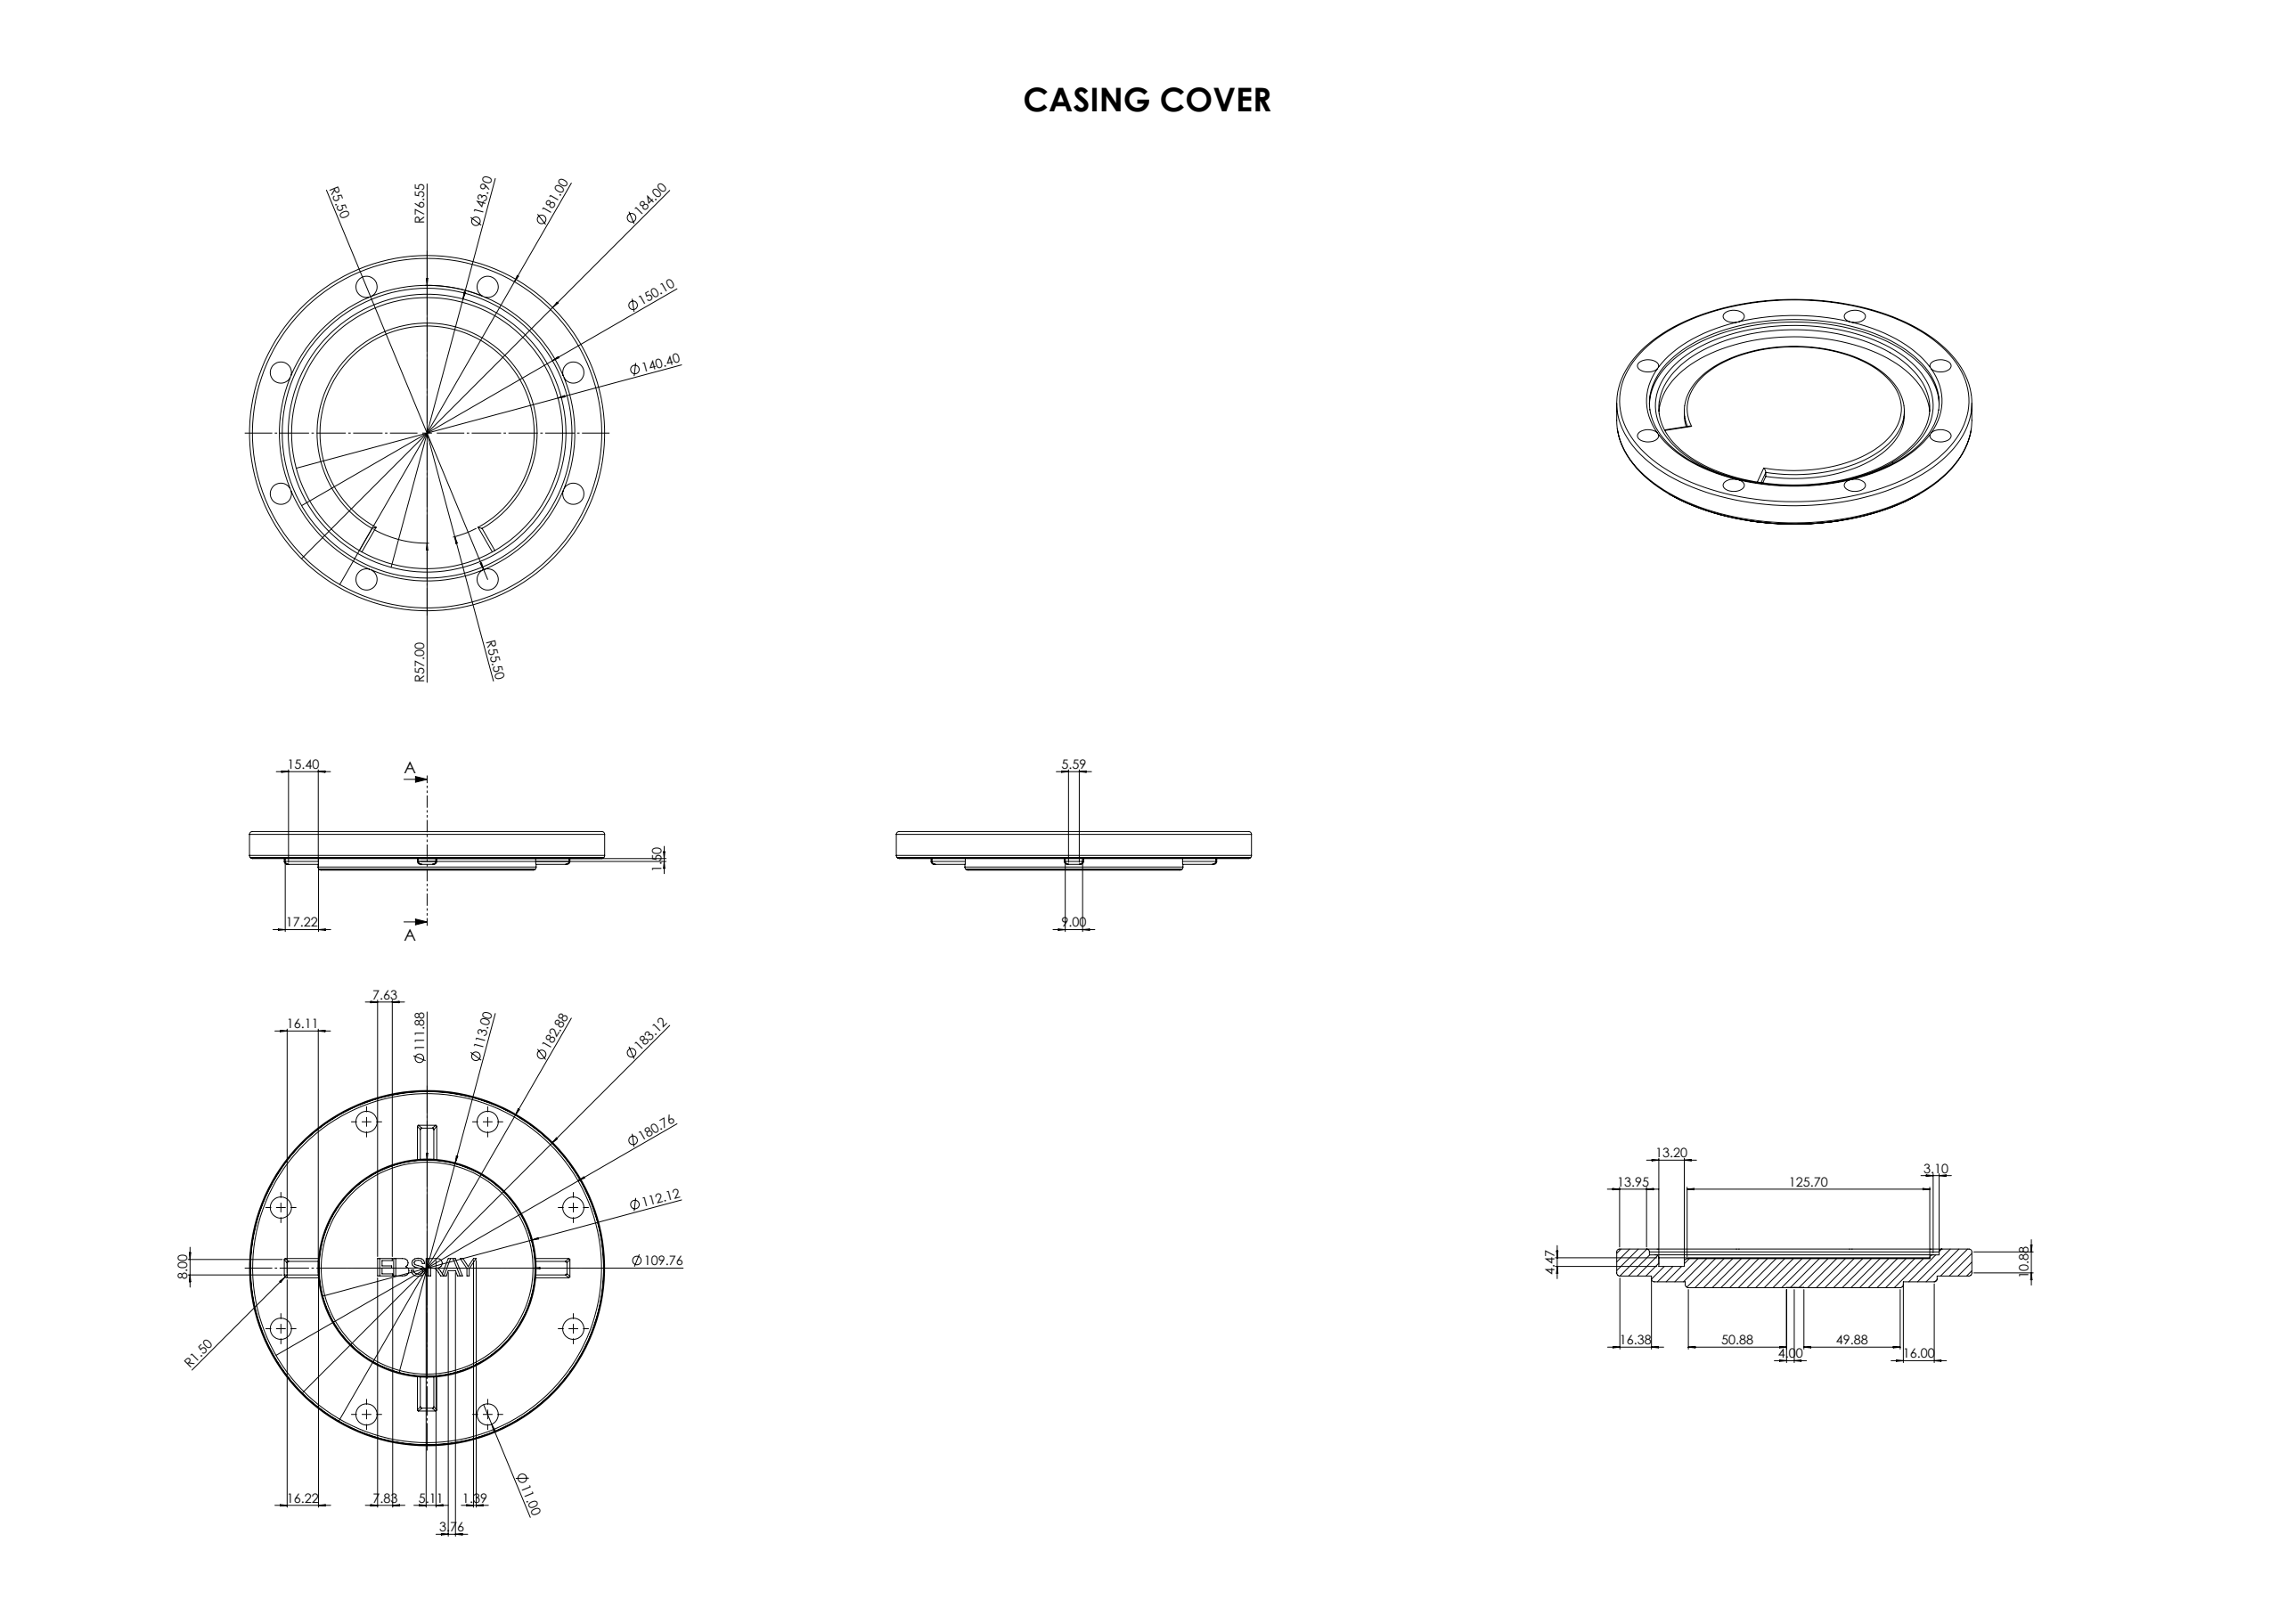
ISO-10303-21;
HEADER;
/* Generated by software containing ST-Developer
 * from STEP Tools, Inc. (www.steptools.com) 
 */

FILE_DESCRIPTION(
/* description */ (''),
/* implementation_level */ '2;1');

FILE_NAME(
/* name */ '02_Casing_Cover.step',
/* time_stamp */ '2026-10-26T04:15:57-07:00',
/* author */ (''),
/* organization */ (''),
/* preprocessor_version */ 'ST-DEVELOPER v20.2',
/* originating_system */ 'Autodesk Translation Framework v15.15.0.0',
/* authorisation */ '');

FILE_SCHEMA (('AUTOMOTIVE_DESIGN { 1 0 10303 214 3 1 1 }'));
ENDSEC;

DATA;
#10=MECHANICAL_DESIGN_GEOMETRIC_PRESENTATION_REPRESENTATION('',(#453),#55737);
#197=ELLIPSE('',#27930,1.60681112727484,1.5);
#198=ELLIPSE('',#27931,1.86380959388014,1.5);
#199=ELLIPSE('',#27932,1.60681112727484,1.5);
#200=ELLIPSE('',#27934,1.62076900489975,1.5);
#201=ELLIPSE('',#27935,1.62076900489975,1.5);
#338=SPHERICAL_SURFACE('',#27885,1.5);
#339=CONICAL_SURFACE('',#27821,91.5,0.785398163397447);
#340=CONICAL_SURFACE('',#27879,56.,0.785398163397451);
#413=SHAPE_REPRESENTATION_RELATIONSHIP('SRR','None',#55822,#433);
#433=ADVANCED_BREP_SHAPE_REPRESENTATION('',(#473),#55718);
#453=STYLED_ITEM('',(#55977),#473);
#473=MANIFOLD_SOLID_BREP('Body1',#27222);
#496=B_SPLINE_SURFACE_WITH_KNOTS('',3,3,((#38586,#38587,#38588,#38589,#38590,
#38591),(#38592,#38593,#38594,#38595,#38596,#38597),(#38598,#38599,#38600,
#38601,#38602,#38603),(#38604,#38605,#38606,#38607,#38608,#38609)),
 .UNSPECIFIED.,.F.,.F.,.F.,(4,4),(4,1,1,4),(0.,1.),(0.,0.571428571428571,
0.857142857142857,1.),.UNSPECIFIED.);
#497=B_SPLINE_SURFACE_WITH_KNOTS('',3,3,((#38729,#38730,#38731,#38732,#38733,
#38734),(#38735,#38736,#38737,#38738,#38739,#38740),(#38741,#38742,#38743,
#38744,#38745,#38746),(#38747,#38748,#38749,#38750,#38751,#38752)),
 .UNSPECIFIED.,.F.,.F.,.F.,(4,4),(4,1,1,4),(0.,1.),(-1.75610615531806,-1.00348923161032,
-0.501744615805159,2.22044604925036E-16),.UNSPECIFIED.);
#498=B_SPLINE_SURFACE_WITH_KNOTS('',3,3,((#38856,#38857,#38858,#38859,#38860,
#38861),(#38862,#38863,#38864,#38865,#38866,#38867),(#38868,#38869,#38870,
#38871,#38872,#38873),(#38874,#38875,#38876,#38877,#38878,#38879)),
 .UNSPECIFIED.,.F.,.F.,.F.,(4,4),(4,1,1,4),(0.,1.),(0.,0.571428571428571,
0.857142857142857,1.),.UNSPECIFIED.);
#499=B_SPLINE_SURFACE_WITH_KNOTS('',3,3,((#38940,#38941,#38942,#38943,#38944,
#38945,#38946),(#38947,#38948,#38949,#38950,#38951,#38952,#38953),(#38954,
#38955,#38956,#38957,#38958,#38959,#38960),(#38961,#38962,#38963,#38964,
#38965,#38966,#38967)),.UNSPECIFIED.,.F.,.F.,.F.,(4,4),(4,1,1,1,4),(0.,
1.),(-1.75610615531806,-1.2543615395129,-0.752616923707738,-0.501744615805159,
4.16333634234434E-16),.UNSPECIFIED.);
#500=B_SPLINE_SURFACE_WITH_KNOTS('',3,3,((#38998,#38999,#39000,#39001,#39002,
#39003),(#39004,#39005,#39006,#39007,#39008,#39009),(#39010,#39011,#39012,
#39013,#39014,#39015),(#39016,#39017,#39018,#39019,#39020,#39021)),
 .UNSPECIFIED.,.F.,.F.,.F.,(4,4),(4,1,1,4),(0.,1.),(0.,0.571428571428571,
0.857142857142857,1.),.UNSPECIFIED.);
#501=B_SPLINE_SURFACE_WITH_KNOTS('',3,3,((#39141,#39142,#39143,#39144,#39145,
#39146),(#39147,#39148,#39149,#39150,#39151,#39152),(#39153,#39154,#39155,
#39156,#39157,#39158),(#39159,#39160,#39161,#39162,#39163,#39164)),
 .UNSPECIFIED.,.F.,.F.,.F.,(4,4),(4,1,1,4),(0.,1.),(-1.75610615531806,-1.00348923161032,
-0.501744615805159,2.77555756156289E-17),.UNSPECIFIED.);
#502=B_SPLINE_SURFACE_WITH_KNOTS('',3,3,((#39202,#39203,#39204,#39205,#39206,
#39207),(#39208,#39209,#39210,#39211,#39212,#39213),(#39214,#39215,#39216,
#39217,#39218,#39219),(#39220,#39221,#39222,#39223,#39224,#39225)),
 .UNSPECIFIED.,.F.,.F.,.F.,(4,4),(4,1,1,4),(0.,1.),(0.,0.571428571428571,
0.857142857142857,1.),.UNSPECIFIED.);
#503=B_SPLINE_SURFACE_WITH_KNOTS('',3,3,((#39345,#39346,#39347,#39348,#39349,
#39350),(#39351,#39352,#39353,#39354,#39355,#39356),(#39357,#39358,#39359,
#39360,#39361,#39362),(#39363,#39364,#39365,#39366,#39367,#39368)),
 .UNSPECIFIED.,.F.,.F.,.F.,(4,4),(4,1,1,4),(0.,1.),(-1.75610615531806,-1.00348923161032,
-0.501744615805159,2.77555756156289E-17),.UNSPECIFIED.);
#504=B_SPLINE_SURFACE_WITH_KNOTS('',3,3,((#39469,#39470,#39471,#39472,#39473,
#39474),(#39475,#39476,#39477,#39478,#39479,#39480),(#39481,#39482,#39483,
#39484,#39485,#39486),(#39487,#39488,#39489,#39490,#39491,#39492)),
 .UNSPECIFIED.,.F.,.F.,.F.,(4,4),(4,1,1,4),(0.,1.),(0.,0.571428571428571,
0.857142857142857,1.),.UNSPECIFIED.);
#505=B_SPLINE_SURFACE_WITH_KNOTS('',3,3,((#39553,#39554,#39555,#39556,#39557,
#39558),(#39559,#39560,#39561,#39562,#39563,#39564),(#39565,#39566,#39567,
#39568,#39569,#39570),(#39571,#39572,#39573,#39574,#39575,#39576)),
 .UNSPECIFIED.,.F.,.F.,.F.,(4,4),(4,1,1,4),(0.,1.),(-1.75610615531806,-1.00348923161032,
-0.501744615805159,1.27116549159798E-31),.UNSPECIFIED.);
#506=B_SPLINE_SURFACE_WITH_KNOTS('',3,3,((#39606,#39607,#39608,#39609,#39610,
#39611),(#39612,#39613,#39614,#39615,#39616,#39617),(#39618,#39619,#39620,
#39621,#39622,#39623),(#39624,#39625,#39626,#39627,#39628,#39629)),
 .UNSPECIFIED.,.F.,.F.,.F.,(4,4),(4,1,1,4),(0.,1.),(0.,0.571428571428571,
0.857142857142857,1.),.UNSPECIFIED.);
#507=B_SPLINE_SURFACE_WITH_KNOTS('',3,3,((#39749,#39750,#39751,#39752,#39753,
#39754,#39755),(#39756,#39757,#39758,#39759,#39760,#39761,#39762),(#39763,
#39764,#39765,#39766,#39767,#39768,#39769),(#39770,#39771,#39772,#39773,
#39774,#39775,#39776)),.UNSPECIFIED.,.F.,.F.,.F.,(4,4),(4,1,1,1,4),(0.,
1.),(-1.75610615531805,-1.25436153951289,-0.752616923707736,-0.501744615805158,
1.11022302462516E-16),.UNSPECIFIED.);
#508=B_SPLINE_SURFACE_WITH_KNOTS('',3,3,((#39880,#39881,#39882,#39883,#39884,
#39885),(#39886,#39887,#39888,#39889,#39890,#39891),(#39892,#39893,#39894,
#39895,#39896,#39897),(#39898,#39899,#39900,#39901,#39902,#39903)),
 .UNSPECIFIED.,.F.,.F.,.F.,(4,4),(4,1,1,4),(0.,1.),(0.,0.571428571428571,
0.857142857142857,1.),.UNSPECIFIED.);
#509=B_SPLINE_SURFACE_WITH_KNOTS('',3,3,((#39964,#39965,#39966,#39967,#39968,
#39969,#39970),(#39971,#39972,#39973,#39974,#39975,#39976,#39977),(#39978,
#39979,#39980,#39981,#39982,#39983,#39984),(#39985,#39986,#39987,#39988,
#39989,#39990,#39991)),.UNSPECIFIED.,.F.,.F.,.F.,(4,4),(4,1,1,1,4),(0.,
1.),(-1.75610615531806,-1.2543615395129,-0.752616923707739,-0.501744615805159,
4.10679309198325E-32),.UNSPECIFIED.);
#510=B_SPLINE_SURFACE_WITH_KNOTS('',2,1,((#40770,#40771),(#40772,#40773),
(#40774,#40775)),.UNSPECIFIED.,.F.,.F.,.F.,(3,3),(2,2),(0.,1.),(0.,0.05),
 .UNSPECIFIED.);
#511=B_SPLINE_SURFACE_WITH_KNOTS('',2,1,((#40783,#40784),(#40785,#40786),
(#40787,#40788)),.UNSPECIFIED.,.F.,.F.,.F.,(3,3),(2,2),(0.,1.),(0.,0.05),
 .UNSPECIFIED.);
#512=B_SPLINE_SURFACE_WITH_KNOTS('',2,1,((#40794,#40795),(#40796,#40797),
(#40798,#40799)),.UNSPECIFIED.,.F.,.F.,.F.,(3,3),(2,2),(0.,1.),(0.,0.05),
 .UNSPECIFIED.);
#513=B_SPLINE_SURFACE_WITH_KNOTS('',2,1,((#40805,#40806),(#40807,#40808),
(#40809,#40810)),.UNSPECIFIED.,.F.,.F.,.F.,(3,3),(2,2),(0.,1.),(0.,0.05),
 .UNSPECIFIED.);
#514=B_SPLINE_SURFACE_WITH_KNOTS('',2,1,((#40816,#40817),(#40818,#40819),
(#40820,#40821)),.UNSPECIFIED.,.F.,.F.,.F.,(3,3),(2,2),(0.,1.),(0.,0.05),
 .UNSPECIFIED.);
#515=B_SPLINE_SURFACE_WITH_KNOTS('',2,1,((#40827,#40828),(#40829,#40830),
(#40831,#40832)),.UNSPECIFIED.,.F.,.F.,.F.,(3,3),(2,2),(0.,1.),(0.,0.05),
 .UNSPECIFIED.);
#516=B_SPLINE_SURFACE_WITH_KNOTS('',2,1,((#40838,#40839),(#40840,#40841),
(#40842,#40843)),.UNSPECIFIED.,.F.,.F.,.F.,(3,3),(2,2),(0.,1.),(0.,0.05),
 .UNSPECIFIED.);
#517=B_SPLINE_SURFACE_WITH_KNOTS('',2,1,((#40849,#40850),(#40851,#40852),
(#40853,#40854)),.UNSPECIFIED.,.F.,.F.,.F.,(3,3),(2,2),(0.,1.),(0.,0.05),
 .UNSPECIFIED.);
#518=B_SPLINE_SURFACE_WITH_KNOTS('',2,1,((#40860,#40861),(#40862,#40863),
(#40864,#40865)),.UNSPECIFIED.,.F.,.F.,.F.,(3,3),(2,2),(0.,1.),(0.,0.05),
 .UNSPECIFIED.);
#519=B_SPLINE_SURFACE_WITH_KNOTS('',2,1,((#40871,#40872),(#40873,#40874),
(#40875,#40876)),.UNSPECIFIED.,.F.,.F.,.F.,(3,3),(2,2),(0.,1.),(0.,0.05),
 .UNSPECIFIED.);
#520=B_SPLINE_SURFACE_WITH_KNOTS('',2,1,((#40888,#40889),(#40890,#40891),
(#40892,#40893)),.UNSPECIFIED.,.F.,.F.,.F.,(3,3),(2,2),(0.,1.),(0.,0.05),
 .UNSPECIFIED.);
#521=B_SPLINE_SURFACE_WITH_KNOTS('',2,1,((#40898,#40899),(#40900,#40901),
(#40902,#40903)),.UNSPECIFIED.,.F.,.F.,.F.,(3,3),(2,2),(0.,1.),(0.,0.05),
 .UNSPECIFIED.);
#522=B_SPLINE_SURFACE_WITH_KNOTS('',2,1,((#40911,#40912),(#40913,#40914),
(#40915,#40916)),.UNSPECIFIED.,.F.,.F.,.F.,(3,3),(2,2),(0.,1.),(0.,0.05),
 .UNSPECIFIED.);
#523=B_SPLINE_SURFACE_WITH_KNOTS('',2,1,((#40922,#40923),(#40924,#40925),
(#40926,#40927)),.UNSPECIFIED.,.F.,.F.,.F.,(3,3),(2,2),(0.,1.),(0.,0.05),
 .UNSPECIFIED.);
#524=B_SPLINE_SURFACE_WITH_KNOTS('',2,1,((#40933,#40934),(#40935,#40936),
(#40937,#40938)),.UNSPECIFIED.,.F.,.F.,.F.,(3,3),(2,2),(0.,1.),(0.,0.05),
 .UNSPECIFIED.);
#525=B_SPLINE_SURFACE_WITH_KNOTS('',2,1,((#40944,#40945),(#40946,#40947),
(#40948,#40949)),.UNSPECIFIED.,.F.,.F.,.F.,(3,3),(2,2),(0.,1.),(0.,0.05),
 .UNSPECIFIED.);
#526=B_SPLINE_SURFACE_WITH_KNOTS('',2,1,((#40955,#40956),(#40957,#40958),
(#40959,#40960)),.UNSPECIFIED.,.F.,.F.,.F.,(3,3),(2,2),(0.,1.),(0.,0.05),
 .UNSPECIFIED.);
#527=B_SPLINE_SURFACE_WITH_KNOTS('',2,1,((#40966,#40967),(#40968,#40969),
(#40970,#40971)),.UNSPECIFIED.,.F.,.F.,.F.,(3,3),(2,2),(0.,1.),(0.,0.05),
 .UNSPECIFIED.);
#528=B_SPLINE_SURFACE_WITH_KNOTS('',2,1,((#40977,#40978),(#40979,#40980),
(#40981,#40982)),.UNSPECIFIED.,.F.,.F.,.F.,(3,3),(2,2),(0.,1.),(0.,0.05),
 .UNSPECIFIED.);
#529=B_SPLINE_SURFACE_WITH_KNOTS('',2,1,((#40988,#40989),(#40990,#40991),
(#40992,#40993)),.UNSPECIFIED.,.F.,.F.,.F.,(3,3),(2,2),(0.,1.),(0.,0.05),
 .UNSPECIFIED.);
#530=B_SPLINE_SURFACE_WITH_KNOTS('',2,1,((#40999,#41000),(#41001,#41002),
(#41003,#41004)),.UNSPECIFIED.,.F.,.F.,.F.,(3,3),(2,2),(0.,1.),(0.,0.05),
 .UNSPECIFIED.);
#531=B_SPLINE_SURFACE_WITH_KNOTS('',2,1,((#41010,#41011),(#41012,#41013),
(#41014,#41015)),.UNSPECIFIED.,.F.,.F.,.F.,(3,3),(2,2),(0.,1.),(0.,0.05),
 .UNSPECIFIED.);
#532=B_SPLINE_SURFACE_WITH_KNOTS('',2,1,((#41021,#41022),(#41023,#41024),
(#41025,#41026)),.UNSPECIFIED.,.F.,.F.,.F.,(3,3),(2,2),(0.,1.),(0.,0.05),
 .UNSPECIFIED.);
#533=B_SPLINE_SURFACE_WITH_KNOTS('',2,1,((#41032,#41033),(#41034,#41035),
(#41036,#41037)),.UNSPECIFIED.,.F.,.F.,.F.,(3,3),(2,2),(0.,1.),(0.,0.05),
 .UNSPECIFIED.);
#534=B_SPLINE_SURFACE_WITH_KNOTS('',2,1,((#41047,#41048),(#41049,#41050),
(#41051,#41052)),.UNSPECIFIED.,.F.,.F.,.F.,(3,3),(2,2),(0.,1.),(0.,0.05),
 .UNSPECIFIED.);
#535=B_SPLINE_SURFACE_WITH_KNOTS('',2,1,((#41058,#41059),(#41060,#41061),
(#41062,#41063)),.UNSPECIFIED.,.F.,.F.,.F.,(3,3),(2,2),(0.,1.),(0.,0.05),
 .UNSPECIFIED.);
#536=B_SPLINE_SURFACE_WITH_KNOTS('',2,1,((#41069,#41070),(#41071,#41072),
(#41073,#41074)),.UNSPECIFIED.,.F.,.F.,.F.,(3,3),(2,2),(0.,1.),(0.,0.05),
 .UNSPECIFIED.);
#537=B_SPLINE_SURFACE_WITH_KNOTS('',2,1,((#41080,#41081),(#41082,#41083),
(#41084,#41085)),.UNSPECIFIED.,.F.,.F.,.F.,(3,3),(2,2),(0.,1.),(0.,0.05),
 .UNSPECIFIED.);
#538=B_SPLINE_SURFACE_WITH_KNOTS('',2,1,((#41091,#41092),(#41093,#41094),
(#41095,#41096)),.UNSPECIFIED.,.F.,.F.,.F.,(3,3),(2,2),(0.,1.),(0.,0.05),
 .UNSPECIFIED.);
#539=B_SPLINE_SURFACE_WITH_KNOTS('',2,1,((#41102,#41103),(#41104,#41105),
(#41106,#41107)),.UNSPECIFIED.,.F.,.F.,.F.,(3,3),(2,2),(0.,1.),(0.,0.05),
 .UNSPECIFIED.);
#540=B_SPLINE_SURFACE_WITH_KNOTS('',2,1,((#41113,#41114),(#41115,#41116),
(#41117,#41118)),.UNSPECIFIED.,.F.,.F.,.F.,(3,3),(2,2),(0.,1.),(0.,0.05),
 .UNSPECIFIED.);
#541=B_SPLINE_SURFACE_WITH_KNOTS('',2,1,((#41124,#41125),(#41126,#41127),
(#41128,#41129)),.UNSPECIFIED.,.F.,.F.,.F.,(3,3),(2,2),(0.,1.),(0.,0.05),
 .UNSPECIFIED.);
#542=B_SPLINE_SURFACE_WITH_KNOTS('',2,1,((#41135,#41136),(#41137,#41138),
(#41139,#41140)),.UNSPECIFIED.,.F.,.F.,.F.,(3,3),(2,2),(0.,1.),(0.,0.05),
 .UNSPECIFIED.);
#543=B_SPLINE_SURFACE_WITH_KNOTS('',2,1,((#41146,#41147),(#41148,#41149),
(#41150,#41151)),.UNSPECIFIED.,.F.,.F.,.F.,(3,3),(2,2),(0.,1.),(0.,0.05),
 .UNSPECIFIED.);
#544=B_SPLINE_SURFACE_WITH_KNOTS('',2,1,((#41157,#41158),(#41159,#41160),
(#41161,#41162)),.UNSPECIFIED.,.F.,.F.,.F.,(3,3),(2,2),(0.,1.),(0.,0.05),
 .UNSPECIFIED.);
#545=B_SPLINE_SURFACE_WITH_KNOTS('',2,1,((#41168,#41169),(#41170,#41171),
(#41172,#41173)),.UNSPECIFIED.,.F.,.F.,.F.,(3,3),(2,2),(0.,1.),(0.,0.05),
 .UNSPECIFIED.);
#546=B_SPLINE_SURFACE_WITH_KNOTS('',2,1,((#41179,#41180),(#41181,#41182),
(#41183,#41184)),.UNSPECIFIED.,.F.,.F.,.F.,(3,3),(2,2),(0.,1.),(0.,0.05),
 .UNSPECIFIED.);
#547=B_SPLINE_SURFACE_WITH_KNOTS('',2,1,((#41190,#41191),(#41192,#41193),
(#41194,#41195)),.UNSPECIFIED.,.F.,.F.,.F.,(3,3),(2,2),(0.,1.),(0.,0.05),
 .UNSPECIFIED.);
#548=B_SPLINE_SURFACE_WITH_KNOTS('',2,1,((#41201,#41202),(#41203,#41204),
(#41205,#41206)),.UNSPECIFIED.,.F.,.F.,.F.,(3,3),(2,2),(0.,1.),(0.,0.05),
 .UNSPECIFIED.);
#549=B_SPLINE_SURFACE_WITH_KNOTS('',2,1,((#41212,#41213),(#41214,#41215),
(#41216,#41217)),.UNSPECIFIED.,.F.,.F.,.F.,(3,3),(2,2),(0.,1.),(0.,0.05),
 .UNSPECIFIED.);
#550=B_SPLINE_SURFACE_WITH_KNOTS('',2,1,((#41223,#41224),(#41225,#41226),
(#41227,#41228)),.UNSPECIFIED.,.F.,.F.,.F.,(3,3),(2,2),(0.,1.),(0.,0.05),
 .UNSPECIFIED.);
#551=B_SPLINE_SURFACE_WITH_KNOTS('',2,1,((#41234,#41235),(#41236,#41237),
(#41238,#41239)),.UNSPECIFIED.,.F.,.F.,.F.,(3,3),(2,2),(0.,1.),(0.,0.05),
 .UNSPECIFIED.);
#552=B_SPLINE_SURFACE_WITH_KNOTS('',2,1,((#41249,#41250),(#41251,#41252),
(#41253,#41254)),.UNSPECIFIED.,.F.,.F.,.F.,(3,3),(2,2),(0.,1.),(0.,0.05),
 .UNSPECIFIED.);
#553=B_SPLINE_SURFACE_WITH_KNOTS('',2,1,((#41260,#41261),(#41262,#41263),
(#41264,#41265)),.UNSPECIFIED.,.F.,.F.,.F.,(3,3),(2,2),(0.,1.),(0.,0.05),
 .UNSPECIFIED.);
#554=B_SPLINE_SURFACE_WITH_KNOTS('',2,1,((#41276,#41277),(#41278,#41279),
(#41280,#41281)),.UNSPECIFIED.,.F.,.F.,.F.,(3,3),(2,2),(0.,1.),(0.,0.05),
 .UNSPECIFIED.);
#555=B_SPLINE_SURFACE_WITH_KNOTS('',2,1,((#41287,#41288),(#41289,#41290),
(#41291,#41292)),.UNSPECIFIED.,.F.,.F.,.F.,(3,3),(2,2),(0.,1.),(0.,0.05),
 .UNSPECIFIED.);
#556=B_SPLINE_SURFACE_WITH_KNOTS('',2,1,((#41298,#41299),(#41300,#41301),
(#41302,#41303)),.UNSPECIFIED.,.F.,.F.,.F.,(3,3),(2,2),(0.,1.),(0.,0.05),
 .UNSPECIFIED.);
#557=B_SPLINE_SURFACE_WITH_KNOTS('',2,1,((#41309,#41310),(#41311,#41312),
(#41313,#41314)),.UNSPECIFIED.,.F.,.F.,.F.,(3,3),(2,2),(0.,1.),(0.,0.05),
 .UNSPECIFIED.);
#558=B_SPLINE_SURFACE_WITH_KNOTS('',2,1,((#41326,#41327),(#41328,#41329),
(#41330,#41331)),.UNSPECIFIED.,.F.,.F.,.F.,(3,3),(2,2),(0.,1.),(0.,0.05),
 .UNSPECIFIED.);
#559=B_SPLINE_SURFACE_WITH_KNOTS('',2,1,((#41337,#41338),(#41339,#41340),
(#41341,#41342)),.UNSPECIFIED.,.F.,.F.,.F.,(3,3),(2,2),(0.,1.),(0.,0.05),
 .UNSPECIFIED.);
#560=B_SPLINE_SURFACE_WITH_KNOTS('',2,1,((#41348,#41349),(#41350,#41351),
(#41352,#41353)),.UNSPECIFIED.,.F.,.F.,.F.,(3,3),(2,2),(0.,1.),(0.,0.05),
 .UNSPECIFIED.);
#561=B_SPLINE_SURFACE_WITH_KNOTS('',2,1,((#41359,#41360),(#41361,#41362),
(#41363,#41364)),.UNSPECIFIED.,.F.,.F.,.F.,(3,3),(2,2),(0.,1.),(0.,0.05),
 .UNSPECIFIED.);
#562=B_SPLINE_SURFACE_WITH_KNOTS('',2,1,((#41370,#41371),(#41372,#41373),
(#41374,#41375)),.UNSPECIFIED.,.F.,.F.,.F.,(3,3),(2,2),(0.,1.),(0.,0.05),
 .UNSPECIFIED.);
#563=B_SPLINE_SURFACE_WITH_KNOTS('',2,1,((#41381,#41382),(#41383,#41384),
(#41385,#41386)),.UNSPECIFIED.,.F.,.F.,.F.,(3,3),(2,2),(0.,1.),(0.,0.05),
 .UNSPECIFIED.);
#564=B_SPLINE_SURFACE_WITH_KNOTS('',2,1,((#41392,#41393),(#41394,#41395),
(#41396,#41397)),.UNSPECIFIED.,.F.,.F.,.F.,(3,3),(2,2),(0.,1.),(0.,0.05),
 .UNSPECIFIED.);
#565=B_SPLINE_SURFACE_WITH_KNOTS('',2,1,((#41426,#41427),(#41428,#41429),
(#41430,#41431)),.UNSPECIFIED.,.F.,.F.,.F.,(3,3),(2,2),(0.,1.),(0.,0.05),
 .UNSPECIFIED.);
#566=B_SPLINE_SURFACE_WITH_KNOTS('',2,1,((#41437,#41438),(#41439,#41440),
(#41441,#41442)),.UNSPECIFIED.,.F.,.F.,.F.,(3,3),(2,2),(0.,1.),(0.,0.05),
 .UNSPECIFIED.);
#631=FACE_BOUND('',#8624,.T.);
#632=FACE_BOUND('',#8625,.T.);
#633=FACE_BOUND('',#8626,.T.);
#634=FACE_BOUND('',#8627,.T.);
#635=FACE_BOUND('',#8628,.T.);
#636=FACE_BOUND('',#8629,.T.);
#637=FACE_BOUND('',#8630,.T.);
#638=FACE_BOUND('',#8631,.T.);
#639=FACE_BOUND('',#8632,.T.);
#640=FACE_BOUND('',#8639,.T.);
#641=FACE_BOUND('',#8643,.T.);
#642=FACE_BOUND('',#8644,.T.);
#643=FACE_BOUND('',#8645,.T.);
#644=FACE_BOUND('',#8646,.T.);
#645=FACE_BOUND('',#8647,.T.);
#646=FACE_BOUND('',#8778,.T.);
#810=PLANE('',#27786);
#811=PLANE('',#27787);
#812=PLANE('',#27791);
#813=PLANE('',#27792);
#814=PLANE('',#27794);
#815=PLANE('',#27795);
#816=PLANE('',#27796);
#817=PLANE('',#27800);
#818=PLANE('',#27801);
#819=PLANE('',#27802);
#820=PLANE('',#27805);
#821=PLANE('',#27806);
#822=PLANE('',#27808);
#823=PLANE('',#27809);
#824=PLANE('',#27810);
#825=PLANE('',#27813);
#826=PLANE('',#27814);
#827=PLANE('',#27816);
#828=PLANE('',#27828);
#829=PLANE('',#27843);
#830=PLANE('',#27845);
#831=PLANE('',#27849);
#832=PLANE('',#27881);
#833=PLANE('',#27888);
#834=PLANE('',#27894);
#835=PLANE('',#27900);
#836=PLANE('',#27936);
#837=PLANE('',#27937);
#838=PLANE('',#27938);
#839=PLANE('',#27939);
#840=PLANE('',#27940);
#841=PLANE('',#27941);
#842=PLANE('',#27942);
#843=PLANE('',#27943);
#844=PLANE('',#27944);
#845=PLANE('',#27945);
#846=PLANE('',#27946);
#847=PLANE('',#27947);
#848=PLANE('',#27948);
#849=PLANE('',#27949);
#850=PLANE('',#27950);
#851=PLANE('',#27951);
#852=PLANE('',#27952);
#853=PLANE('',#27953);
#854=PLANE('',#27954);
#855=PLANE('',#27955);
#856=PLANE('',#27956);
#857=PLANE('',#27957);
#858=PLANE('',#27958);
#859=PLANE('',#27959);
#860=PLANE('',#27960);
#861=PLANE('',#27961);
#862=PLANE('',#27962);
#863=PLANE('',#27963);
#864=PLANE('',#27964);
#865=PLANE('',#27965);
#866=PLANE('',#27966);
#867=PLANE('',#27967);
#868=PLANE('',#27968);
#869=PLANE('',#27969);
#870=PLANE('',#27970);
#871=PLANE('',#27971);
#872=PLANE('',#27972);
#873=PLANE('',#27973);
#874=PLANE('',#27974);
#875=PLANE('',#27975);
#876=PLANE('',#27976);
#877=PLANE('',#27977);
#878=PLANE('',#27982);
#879=PLANE('',#27985);
#880=PLANE('',#27986);
#881=PLANE('',#27987);
#882=PLANE('',#27988);
#1899=LINE('',#38728,#4270);
#1900=LINE('',#38761,#4271);
#1901=LINE('',#38771,#4272);
#1902=LINE('',#38772,#4273);
#1903=LINE('',#38773,#4274);
#1904=LINE('',#38776,#4275);
#1905=LINE('',#38778,#4276);
#1906=LINE('',#38780,#4277);
#1907=LINE('',#38785,#4278);
#1908=LINE('',#38788,#4279);
#1909=LINE('',#38854,#4280);
#1910=LINE('',#38855,#4281);
#1911=LINE('',#38969,#4282);
#1912=LINE('',#38979,#4283);
#1913=LINE('',#38980,#4284);
#1914=LINE('',#38983,#4285);
#1915=LINE('',#38996,#4286);
#1916=LINE('',#38997,#4287);
#1917=LINE('',#39140,#4288);
#1918=LINE('',#39173,#4289);
#1919=LINE('',#39183,#4290);
#1920=LINE('',#39184,#4291);
#1921=LINE('',#39185,#4292);
#1922=LINE('',#39188,#4293);
#1923=LINE('',#39190,#4294);
#1924=LINE('',#39193,#4295);
#1925=LINE('',#39196,#4296);
#1926=LINE('',#39200,#4297);
#1927=LINE('',#39201,#4298);
#1928=LINE('',#39344,#4299);
#1929=LINE('',#39377,#4300);
#1930=LINE('',#39387,#4301);
#1931=LINE('',#39388,#4302);
#1932=LINE('',#39389,#4303);
#1933=LINE('',#39392,#4304);
#1934=LINE('',#39394,#4305);
#1935=LINE('',#39396,#4306);
#1936=LINE('',#39399,#4307);
#1937=LINE('',#39402,#4308);
#1938=LINE('',#39467,#4309);
#1939=LINE('',#39468,#4310);
#1940=LINE('',#39578,#4311);
#1941=LINE('',#39587,#4312);
#1942=LINE('',#39588,#4313);
#1943=LINE('',#39591,#4314);
#1944=LINE('',#39604,#4315);
#1945=LINE('',#39605,#4316);
#1946=LINE('',#39748,#4317);
#1947=LINE('',#39786,#4318);
#1948=LINE('',#39797,#4319);
#1949=LINE('',#39798,#4320);
#1950=LINE('',#39799,#4321);
#1951=LINE('',#39802,#4322);
#1952=LINE('',#39804,#4323);
#1953=LINE('',#39806,#4324);
#1954=LINE('',#39809,#4325);
#1955=LINE('',#39812,#4326);
#1956=LINE('',#39878,#4327);
#1957=LINE('',#39879,#4328);
#1958=LINE('',#39993,#4329);
#1959=LINE('',#40003,#4330);
#1960=LINE('',#40004,#4331);
#1961=LINE('',#40007,#4332);
#1962=LINE('',#40020,#4333);
#1963=LINE('',#40021,#4334);
#1964=LINE('',#40030,#4335);
#1965=LINE('',#40035,#4336);
#1966=LINE('',#40058,#4337);
#1967=LINE('',#40062,#4338);
#1968=LINE('',#40065,#4339);
#1969=LINE('',#40068,#4340);
#1970=LINE('',#40071,#4341);
#1971=LINE('',#40085,#4342);
#1972=LINE('',#40087,#4343);
#1973=LINE('',#40100,#4344);
#1974=LINE('',#40102,#4345);
#1975=LINE('',#40167,#4346);
#1976=LINE('',#40183,#4347);
#1977=LINE('',#40257,#4348);
#1978=LINE('',#40307,#4349);
#1979=LINE('',#40309,#4350);
#1980=LINE('',#40311,#4351);
#1981=LINE('',#40313,#4352);
#1982=LINE('',#40315,#4353);
#1983=LINE('',#40317,#4354);
#1984=LINE('',#40319,#4355);
#1985=LINE('',#40329,#4356);
#1986=LINE('',#40330,#4357);
#1987=LINE('',#40333,#4358);
#1988=LINE('',#40335,#4359);
#1989=LINE('',#40337,#4360);
#1990=LINE('',#40339,#4361);
#1991=LINE('',#40341,#4362);
#1992=LINE('',#40343,#4363);
#1993=LINE('',#40345,#4364);
#1994=LINE('',#40347,#4365);
#1995=LINE('',#40349,#4366);
#1996=LINE('',#40351,#4367);
#1997=LINE('',#40353,#4368);
#1998=LINE('',#40354,#4369);
#1999=LINE('',#40357,#4370);
#2000=LINE('',#40403,#4371);
#2001=LINE('',#40404,#4372);
#2002=LINE('',#40407,#4373);
#2003=LINE('',#40437,#4374);
#2004=LINE('',#40439,#4375);
#2005=LINE('',#40441,#4376);
#2006=LINE('',#40443,#4377);
#2007=LINE('',#40445,#4378);
#2008=LINE('',#40447,#4379);
#2009=LINE('',#40449,#4380);
#2010=LINE('',#40451,#4381);
#2011=LINE('',#40453,#4382);
#2012=LINE('',#40455,#4383);
#2013=LINE('',#40473,#4384);
#2014=LINE('',#40475,#4385);
#2015=LINE('',#40477,#4386);
#2016=LINE('',#40478,#4387);
#2017=LINE('',#40491,#4388);
#2018=LINE('',#40495,#4389);
#2019=LINE('',#40500,#4390);
#2020=LINE('',#40512,#4391);
#2021=LINE('',#40519,#4392);
#2022=LINE('',#40530,#4393);
#2023=LINE('',#40531,#4394);
#2024=LINE('',#40533,#4395);
#2025=LINE('',#40572,#4396);
#2026=LINE('',#40584,#4397);
#2027=LINE('',#40587,#4398);
#2028=LINE('',#40599,#4399);
#2029=LINE('',#40612,#4400);
#2030=LINE('',#40615,#4401);
#2031=LINE('',#40618,#4402);
#2032=LINE('',#40658,#4403);
#2033=LINE('',#40660,#4404);
#2034=LINE('',#40662,#4405);
#2035=LINE('',#40664,#4406);
#2036=LINE('',#40668,#4407);
#2037=LINE('',#40674,#4408);
#2038=LINE('',#40680,#4409);
#2039=LINE('',#40686,#4410);
#2040=LINE('',#40694,#4411);
#2041=LINE('',#40700,#4412);
#2042=LINE('',#40703,#4413);
#2043=LINE('',#40705,#4414);
#2044=LINE('',#40706,#4415);
#2045=LINE('',#40709,#4416);
#2046=LINE('',#40710,#4417);
#2047=LINE('',#40712,#4418);
#2048=LINE('',#40714,#4419);
#2049=LINE('',#40717,#4420);
#2050=LINE('',#40718,#4421);
#2051=LINE('',#40720,#4422);
#2052=LINE('',#40722,#4423);
#2053=LINE('',#40723,#4424);
#2054=LINE('',#40725,#4425);
#2055=LINE('',#40729,#4426);
#2056=LINE('',#40731,#4427);
#2057=LINE('',#40732,#4428);
#2058=LINE('',#40735,#4429);
#2059=LINE('',#40736,#4430);
#2060=LINE('',#40739,#4431);
#2061=LINE('',#40740,#4432);
#2062=LINE('',#40743,#4433);
#2063=LINE('',#40744,#4434);
#2064=LINE('',#40747,#4435);
#2065=LINE('',#40748,#4436);
#2066=LINE('',#40751,#4437);
#2067=LINE('',#40752,#4438);
#2068=LINE('',#40755,#4439);
#2069=LINE('',#40756,#4440);
#2070=LINE('',#40759,#4441);
#2071=LINE('',#40760,#4442);
#2072=LINE('',#40762,#4443);
#2073=LINE('',#40765,#4444);
#2074=LINE('',#40766,#4445);
#2075=LINE('',#40768,#4446);
#2076=LINE('',#40777,#4447);
#2077=LINE('',#40782,#4448);
#2078=LINE('',#40790,#4449);
#2079=LINE('',#40801,#4450);
#2080=LINE('',#40812,#4451);
#2081=LINE('',#40823,#4452);
#2082=LINE('',#40834,#4453);
#2083=LINE('',#40845,#4454);
#2084=LINE('',#40856,#4455);
#2085=LINE('',#40867,#4456);
#2086=LINE('',#40878,#4457);
#2087=LINE('',#40883,#4458);
#2088=LINE('',#40886,#4459);
#2089=LINE('',#40887,#4460);
#2090=LINE('',#40905,#4461);
#2091=LINE('',#40910,#4462);
#2092=LINE('',#40918,#4463);
#2093=LINE('',#40929,#4464);
#2094=LINE('',#40940,#4465);
#2095=LINE('',#40951,#4466);
#2096=LINE('',#40962,#4467);
#2097=LINE('',#40973,#4468);
#2098=LINE('',#40984,#4469);
#2099=LINE('',#40995,#4470);
#2100=LINE('',#41006,#4471);
#2101=LINE('',#41017,#4472);
#2102=LINE('',#41028,#4473);
#2103=LINE('',#41039,#4474);
#2104=LINE('',#41045,#4475);
#2105=LINE('',#41046,#4476);
#2106=LINE('',#41054,#4477);
#2107=LINE('',#41065,#4478);
#2108=LINE('',#41076,#4479);
#2109=LINE('',#41087,#4480);
#2110=LINE('',#41098,#4481);
#2111=LINE('',#41109,#4482);
#2112=LINE('',#41120,#4483);
#2113=LINE('',#41131,#4484);
#2114=LINE('',#41142,#4485);
#2115=LINE('',#41153,#4486);
#2116=LINE('',#41164,#4487);
#2117=LINE('',#41175,#4488);
#2118=LINE('',#41186,#4489);
#2119=LINE('',#41197,#4490);
#2120=LINE('',#41208,#4491);
#2121=LINE('',#41219,#4492);
#2122=LINE('',#41230,#4493);
#2123=LINE('',#41241,#4494);
#2124=LINE('',#41247,#4495);
#2125=LINE('',#41248,#4496);
#2126=LINE('',#41256,#4497);
#2127=LINE('',#41272,#4498);
#2128=LINE('',#41274,#4499);
#2129=LINE('',#41275,#4500);
#2130=LINE('',#41283,#4501);
#2131=LINE('',#41294,#4502);
#2132=LINE('',#41305,#4503);
#2133=LINE('',#41316,#4504);
#2134=LINE('',#41321,#4505);
#2135=LINE('',#41324,#4506);
#2136=LINE('',#41325,#4507);
#2137=LINE('',#41333,#4508);
#2138=LINE('',#41344,#4509);
#2139=LINE('',#41355,#4510);
#2140=LINE('',#41366,#4511);
#2141=LINE('',#41377,#4512);
#2142=LINE('',#41388,#4513);
#2143=LINE('',#41399,#4514);
#2144=LINE('',#41404,#4515);
#2145=LINE('',#41407,#4516);
#2146=LINE('',#41408,#4517);
#2147=LINE('',#41410,#4518);
#2148=LINE('',#41414,#4519);
#2149=LINE('',#41416,#4520);
#2150=LINE('',#41417,#4521);
#2151=LINE('',#41420,#4522);
#2152=LINE('',#41421,#4523);
#2153=LINE('',#41424,#4524);
#2154=LINE('',#41425,#4525);
#2155=LINE('',#41433,#4526);
#2156=LINE('',#41444,#4527);
#2157=LINE('',#41450,#4528);
#2158=LINE('',#41451,#4529);
#2159=LINE('',#41454,#4530);
#2160=LINE('',#41455,#4531);
#2161=LINE('',#41458,#4532);
#2162=LINE('',#41459,#4533);
#2163=LINE('',#41462,#4534);
#2164=LINE('',#41463,#4535);
#2165=LINE('',#41466,#4536);
#2166=LINE('',#41467,#4537);
#2167=LINE('',#41469,#4538);
#2168=LINE('',#41472,#4539);
#2169=LINE('',#41474,#4540);
#2170=LINE('',#41476,#4541);
#2171=LINE('',#41478,#4542);
#2172=LINE('',#41482,#4543);
#2173=LINE('',#41485,#4544);
#2174=LINE('',#41487,#4545);
#2175=LINE('',#41489,#4546);
#4270=VECTOR('',#30765,10.);
#4271=VECTOR('',#30766,10.);
#4272=VECTOR('',#30769,10.);
#4273=VECTOR('',#30770,10.);
#4274=VECTOR('',#30771,10.);
#4275=VECTOR('',#30774,10.);
#4276=VECTOR('',#30775,10.);
#4277=VECTOR('',#30776,10.);
#4278=VECTOR('',#30781,10.);
#4279=VECTOR('',#30784,10.);
#4280=VECTOR('',#30787,10.);
#4281=VECTOR('',#30788,10.);
#4282=VECTOR('',#30789,10.);
#4283=VECTOR('',#30792,10.);
#4284=VECTOR('',#30793,10.);
#4285=VECTOR('',#30796,10.);
#4286=VECTOR('',#30799,10.);
#4287=VECTOR('',#30800,10.);
#4288=VECTOR('',#30801,10.);
#4289=VECTOR('',#30802,10.);
#4290=VECTOR('',#30805,10.);
#4291=VECTOR('',#30806,10.);
#4292=VECTOR('',#30807,10.);
#4293=VECTOR('',#30810,10.);
#4294=VECTOR('',#30811,10.);
#4295=VECTOR('',#30814,10.);
#4296=VECTOR('',#30817,10.);
#4297=VECTOR('',#30822,10.);
#4298=VECTOR('',#30823,10.);
#4299=VECTOR('',#30824,10.);
#4300=VECTOR('',#30825,10.);
#4301=VECTOR('',#30828,10.);
#4302=VECTOR('',#30829,10.);
#4303=VECTOR('',#30830,10.);
#4304=VECTOR('',#30833,10.);
#4305=VECTOR('',#30834,10.);
#4306=VECTOR('',#30835,10.);
#4307=VECTOR('',#30838,10.);
#4308=VECTOR('',#30841,10.);
#4309=VECTOR('',#30844,10.);
#4310=VECTOR('',#30845,10.);
#4311=VECTOR('',#30846,10.);
#4312=VECTOR('',#30849,10.);
#4313=VECTOR('',#30850,10.);
#4314=VECTOR('',#30853,10.);
#4315=VECTOR('',#30856,10.);
#4316=VECTOR('',#30857,10.);
#4317=VECTOR('',#30858,10.);
#4318=VECTOR('',#30859,10.);
#4319=VECTOR('',#30862,10.);
#4320=VECTOR('',#30863,10.);
#4321=VECTOR('',#30864,10.);
#4322=VECTOR('',#30867,10.);
#4323=VECTOR('',#30868,10.);
#4324=VECTOR('',#30869,10.);
#4325=VECTOR('',#30872,10.);
#4326=VECTOR('',#30875,10.);
#4327=VECTOR('',#30878,10.);
#4328=VECTOR('',#30879,10.);
#4329=VECTOR('',#30880,10.);
#4330=VECTOR('',#30883,10.);
#4331=VECTOR('',#30884,10.);
#4332=VECTOR('',#30887,10.);
#4333=VECTOR('',#30890,10.);
#4334=VECTOR('',#30891,10.);
#4335=VECTOR('',#30902,91.5);
#4336=VECTOR('',#30909,92.);
#4337=VECTOR('',#30934,10.);
#4338=VECTOR('',#30937,10.);
#4339=VECTOR('',#30940,10.);
#4340=VECTOR('',#30943,10.);
#4341=VECTOR('',#30946,10.);
#4342=VECTOR('',#30951,10.);
#4343=VECTOR('',#30954,10.);
#4344=VECTOR('',#30957,10.);
#4345=VECTOR('',#30960,10.);
#4346=VECTOR('',#31031,56.);
#4347=VECTOR('',#31034,10.);
#4348=VECTOR('',#31035,10.);
#4349=VECTOR('',#31036,10.);
#4350=VECTOR('',#31037,10.);
#4351=VECTOR('',#31038,10.);
#4352=VECTOR('',#31039,10.);
#4353=VECTOR('',#31040,10.);
#4354=VECTOR('',#31041,10.);
#4355=VECTOR('',#31042,10.);
#4356=VECTOR('',#31043,10.);
#4357=VECTOR('',#31044,10.);
#4358=VECTOR('',#31045,10.);
#4359=VECTOR('',#31046,10.);
#4360=VECTOR('',#31047,10.);
#4361=VECTOR('',#31048,10.);
#4362=VECTOR('',#31049,10.);
#4363=VECTOR('',#31050,10.);
#4364=VECTOR('',#31051,10.);
#4365=VECTOR('',#31052,10.);
#4366=VECTOR('',#31053,10.);
#4367=VECTOR('',#31054,10.);
#4368=VECTOR('',#31055,10.);
#4369=VECTOR('',#31056,1.5);
#4370=VECTOR('',#31057,10.);
#4371=VECTOR('',#31058,10.);
#4372=VECTOR('',#31059,1.5);
#4373=VECTOR('',#31060,10.);
#4374=VECTOR('',#31061,10.);
#4375=VECTOR('',#31062,1.5);
#4376=VECTOR('',#31063,10.);
#4377=VECTOR('',#31064,1.5);
#4378=VECTOR('',#31065,10.);
#4379=VECTOR('',#31066,10.);
#4380=VECTOR('',#31067,10.);
#4381=VECTOR('',#31068,10.);
#4382=VECTOR('',#31069,10.);
#4383=VECTOR('',#31070,10.);
#4384=VECTOR('',#31071,10.);
#4385=VECTOR('',#31072,10.);
#4386=VECTOR('',#31073,10.);
#4387=VECTOR('',#31074,1.5);
#4388=VECTOR('',#31077,10.);
#4389=VECTOR('',#31082,10.);
#4390=VECTOR('',#31089,10.);
#4391=VECTOR('',#31092,10.);
#4392=VECTOR('',#31101,10.);
#4393=VECTOR('',#31102,56.5);
#4394=VECTOR('',#31103,10.);
#4395=VECTOR('',#31106,10.);
#4396=VECTOR('',#31117,10.);
#4397=VECTOR('',#31118,10.);
#4398=VECTOR('',#31121,10.);
#4399=VECTOR('',#31122,10.);
#4400=VECTOR('',#31139,10.);
#4401=VECTOR('',#31142,70.2);
#4402=VECTOR('',#31145,10.);
#4403=VECTOR('',#31156,5.5);
#4404=VECTOR('',#31159,5.5);
#4405=VECTOR('',#31162,5.5);
#4406=VECTOR('',#31165,5.5);
#4407=VECTOR('',#31170,75.05);
#4408=VECTOR('',#31177,10.);
#4409=VECTOR('',#31184,10.);
#4410=VECTOR('',#31191,10.);
#4411=VECTOR('',#31200,10.);
#4412=VECTOR('',#31207,10.);
#4413=VECTOR('',#31210,10.);
#4414=VECTOR('',#31211,10.);
#4415=VECTOR('',#31212,10.);
#4416=VECTOR('',#31215,10.);
#4417=VECTOR('',#31216,10.);
#4418=VECTOR('',#31219,10.);
#4419=VECTOR('',#31222,10.);
#4420=VECTOR('',#31225,10.);
#4421=VECTOR('',#31226,10.);
#4422=VECTOR('',#31227,10.);
#4423=VECTOR('',#31228,10.);
#4424=VECTOR('',#31229,10.);
#4425=VECTOR('',#31232,10.);
#4426=VECTOR('',#31237,10.);
#4427=VECTOR('',#31238,10.);
#4428=VECTOR('',#31239,10.);
#4429=VECTOR('',#31242,10.);
#4430=VECTOR('',#31243,10.);
#4431=VECTOR('',#31246,10.);
#4432=VECTOR('',#31247,10.);
#4433=VECTOR('',#31250,10.);
#4434=VECTOR('',#31251,10.);
#4435=VECTOR('',#31254,10.);
#4436=VECTOR('',#31255,10.);
#4437=VECTOR('',#31258,10.);
#4438=VECTOR('',#31259,10.);
#4439=VECTOR('',#31262,10.);
#4440=VECTOR('',#31263,10.);
#4441=VECTOR('',#31266,10.);
#4442=VECTOR('',#31267,10.);
#4443=VECTOR('',#31270,10.);
#4444=VECTOR('',#31273,10.);
#4445=VECTOR('',#31274,10.);
#4446=VECTOR('',#31277,10.);
#4447=VECTOR('',#31280,10.);
#4448=VECTOR('',#31281,10.);
#4449=VECTOR('',#31282,10.);
#4450=VECTOR('',#31283,10.);
#4451=VECTOR('',#31284,10.);
#4452=VECTOR('',#31285,10.);
#4453=VECTOR('',#31286,10.);
#4454=VECTOR('',#31287,10.);
#4455=VECTOR('',#31288,10.);
#4456=VECTOR('',#31289,10.);
#4457=VECTOR('',#31290,10.);
#4458=VECTOR('',#31293,10.);
#4459=VECTOR('',#31296,10.);
#4460=VECTOR('',#31297,10.);
#4461=VECTOR('',#31300,10.);
#4462=VECTOR('',#31301,10.);
#4463=VECTOR('',#31302,10.);
#4464=VECTOR('',#31303,10.);
#4465=VECTOR('',#31304,10.);
#4466=VECTOR('',#31305,10.);
#4467=VECTOR('',#31306,10.);
#4468=VECTOR('',#31307,10.);
#4469=VECTOR('',#31308,10.);
#4470=VECTOR('',#31309,10.);
#4471=VECTOR('',#31310,10.);
#4472=VECTOR('',#31311,10.);
#4473=VECTOR('',#31312,10.);
#4474=VECTOR('',#31313,10.);
#4475=VECTOR('',#31316,10.);
#4476=VECTOR('',#31317,10.);
#4477=VECTOR('',#31318,10.);
#4478=VECTOR('',#31319,10.);
#4479=VECTOR('',#31320,10.);
#4480=VECTOR('',#31321,10.);
#4481=VECTOR('',#31322,10.);
#4482=VECTOR('',#31323,10.);
#4483=VECTOR('',#31324,10.);
#4484=VECTOR('',#31325,10.);
#4485=VECTOR('',#31326,10.);
#4486=VECTOR('',#31327,10.);
#4487=VECTOR('',#31328,10.);
#4488=VECTOR('',#31329,10.);
#4489=VECTOR('',#31330,10.);
#4490=VECTOR('',#31331,10.);
#4491=VECTOR('',#31332,10.);
#4492=VECTOR('',#31333,10.);
#4493=VECTOR('',#31334,10.);
#4494=VECTOR('',#31335,10.);
#4495=VECTOR('',#31338,10.);
#4496=VECTOR('',#31339,10.);
#4497=VECTOR('',#31340,10.);
#4498=VECTOR('',#31345,10.);
#4499=VECTOR('',#31346,10.);
#4500=VECTOR('',#31347,10.);
#4501=VECTOR('',#31348,10.);
#4502=VECTOR('',#31349,10.);
#4503=VECTOR('',#31350,10.);
#4504=VECTOR('',#31351,10.);
#4505=VECTOR('',#31354,10.);
#4506=VECTOR('',#31357,10.);
#4507=VECTOR('',#31358,10.);
#4508=VECTOR('',#31359,10.);
#4509=VECTOR('',#31360,10.);
#4510=VECTOR('',#31361,10.);
#4511=VECTOR('',#31362,10.);
#4512=VECTOR('',#31363,10.);
#4513=VECTOR('',#31364,10.);
#4514=VECTOR('',#31365,10.);
#4515=VECTOR('',#31368,10.);
#4516=VECTOR('',#31371,10.);
#4517=VECTOR('',#31372,10.);
#4518=VECTOR('',#31375,10.);
#4519=VECTOR('',#31380,10.);
#4520=VECTOR('',#31381,10.);
#4521=VECTOR('',#31382,10.);
#4522=VECTOR('',#31385,10.);
#4523=VECTOR('',#31386,10.);
#4524=VECTOR('',#31389,10.);
#4525=VECTOR('',#31390,10.);
#4526=VECTOR('',#31391,10.);
#4527=VECTOR('',#31392,10.);
#4528=VECTOR('',#31395,10.);
#4529=VECTOR('',#31396,10.);
#4530=VECTOR('',#31399,10.);
#4531=VECTOR('',#31400,10.);
#4532=VECTOR('',#31403,10.);
#4533=VECTOR('',#31404,10.);
#4534=VECTOR('',#31407,10.);
#4535=VECTOR('',#31408,10.);
#4536=VECTOR('',#31411,10.);
#4537=VECTOR('',#31412,10.);
#4538=VECTOR('',#31415,10.);
#4539=VECTOR('',#31420,5.5);
#4540=VECTOR('',#31423,5.5);
#4541=VECTOR('',#31426,5.5);
#4542=VECTOR('',#31429,5.5);
#4543=VECTOR('',#31434,10.);
#4544=VECTOR('',#31437,10.);
#4545=VECTOR('',#31440,10.);
#4546=VECTOR('',#31443,10.);
#6569=CYLINDRICAL_SURFACE('',#27790,1.5);
#6570=CYLINDRICAL_SURFACE('',#27793,1.5);
#6571=CYLINDRICAL_SURFACE('',#27798,1.5);
#6572=CYLINDRICAL_SURFACE('',#27804,1.5);
#6573=CYLINDRICAL_SURFACE('',#27807,1.5);
#6574=CYLINDRICAL_SURFACE('',#27812,1.5);
#6575=CYLINDRICAL_SURFACE('',#27815,1.5);
#6576=CYLINDRICAL_SURFACE('',#27823,92.);
#6577=CYLINDRICAL_SURFACE('',#27842,1.5);
#6578=CYLINDRICAL_SURFACE('',#27844,1.5);
#6579=CYLINDRICAL_SURFACE('',#27882,1.5);
#6580=CYLINDRICAL_SURFACE('',#27883,1.5);
#6581=CYLINDRICAL_SURFACE('',#27887,1.5);
#6582=CYLINDRICAL_SURFACE('',#27892,56.5);
#6583=CYLINDRICAL_SURFACE('',#27893,1.5);
#6584=CYLINDRICAL_SURFACE('',#27898,1.5);
#6585=CYLINDRICAL_SURFACE('',#27899,1.5);
#6586=CYLINDRICAL_SURFACE('',#27907,70.2);
#6587=CYLINDRICAL_SURFACE('',#27914,5.5);
#6588=CYLINDRICAL_SURFACE('',#27915,5.5);
#6589=CYLINDRICAL_SURFACE('',#27916,5.5);
#6590=CYLINDRICAL_SURFACE('',#27917,5.5);
#6591=CYLINDRICAL_SURFACE('',#27918,75.05);
#6592=CYLINDRICAL_SURFACE('',#27920,1.5);
#6593=CYLINDRICAL_SURFACE('',#27923,1.5);
#6594=CYLINDRICAL_SURFACE('',#27926,1.5);
#6595=CYLINDRICAL_SURFACE('',#27929,1.5);
#6596=CYLINDRICAL_SURFACE('',#27933,1.5);
#6597=CYLINDRICAL_SURFACE('',#27978,5.5);
#6598=CYLINDRICAL_SURFACE('',#27979,5.5);
#6599=CYLINDRICAL_SURFACE('',#27980,5.5);
#6600=CYLINDRICAL_SURFACE('',#27981,5.5);
#6601=CYLINDRICAL_SURFACE('',#27983,57.);
#6984=FACE_OUTER_BOUND('',#8580,.T.);
#6985=FACE_OUTER_BOUND('',#8581,.T.);
#6986=FACE_OUTER_BOUND('',#8582,.T.);
#6987=FACE_OUTER_BOUND('',#8583,.T.);
#6988=FACE_OUTER_BOUND('',#8584,.T.);
#6989=FACE_OUTER_BOUND('',#8585,.T.);
#6990=FACE_OUTER_BOUND('',#8586,.T.);
#6991=FACE_OUTER_BOUND('',#8587,.T.);
#6992=FACE_OUTER_BOUND('',#8588,.T.);
#6993=FACE_OUTER_BOUND('',#8589,.T.);
#6994=FACE_OUTER_BOUND('',#8590,.T.);
#6995=FACE_OUTER_BOUND('',#8591,.T.);
#6996=FACE_OUTER_BOUND('',#8592,.T.);
#6997=FACE_OUTER_BOUND('',#8593,.T.);
#6998=FACE_OUTER_BOUND('',#8594,.T.);
#6999=FACE_OUTER_BOUND('',#8595,.T.);
#7000=FACE_OUTER_BOUND('',#8596,.T.);
#7001=FACE_OUTER_BOUND('',#8597,.T.);
#7002=FACE_OUTER_BOUND('',#8598,.T.);
#7003=FACE_OUTER_BOUND('',#8599,.T.);
#7004=FACE_OUTER_BOUND('',#8600,.T.);
#7005=FACE_OUTER_BOUND('',#8601,.T.);
#7006=FACE_OUTER_BOUND('',#8602,.T.);
#7007=FACE_OUTER_BOUND('',#8603,.T.);
#7008=FACE_OUTER_BOUND('',#8604,.T.);
#7009=FACE_OUTER_BOUND('',#8605,.T.);
#7010=FACE_OUTER_BOUND('',#8606,.T.);
#7011=FACE_OUTER_BOUND('',#8607,.T.);
#7012=FACE_OUTER_BOUND('',#8608,.T.);
#7013=FACE_OUTER_BOUND('',#8609,.T.);
#7014=FACE_OUTER_BOUND('',#8610,.T.);
#7015=FACE_OUTER_BOUND('',#8611,.T.);
#7016=FACE_OUTER_BOUND('',#8612,.T.);
#7017=FACE_OUTER_BOUND('',#8613,.T.);
#7018=FACE_OUTER_BOUND('',#8614,.T.);
#7019=FACE_OUTER_BOUND('',#8615,.T.);
#7020=FACE_OUTER_BOUND('',#8616,.T.);
#7021=FACE_OUTER_BOUND('',#8617,.T.);
#7022=FACE_OUTER_BOUND('',#8618,.T.);
#7023=FACE_OUTER_BOUND('',#8619,.T.);
#7024=FACE_OUTER_BOUND('',#8620,.T.);
#7025=FACE_OUTER_BOUND('',#8621,.T.);
#7026=FACE_OUTER_BOUND('',#8622,.T.);
#7027=FACE_OUTER_BOUND('',#8623,.T.);
#7028=FACE_OUTER_BOUND('',#8633,.T.);
#7029=FACE_OUTER_BOUND('',#8634,.T.);
#7030=FACE_OUTER_BOUND('',#8635,.T.);
#7031=FACE_OUTER_BOUND('',#8636,.T.);
#7032=FACE_OUTER_BOUND('',#8637,.T.);
#7033=FACE_OUTER_BOUND('',#8638,.T.);
#7034=FACE_OUTER_BOUND('',#8640,.T.);
#7035=FACE_OUTER_BOUND('',#8641,.T.);
#7036=FACE_OUTER_BOUND('',#8642,.T.);
#7037=FACE_OUTER_BOUND('',#8648,.T.);
#7038=FACE_OUTER_BOUND('',#8649,.T.);
#7039=FACE_OUTER_BOUND('',#8650,.T.);
#7040=FACE_OUTER_BOUND('',#8651,.T.);
#7041=FACE_OUTER_BOUND('',#8652,.T.);
#7042=FACE_OUTER_BOUND('',#8653,.T.);
#7043=FACE_OUTER_BOUND('',#8654,.T.);
#7044=FACE_OUTER_BOUND('',#8655,.T.);
#7045=FACE_OUTER_BOUND('',#8656,.T.);
#7046=FACE_OUTER_BOUND('',#8657,.T.);
#7047=FACE_OUTER_BOUND('',#8658,.T.);
#7048=FACE_OUTER_BOUND('',#8659,.T.);
#7049=FACE_OUTER_BOUND('',#8660,.T.);
#7050=FACE_OUTER_BOUND('',#8661,.T.);
#7051=FACE_OUTER_BOUND('',#8662,.T.);
#7052=FACE_OUTER_BOUND('',#8663,.T.);
#7053=FACE_OUTER_BOUND('',#8664,.T.);
#7054=FACE_OUTER_BOUND('',#8665,.T.);
#7055=FACE_OUTER_BOUND('',#8666,.T.);
#7056=FACE_OUTER_BOUND('',#8667,.T.);
#7057=FACE_OUTER_BOUND('',#8668,.T.);
#7058=FACE_OUTER_BOUND('',#8669,.T.);
#7059=FACE_OUTER_BOUND('',#8670,.T.);
#7060=FACE_OUTER_BOUND('',#8671,.T.);
#7061=FACE_OUTER_BOUND('',#8672,.T.);
#7062=FACE_OUTER_BOUND('',#8673,.T.);
#7063=FACE_OUTER_BOUND('',#8674,.T.);
#7064=FACE_OUTER_BOUND('',#8675,.T.);
#7065=FACE_OUTER_BOUND('',#8676,.T.);
#7066=FACE_OUTER_BOUND('',#8677,.T.);
#7067=FACE_OUTER_BOUND('',#8678,.T.);
#7068=FACE_OUTER_BOUND('',#8679,.T.);
#7069=FACE_OUTER_BOUND('',#8680,.T.);
#7070=FACE_OUTER_BOUND('',#8681,.T.);
#7071=FACE_OUTER_BOUND('',#8682,.T.);
#7072=FACE_OUTER_BOUND('',#8683,.T.);
#7073=FACE_OUTER_BOUND('',#8684,.T.);
#7074=FACE_OUTER_BOUND('',#8685,.T.);
#7075=FACE_OUTER_BOUND('',#8686,.T.);
#7076=FACE_OUTER_BOUND('',#8687,.T.);
#7077=FACE_OUTER_BOUND('',#8688,.T.);
#7078=FACE_OUTER_BOUND('',#8689,.T.);
#7079=FACE_OUTER_BOUND('',#8690,.T.);
#7080=FACE_OUTER_BOUND('',#8691,.T.);
#7081=FACE_OUTER_BOUND('',#8692,.T.);
#7082=FACE_OUTER_BOUND('',#8693,.T.);
#7083=FACE_OUTER_BOUND('',#8694,.T.);
#7084=FACE_OUTER_BOUND('',#8695,.T.);
#7085=FACE_OUTER_BOUND('',#8696,.T.);
#7086=FACE_OUTER_BOUND('',#8697,.T.);
#7087=FACE_OUTER_BOUND('',#8698,.T.);
#7088=FACE_OUTER_BOUND('',#8699,.T.);
#7089=FACE_OUTER_BOUND('',#8700,.T.);
#7090=FACE_OUTER_BOUND('',#8701,.T.);
#7091=FACE_OUTER_BOUND('',#8702,.T.);
#7092=FACE_OUTER_BOUND('',#8703,.T.);
#7093=FACE_OUTER_BOUND('',#8704,.T.);
#7094=FACE_OUTER_BOUND('',#8705,.T.);
#7095=FACE_OUTER_BOUND('',#8706,.T.);
#7096=FACE_OUTER_BOUND('',#8707,.T.);
#7097=FACE_OUTER_BOUND('',#8708,.T.);
#7098=FACE_OUTER_BOUND('',#8709,.T.);
#7099=FACE_OUTER_BOUND('',#8710,.T.);
#7100=FACE_OUTER_BOUND('',#8711,.T.);
#7101=FACE_OUTER_BOUND('',#8712,.T.);
#7102=FACE_OUTER_BOUND('',#8713,.T.);
#7103=FACE_OUTER_BOUND('',#8714,.T.);
#7104=FACE_OUTER_BOUND('',#8715,.T.);
#7105=FACE_OUTER_BOUND('',#8716,.T.);
#7106=FACE_OUTER_BOUND('',#8717,.T.);
#7107=FACE_OUTER_BOUND('',#8718,.T.);
#7108=FACE_OUTER_BOUND('',#8719,.T.);
#7109=FACE_OUTER_BOUND('',#8720,.T.);
#7110=FACE_OUTER_BOUND('',#8721,.T.);
#7111=FACE_OUTER_BOUND('',#8722,.T.);
#7112=FACE_OUTER_BOUND('',#8723,.T.);
#7113=FACE_OUTER_BOUND('',#8724,.T.);
#7114=FACE_OUTER_BOUND('',#8725,.T.);
#7115=FACE_OUTER_BOUND('',#8726,.T.);
#7116=FACE_OUTER_BOUND('',#8727,.T.);
#7117=FACE_OUTER_BOUND('',#8728,.T.);
#7118=FACE_OUTER_BOUND('',#8729,.T.);
#7119=FACE_OUTER_BOUND('',#8730,.T.);
#7120=FACE_OUTER_BOUND('',#8731,.T.);
#7121=FACE_OUTER_BOUND('',#8732,.T.);
#7122=FACE_OUTER_BOUND('',#8733,.T.);
#7123=FACE_OUTER_BOUND('',#8734,.T.);
#7124=FACE_OUTER_BOUND('',#8735,.T.);
#7125=FACE_OUTER_BOUND('',#8736,.T.);
#7126=FACE_OUTER_BOUND('',#8737,.T.);
#7127=FACE_OUTER_BOUND('',#8738,.T.);
#7128=FACE_OUTER_BOUND('',#8739,.T.);
#7129=FACE_OUTER_BOUND('',#8740,.T.);
#7130=FACE_OUTER_BOUND('',#8741,.T.);
#7131=FACE_OUTER_BOUND('',#8742,.T.);
#7132=FACE_OUTER_BOUND('',#8743,.T.);
#7133=FACE_OUTER_BOUND('',#8744,.T.);
#7134=FACE_OUTER_BOUND('',#8745,.T.);
#7135=FACE_OUTER_BOUND('',#8746,.T.);
#7136=FACE_OUTER_BOUND('',#8747,.T.);
#7137=FACE_OUTER_BOUND('',#8748,.T.);
#7138=FACE_OUTER_BOUND('',#8749,.T.);
#7139=FACE_OUTER_BOUND('',#8750,.T.);
#7140=FACE_OUTER_BOUND('',#8751,.T.);
#7141=FACE_OUTER_BOUND('',#8752,.T.);
#7142=FACE_OUTER_BOUND('',#8753,.T.);
#7143=FACE_OUTER_BOUND('',#8754,.T.);
#7144=FACE_OUTER_BOUND('',#8755,.T.);
#7145=FACE_OUTER_BOUND('',#8756,.T.);
#7146=FACE_OUTER_BOUND('',#8757,.T.);
#7147=FACE_OUTER_BOUND('',#8758,.T.);
#7148=FACE_OUTER_BOUND('',#8759,.T.);
#7149=FACE_OUTER_BOUND('',#8760,.T.);
#7150=FACE_OUTER_BOUND('',#8761,.T.);
#7151=FACE_OUTER_BOUND('',#8762,.T.);
#7152=FACE_OUTER_BOUND('',#8763,.T.);
#7153=FACE_OUTER_BOUND('',#8764,.T.);
#7154=FACE_OUTER_BOUND('',#8765,.T.);
#7155=FACE_OUTER_BOUND('',#8766,.T.);
#7156=FACE_OUTER_BOUND('',#8767,.T.);
#7157=FACE_OUTER_BOUND('',#8768,.T.);
#7158=FACE_OUTER_BOUND('',#8769,.T.);
#7159=FACE_OUTER_BOUND('',#8770,.T.);
#7160=FACE_OUTER_BOUND('',#8771,.T.);
#7161=FACE_OUTER_BOUND('',#8772,.T.);
#7162=FACE_OUTER_BOUND('',#8773,.T.);
#7163=FACE_OUTER_BOUND('',#8774,.T.);
#7164=FACE_OUTER_BOUND('',#8775,.T.);
#7165=FACE_OUTER_BOUND('',#8776,.T.);
#7166=FACE_OUTER_BOUND('',#8777,.T.);
#7167=FACE_OUTER_BOUND('',#8779,.T.);
#7168=FACE_OUTER_BOUND('',#8780,.T.);
#7169=FACE_OUTER_BOUND('',#8781,.T.);
#7170=FACE_OUTER_BOUND('',#8782,.T.);
#7171=FACE_OUTER_BOUND('',#8783,.T.);
#8580=EDGE_LOOP('',(#18492,#18493,#18494,#18495));
#8581=EDGE_LOOP('',(#18496,#18497,#18498,#18499));
#8582=EDGE_LOOP('',(#18500,#18501,#18502,#18503));
#8583=EDGE_LOOP('',(#18504,#18505,#18506,#18507,#18508,#18509,#18510));
#8584=EDGE_LOOP('',(#18511,#18512,#18513,#18514,#18515,#18516));
#8585=EDGE_LOOP('',(#18517,#18518,#18519,#18520));
#8586=EDGE_LOOP('',(#18521,#18522,#18523,#18524));
#8587=EDGE_LOOP('',(#18525,#18526,#18527,#18528));
#8588=EDGE_LOOP('',(#18529,#18530,#18531,#18532));
#8589=EDGE_LOOP('',(#18533,#18534,#18535,#18536,#18537));
#8590=EDGE_LOOP('',(#18538,#18539,#18540,#18541));
#8591=EDGE_LOOP('',(#18542,#18543,#18544,#18545));
#8592=EDGE_LOOP('',(#18546,#18547,#18548,#18549));
#8593=EDGE_LOOP('',(#18550,#18551,#18552,#18553));
#8594=EDGE_LOOP('',(#18554,#18555,#18556,#18557,#18558));
#8595=EDGE_LOOP('',(#18559,#18560,#18561,#18562,#18563));
#8596=EDGE_LOOP('',(#18564,#18565,#18566,#18567));
#8597=EDGE_LOOP('',(#18568,#18569,#18570,#18571));
#8598=EDGE_LOOP('',(#18572,#18573,#18574,#18575));
#8599=EDGE_LOOP('',(#18576,#18577,#18578,#18579));
#8600=EDGE_LOOP('',(#18580,#18581,#18582,#18583,#18584,#18585));
#8601=EDGE_LOOP('',(#18586,#18587,#18588,#18589,#18590,#18591));
#8602=EDGE_LOOP('',(#18592,#18593,#18594,#18595));
#8603=EDGE_LOOP('',(#18596,#18597,#18598,#18599));
#8604=EDGE_LOOP('',(#18600,#18601,#18602,#18603));
#8605=EDGE_LOOP('',(#18604,#18605,#18606,#18607));
#8606=EDGE_LOOP('',(#18608,#18609,#18610,#18611,#18612));
#8607=EDGE_LOOP('',(#18613,#18614,#18615,#18616));
#8608=EDGE_LOOP('',(#18617,#18618,#18619,#18620));
#8609=EDGE_LOOP('',(#18621,#18622,#18623,#18624));
#8610=EDGE_LOOP('',(#18625,#18626,#18627,#18628));
#8611=EDGE_LOOP('',(#18629,#18630,#18631,#18632,#18633,#18634));
#8612=EDGE_LOOP('',(#18635,#18636,#18637,#18638,#18639,#18640));
#8613=EDGE_LOOP('',(#18641,#18642,#18643,#18644));
#8614=EDGE_LOOP('',(#18645,#18646,#18647,#18648));
#8615=EDGE_LOOP('',(#18649,#18650,#18651,#18652));
#8616=EDGE_LOOP('',(#18653,#18654,#18655,#18656));
#8617=EDGE_LOOP('',(#18657,#18658,#18659,#18660,#18661));
#8618=EDGE_LOOP('',(#18662,#18663,#18664,#18665));
#8619=EDGE_LOOP('',(#18666,#18667,#18668,#18669));
#8620=EDGE_LOOP('',(#18670,#18671,#18672,#18673));
#8621=EDGE_LOOP('',(#18674,#18675,#18676,#18677));
#8622=EDGE_LOOP('',(#18678,#18679,#18680,#18681));
#8623=EDGE_LOOP('',(#18682));
#8624=EDGE_LOOP('',(#18683));
#8625=EDGE_LOOP('',(#18684));
#8626=EDGE_LOOP('',(#18685));
#8627=EDGE_LOOP('',(#18686));
#8628=EDGE_LOOP('',(#18687));
#8629=EDGE_LOOP('',(#18688));
#8630=EDGE_LOOP('',(#18689));
#8631=EDGE_LOOP('',(#18690));
#8632=EDGE_LOOP('',(#18691,#18692,#18693,#18694,#18695,#18696,#18697,#18698,
#18699,#18700,#18701,#18702,#18703,#18704,#18705,#18706,#18707,#18708,#18709,
#18710,#18711,#18712,#18713,#18714));
#8633=EDGE_LOOP('',(#18715,#18716,#18717,#18718,#18719));
#8634=EDGE_LOOP('',(#18720,#18721,#18722,#18723));
#8635=EDGE_LOOP('',(#18724,#18725,#18726,#18727,#18728));
#8636=EDGE_LOOP('',(#18729,#18730,#18731,#18732));
#8637=EDGE_LOOP('',(#18733,#18734,#18735,#18736));
#8638=EDGE_LOOP('',(#18737));
#8639=EDGE_LOOP('',(#18738,#18739,#18740,#18741,#18742,#18743,#18744,#18745,
#18746,#18747,#18748,#18749,#18750,#18751,#18752,#18753,#18754,#18755,#18756,
#18757,#18758,#18759,#18760,#18761,#18762));
#8640=EDGE_LOOP('',(#18763,#18764,#18765,#18766));
#8641=EDGE_LOOP('',(#18767,#18768,#18769,#18770));
#8642=EDGE_LOOP('',(#18771));
#8643=EDGE_LOOP('',(#18772,#18773,#18774,#18775,#18776,#18777,#18778,#18779,
#18780,#18781,#18782,#18783,#18784,#18785,#18786,#18787,#18788,#18789,#18790,
#18791,#18792,#18793,#18794,#18795,#18796,#18797,#18798,#18799,#18800,#18801,
#18802,#18803,#18804,#18805,#18806));
#8644=EDGE_LOOP('',(#18807,#18808,#18809,#18810,#18811,#18812,#18813,#18814,
#18815,#18816,#18817));
#8645=EDGE_LOOP('',(#18818,#18819,#18820,#18821,#18822,#18823,#18824,#18825,
#18826,#18827,#18828,#18829));
#8646=EDGE_LOOP('',(#18830,#18831,#18832,#18833,#18834,#18835,#18836,#18837,
#18838,#18839,#18840,#18841,#18842,#18843));
#8647=EDGE_LOOP('',(#18844,#18845,#18846,#18847,#18848,#18849,#18850,#18851,
#18852,#18853,#18854,#18855,#18856,#18857,#18858,#18859,#18860,#18861,#18862,
#18863,#18864,#18865,#18866,#18867,#18868,#18869));
#8648=EDGE_LOOP('',(#18870,#18871,#18872,#18873,#18874));
#8649=EDGE_LOOP('',(#18875,#18876,#18877,#18878));
#8650=EDGE_LOOP('',(#18879,#18880,#18881));
#8651=EDGE_LOOP('',(#18882,#18883,#18884,#18885));
#8652=EDGE_LOOP('',(#18886,#18887,#18888,#18889));
#8653=EDGE_LOOP('',(#18890,#18891,#18892,#18893));
#8654=EDGE_LOOP('',(#18894,#18895,#18896,#18897,#18898,#18899,#18900,#18901,
#18902,#18903,#18904,#18905,#18906,#18907,#18908,#18909,#18910,#18911,#18912,
#18913,#18914,#18915,#18916,#18917,#18918,#18919,#18920,#18921));
#8655=EDGE_LOOP('',(#18922,#18923,#18924,#18925,#18926));
#8656=EDGE_LOOP('',(#18927,#18928,#18929,#18930));
#8657=EDGE_LOOP('',(#18931,#18932,#18933,#18934));
#8658=EDGE_LOOP('',(#18935,#18936,#18937,#18938));
#8659=EDGE_LOOP('',(#18939,#18940,#18941,#18942));
#8660=EDGE_LOOP('',(#18943,#18944,#18945,#18946));
#8661=EDGE_LOOP('',(#18947,#18948,#18949,#18950,#18951));
#8662=EDGE_LOOP('',(#18952,#18953,#18954,#18955,#18956,#18957,#18958,#18959,
#18960,#18961,#18962));
#8663=EDGE_LOOP('',(#18963,#18964,#18965,#18966,#18967,#18968,#18969,#18970,
#18971,#18972,#18973,#18974,#18975,#18976,#18977,#18978,#18979,#18980,#18981,
#18982,#18983));
#8664=EDGE_LOOP('',(#18984,#18985,#18986,#18987,#18988,#18989));
#8665=EDGE_LOOP('',(#18990,#18991,#18992,#18993,#18994,#18995));
#8666=EDGE_LOOP('',(#18996,#18997,#18998,#18999,#19000,#19001));
#8667=EDGE_LOOP('',(#19002,#19003,#19004,#19005,#19006,#19007));
#8668=EDGE_LOOP('',(#19008,#19009,#19010,#19011,#19012));
#8669=EDGE_LOOP('',(#19013,#19014,#19015,#19016));
#8670=EDGE_LOOP('',(#19017,#19018,#19019,#19020));
#8671=EDGE_LOOP('',(#19021,#19022,#19023,#19024));
#8672=EDGE_LOOP('',(#19025,#19026,#19027,#19028,#19029));
#8673=EDGE_LOOP('',(#19030,#19031,#19032,#19033));
#8674=EDGE_LOOP('',(#19034,#19035,#19036,#19037));
#8675=EDGE_LOOP('',(#19038,#19039,#19040,#19041));
#8676=EDGE_LOOP('',(#19042,#19043,#19044,#19045));
#8677=EDGE_LOOP('',(#19046,#19047,#19048,#19049));
#8678=EDGE_LOOP('',(#19050,#19051,#19052,#19053,#19054,#19055,#19056));
#8679=EDGE_LOOP('',(#19057,#19058,#19059,#19060));
#8680=EDGE_LOOP('',(#19061,#19062,#19063,#19064,#19065,#19066,#19067,#19068));
#8681=EDGE_LOOP('',(#19069,#19070,#19071,#19072));
#8682=EDGE_LOOP('',(#19073,#19074,#19075,#19076));
#8683=EDGE_LOOP('',(#19077,#19078,#19079,#19080));
#8684=EDGE_LOOP('',(#19081,#19082,#19083,#19084));
#8685=EDGE_LOOP('',(#19085,#19086,#19087,#19088));
#8686=EDGE_LOOP('',(#19089,#19090,#19091,#19092));
#8687=EDGE_LOOP('',(#19093,#19094,#19095,#19096));
#8688=EDGE_LOOP('',(#19097,#19098,#19099,#19100));
#8689=EDGE_LOOP('',(#19101,#19102,#19103,#19104));
#8690=EDGE_LOOP('',(#19105,#19106,#19107,#19108));
#8691=EDGE_LOOP('',(#19109,#19110,#19111,#19112));
#8692=EDGE_LOOP('',(#19113,#19114,#19115,#19116,#19117,#19118,#19119,#19120,
#19121,#19122,#19123,#19124));
#8693=EDGE_LOOP('',(#19125,#19126,#19127,#19128));
#8694=EDGE_LOOP('',(#19129,#19130,#19131,#19132));
#8695=EDGE_LOOP('',(#19133,#19134,#19135,#19136));
#8696=EDGE_LOOP('',(#19137,#19138,#19139,#19140));
#8697=EDGE_LOOP('',(#19141,#19142,#19143,#19144));
#8698=EDGE_LOOP('',(#19145,#19146,#19147,#19148));
#8699=EDGE_LOOP('',(#19149,#19150,#19151,#19152));
#8700=EDGE_LOOP('',(#19153,#19154,#19155,#19156));
#8701=EDGE_LOOP('',(#19157,#19158,#19159,#19160));
#8702=EDGE_LOOP('',(#19161,#19162,#19163,#19164));
#8703=EDGE_LOOP('',(#19165,#19166,#19167,#19168));
#8704=EDGE_LOOP('',(#19169,#19170,#19171,#19172));
#8705=EDGE_LOOP('',(#19173,#19174,#19175,#19176));
#8706=EDGE_LOOP('',(#19177,#19178,#19179,#19180,#19181,#19182,#19183,#19184,
#19185,#19186,#19187,#19188,#19189,#19190));
#8707=EDGE_LOOP('',(#19191,#19192,#19193,#19194));
#8708=EDGE_LOOP('',(#19195,#19196,#19197,#19198));
#8709=EDGE_LOOP('',(#19199,#19200,#19201,#19202));
#8710=EDGE_LOOP('',(#19203,#19204,#19205,#19206));
#8711=EDGE_LOOP('',(#19207,#19208,#19209,#19210));
#8712=EDGE_LOOP('',(#19211,#19212,#19213,#19214));
#8713=EDGE_LOOP('',(#19215,#19216,#19217,#19218));
#8714=EDGE_LOOP('',(#19219,#19220,#19221,#19222));
#8715=EDGE_LOOP('',(#19223,#19224,#19225,#19226));
#8716=EDGE_LOOP('',(#19227,#19228,#19229,#19230));
#8717=EDGE_LOOP('',(#19231,#19232,#19233,#19234));
#8718=EDGE_LOOP('',(#19235,#19236,#19237,#19238));
#8719=EDGE_LOOP('',(#19239,#19240,#19241,#19242));
#8720=EDGE_LOOP('',(#19243,#19244,#19245,#19246));
#8721=EDGE_LOOP('',(#19247,#19248,#19249,#19250));
#8722=EDGE_LOOP('',(#19251,#19252,#19253,#19254));
#8723=EDGE_LOOP('',(#19255,#19256,#19257,#19258));
#8724=EDGE_LOOP('',(#19259,#19260,#19261,#19262));
#8725=EDGE_LOOP('',(#19263,#19264,#19265,#19266));
#8726=EDGE_LOOP('',(#19267,#19268,#19269,#19270));
#8727=EDGE_LOOP('',(#19271,#19272,#19273,#19274));
#8728=EDGE_LOOP('',(#19275,#19276,#19277,#19278));
#8729=EDGE_LOOP('',(#19279,#19280,#19281,#19282));
#8730=EDGE_LOOP('',(#19283,#19284,#19285,#19286));
#8731=EDGE_LOOP('',(#19287,#19288,#19289,#19290));
#8732=EDGE_LOOP('',(#19291,#19292,#19293,#19294));
#8733=EDGE_LOOP('',(#19295,#19296,#19297,#19298));
#8734=EDGE_LOOP('',(#19299,#19300,#19301,#19302));
#8735=EDGE_LOOP('',(#19303,#19304,#19305,#19306));
#8736=EDGE_LOOP('',(#19307,#19308,#19309,#19310));
#8737=EDGE_LOOP('',(#19311,#19312,#19313,#19314));
#8738=EDGE_LOOP('',(#19315,#19316,#19317,#19318));
#8739=EDGE_LOOP('',(#19319,#19320,#19321,#19322));
#8740=EDGE_LOOP('',(#19323,#19324,#19325,#19326));
#8741=EDGE_LOOP('',(#19327,#19328,#19329,#19330));
#8742=EDGE_LOOP('',(#19331,#19332,#19333,#19334,#19335,#19336,#19337,#19338,
#19339,#19340,#19341,#19342,#19343,#19344,#19345,#19346,#19347,#19348,#19349,
#19350,#19351,#19352,#19353,#19354,#19355,#19356,#19357,#19358,#19359,#19360,
#19361,#19362,#19363,#19364,#19365));
#8743=EDGE_LOOP('',(#19366,#19367,#19368,#19369));
#8744=EDGE_LOOP('',(#19370,#19371,#19372,#19373));
#8745=EDGE_LOOP('',(#19374,#19375,#19376,#19377));
#8746=EDGE_LOOP('',(#19378,#19379,#19380,#19381));
#8747=EDGE_LOOP('',(#19382,#19383,#19384,#19385));
#8748=EDGE_LOOP('',(#19386,#19387,#19388,#19389));
#8749=EDGE_LOOP('',(#19390,#19391,#19392,#19393,#19394));
#8750=EDGE_LOOP('',(#19395,#19396,#19397,#19398));
#8751=EDGE_LOOP('',(#19399,#19400,#19401,#19402));
#8752=EDGE_LOOP('',(#19403,#19404,#19405,#19406));
#8753=EDGE_LOOP('',(#19407,#19408,#19409,#19410));
#8754=EDGE_LOOP('',(#19411,#19412,#19413,#19414));
#8755=EDGE_LOOP('',(#19415,#19416,#19417,#19418));
#8756=EDGE_LOOP('',(#19419,#19420,#19421,#19422));
#8757=EDGE_LOOP('',(#19423,#19424,#19425,#19426));
#8758=EDGE_LOOP('',(#19427,#19428,#19429,#19430));
#8759=EDGE_LOOP('',(#19431,#19432,#19433,#19434));
#8760=EDGE_LOOP('',(#19435,#19436,#19437,#19438,#19439,#19440,#19441,#19442,
#19443,#19444,#19445,#19446,#19447,#19448,#19449,#19450,#19451,#19452,#19453));
#8761=EDGE_LOOP('',(#19454,#19455,#19456,#19457));
#8762=EDGE_LOOP('',(#19458,#19459,#19460,#19461));
#8763=EDGE_LOOP('',(#19462,#19463,#19464,#19465));
#8764=EDGE_LOOP('',(#19466,#19467,#19468,#19469));
#8765=EDGE_LOOP('',(#19470,#19471,#19472,#19473));
#8766=EDGE_LOOP('',(#19474,#19475,#19476,#19477));
#8767=EDGE_LOOP('',(#19478,#19479,#19480,#19481));
#8768=EDGE_LOOP('',(#19482,#19483,#19484,#19485));
#8769=EDGE_LOOP('',(#19486,#19487,#19488,#19489));
#8770=EDGE_LOOP('',(#19490,#19491,#19492,#19493));
#8771=EDGE_LOOP('',(#19494,#19495,#19496,#19497));
#8772=EDGE_LOOP('',(#19498,#19499,#19500,#19501,#19502,#19503,#19504,#19505,
#19506,#19507,#19508));
#8773=EDGE_LOOP('',(#19509,#19510,#19511,#19512,#19513,#19514));
#8774=EDGE_LOOP('',(#19515,#19516,#19517,#19518,#19519,#19520));
#8775=EDGE_LOOP('',(#19521,#19522,#19523,#19524,#19525,#19526));
#8776=EDGE_LOOP('',(#19527,#19528,#19529,#19530,#19531,#19532));
#8777=EDGE_LOOP('',(#19533));
#8778=EDGE_LOOP('',(#19534));
#8779=EDGE_LOOP('',(#19535,#19536,#19537,#19538));
#8780=EDGE_LOOP('',(#19539,#19540,#19541,#19542));
#8781=EDGE_LOOP('',(#19543,#19544,#19545,#19546));
#8782=EDGE_LOOP('',(#19547,#19548,#19549,#19550,#19551));
#8783=EDGE_LOOP('',(#19552,#19553,#19554,#19555));
#10303=CIRCLE('',#27788,56.5);
#10304=CIRCLE('',#27789,56.5);
#10305=CIRCLE('',#27797,56.5);
#10306=CIRCLE('',#27799,1.5);
#10307=CIRCLE('',#27803,56.5);
#10308=CIRCLE('',#27811,56.5);
#10309=CIRCLE('',#27818,92.);
#10310=CIRCLE('',#27819,1.5);
#10311=CIRCLE('',#27820,91.5606601717798);
#10312=CIRCLE('',#27822,91.4393398282202);
#10313=CIRCLE('',#27824,92.);
#10314=CIRCLE('',#27826,1.5);
#10315=CIRCLE('',#27827,90.3786796564403);
#10316=CIRCLE('',#27829,5.5);
#10317=CIRCLE('',#27830,5.5);
#10318=CIRCLE('',#27831,5.5);
#10319=CIRCLE('',#27832,5.5);
#10320=CIRCLE('',#27833,5.5);
#10321=CIRCLE('',#27834,5.5);
#10322=CIRCLE('',#27835,5.5);
#10323=CIRCLE('',#27836,5.5);
#10324=CIRCLE('',#27837,56.5);
#10325=CIRCLE('',#27838,1.5);
#10326=CIRCLE('',#27839,56.5);
#10327=CIRCLE('',#27840,56.5);
#10328=CIRCLE('',#27841,56.5);
#10329=CIRCLE('',#27847,90.5);
#10330=CIRCLE('',#27848,1.5);
#10331=CIRCLE('',#27850,76.55);
#10332=CIRCLE('',#27851,5.5);
#10333=CIRCLE('',#27852,5.5);
#10334=CIRCLE('',#27853,76.55);
#10335=CIRCLE('',#27854,5.5);
#10336=CIRCLE('',#27855,5.5);
#10337=CIRCLE('',#27856,76.55);
#10338=CIRCLE('',#27857,5.5);
#10339=CIRCLE('',#27858,5.5);
#10340=CIRCLE('',#27859,76.55);
#10341=CIRCLE('',#27860,5.5);
#10342=CIRCLE('',#27861,5.5);
#10343=CIRCLE('',#27862,76.55);
#10344=CIRCLE('',#27863,5.5);
#10345=CIRCLE('',#27864,5.5);
#10346=CIRCLE('',#27865,76.55);
#10347=CIRCLE('',#27866,5.5);
#10348=CIRCLE('',#27867,5.5);
#10349=CIRCLE('',#27868,76.55);
#10350=CIRCLE('',#27869,76.55);
#10351=CIRCLE('',#27870,5.5);
#10352=CIRCLE('',#27871,5.5);
#10353=CIRCLE('',#27872,76.55);
#10354=CIRCLE('',#27873,5.5);
#10355=CIRCLE('',#27874,5.5);
#10356=CIRCLE('',#27876,55.9393398282202);
#10357=CIRCLE('',#27877,1.5);
#10358=CIRCLE('',#27878,54.8786796564404);
#10359=CIRCLE('',#27880,56.0606601717798);
#10360=CIRCLE('',#27884,1.5);
#10361=CIRCLE('',#27886,1.5);
#10362=CIRCLE('',#27890,56.5);
#10363=CIRCLE('',#27891,1.5);
#10364=CIRCLE('',#27896,55.5);
#10365=CIRCLE('',#27897,57.);
#10366=CIRCLE('',#27901,70.2);
#10367=CIRCLE('',#27903,70.2);
#10368=CIRCLE('',#27904,70.2);
#10369=CIRCLE('',#27905,1.5);
#10370=CIRCLE('',#27906,71.95);
#10371=CIRCLE('',#27908,70.2);
#10372=CIRCLE('',#27909,70.2);
#10373=CIRCLE('',#27911,1.5);
#10374=CIRCLE('',#27912,75.05);
#10375=CIRCLE('',#27913,75.05);
#10376=CIRCLE('',#27919,75.05);
#10377=CIRCLE('',#27921,1.5);
#10378=CIRCLE('',#27922,1.5);
#10379=CIRCLE('',#27924,1.5);
#10380=CIRCLE('',#27925,1.5);
#10381=CIRCLE('',#27927,1.5);
#10382=CIRCLE('',#27928,1.5);
#10383=CIRCLE('',#27984,57.);
#10998=B_SPLINE_CURVE_WITH_KNOTS('',3,(#38612,#38613,#38614,#38615,#38616,
#38617,#38618,#38619,#38620,#38621,#38622,#38623,#38624,#38625,#38626,#38627,
#38628,#38629,#38630,#38631,#38632,#38633,#38634,#38635,#38636,#38637,#38638,
#38639,#38640,#38641,#38642,#38643,#38644,#38645,#38646,#38647,#38648,#38649,
#38650,#38651,#38652,#38653,#38654,#38655,#38656,#38657,#38658,#38659,#38660,
#38661,#38662,#38663,#38664,#38665,#38666),.UNSPECIFIED.,.F.,.F.,(4,3,3,
3,3,3,3,3,3,3,3,3,3,3,3,3,3,3,4),(0.,0.0454718630240152,0.0931953780618431,
0.144039899826263,0.200168007591155,0.270586701894521,0.345292422602525,
0.401891619293991,0.452964632778209,0.503347839957264,0.552485563146028,
0.605298848841166,0.665634056699999,0.749225542524999,0.811919156893749,
0.864445081091848,0.913828865901365,0.959856605634592,1.),.UNSPECIFIED.);
#10999=B_SPLINE_CURVE_WITH_KNOTS('',3,(#38668,#38669,#38670,#38671),
 .UNSPECIFIED.,.F.,.F.,(4,4),(0.,1.),.UNSPECIFIED.);
#11000=B_SPLINE_CURVE_WITH_KNOTS('',3,(#38673,#38674,#38675,#38676,#38677,
#38678,#38679,#38680,#38681,#38682,#38683,#38684,#38685,#38686,#38687,#38688,
#38689,#38690,#38691,#38692,#38693,#38694,#38695,#38696,#38697,#38698,#38699,
#38700,#38701,#38702,#38703,#38704,#38705,#38706,#38707,#38708,#38709,#38710,
#38711,#38712,#38713,#38714,#38715,#38716,#38717,#38718,#38719,#38720,#38721,
#38722,#38723,#38724,#38725,#38726,#38727),.UNSPECIFIED.,.F.,.F.,(4,3,3,
3,3,3,3,3,3,3,3,3,3,3,3,3,3,3,4),(0.,0.0454743571758764,0.0932006890496627,
0.144048574957221,0.200181673047881,0.270614812390671,0.345307027643352,
0.401906381576288,0.452980318796474,0.503379519506409,0.552517196305072,
0.605331277143381,0.665671120969662,0.749253340727247,0.811940005545435,
0.864461351673187,0.913841478931383,0.959866376897951,1.),.UNSPECIFIED.);
#11001=B_SPLINE_CURVE_WITH_KNOTS('',3,(#38754,#38755,#38756,#38757,#38758,
#38759),.UNSPECIFIED.,.F.,.F.,(4,1,1,4),(-1.75610615531806,-1.00348923161032,
-0.501744615805159,2.22044604925036E-16),.UNSPECIFIED.);
#11002=B_SPLINE_CURVE_WITH_KNOTS('',3,(#38762,#38763,#38764,#38765,#38766,
#38767),.UNSPECIFIED.,.F.,.F.,(4,1,1,4),(-2.22044604925036E-16,0.501744615805159,
1.00348923161032,1.75610615531806),.UNSPECIFIED.);
#11003=B_SPLINE_CURVE_WITH_KNOTS('',3,(#38790,#38791,#38792,#38793,#38794,
#38795,#38796),.UNSPECIFIED.,.F.,.F.,(4,1,1,1,4),(-1.75610615531806,-1.2543615395129,
-0.752616923707738,-0.501744615805159,4.16333634234434E-16),
 .UNSPECIFIED.);
#11004=B_SPLINE_CURVE_WITH_KNOTS('',3,(#38797,#38798,#38799,#38800,#38801,
#38802,#38803,#38804,#38805,#38806,#38807,#38808,#38809,#38810,#38811,#38812,
#38813,#38814,#38815,#38816,#38817,#38818,#38819,#38820,#38821,#38822,#38823,
#38824,#38825,#38826,#38827,#38828,#38829,#38830,#38831,#38832,#38833,#38834,
#38835,#38836,#38837,#38838,#38839,#38840,#38841,#38842,#38843,#38844,#38845,
#38846,#38847,#38848,#38849,#38850,#38851),.UNSPECIFIED.,.F.,.F.,(4,3,3,
3,3,3,3,3,3,3,3,3,3,3,3,3,3,3,4),(0.,0.0454718630244078,0.093195378062645,
0.144039899827185,0.200168007593219,0.270586701897487,0.345292422601172,
0.401891619293172,0.452964632777252,0.503347839955838,0.552485563143815,
0.605298848838466,0.665634056695191,0.749225542521393,0.811919156891045,
0.864445081089156,0.913828865898862,0.959856605632137,1.),.UNSPECIFIED.);
#11005=B_SPLINE_CURVE_WITH_KNOTS('',3,(#38881,#38882,#38883,#38884),
 .UNSPECIFIED.,.F.,.F.,(4,4),(0.,1.),.UNSPECIFIED.);
#11006=B_SPLINE_CURVE_WITH_KNOTS('',3,(#38885,#38886,#38887,#38888,#38889,
#38890,#38891,#38892,#38893,#38894,#38895,#38896,#38897,#38898,#38899,#38900,
#38901,#38902,#38903,#38904,#38905,#38906,#38907,#38908,#38909,#38910,#38911,
#38912,#38913,#38914,#38915,#38916,#38917,#38918,#38919,#38920,#38921,#38922,
#38923,#38924,#38925,#38926,#38927,#38928,#38929,#38930,#38931,#38932,#38933,
#38934,#38935,#38936,#38937,#38938,#38939),.UNSPECIFIED.,.F.,.F.,(4,3,3,
3,3,3,3,3,3,3,3,3,3,3,3,3,3,3,4),(0.,0.0454743571757827,0.0932006890496455,
0.144048574957222,0.200181673048135,0.270614812391146,0.345307027643342,
0.401906381576231,0.452980318796516,0.503379519506306,0.552517196304985,
0.60533127714324,0.665671120969617,0.749253340727213,0.81194000554541,0.86446135167315,
0.913841478931319,0.959866376897937,1.),.UNSPECIFIED.);
#11007=B_SPLINE_CURVE_WITH_KNOTS('',3,(#38970,#38971,#38972,#38973,#38974,
#38975,#38976),.UNSPECIFIED.,.F.,.F.,(4,1,1,1,4),(-4.16333634234434E-16,
0.501744615805159,0.752616923707738,1.2543615395129,1.75610615531806),
 .UNSPECIFIED.);
#11008=B_SPLINE_CURVE_WITH_KNOTS('',3,(#38984,#38985,#38986,#38987,#38988,
#38989,#38990,#38991,#38992,#38993),.UNSPECIFIED.,.F.,.F.,(4,2,2,2,4),(-0.226321012475095,
-0.169664342772315,-0.113007673069535,-0.0565038365347675,0.),
 .UNSPECIFIED.);
#11009=B_SPLINE_CURVE_WITH_KNOTS('',3,(#39024,#39025,#39026,#39027,#39028,
#39029,#39030,#39031,#39032,#39033,#39034,#39035,#39036,#39037,#39038,#39039,
#39040,#39041,#39042,#39043,#39044,#39045,#39046,#39047,#39048,#39049,#39050,
#39051,#39052,#39053,#39054,#39055,#39056,#39057,#39058,#39059,#39060,#39061,
#39062,#39063,#39064,#39065,#39066,#39067,#39068,#39069,#39070,#39071,#39072,
#39073,#39074,#39075,#39076,#39077,#39078),.UNSPECIFIED.,.F.,.F.,(4,3,3,
3,3,3,3,3,3,3,3,3,3,3,3,3,3,3,4),(0.,0.0454718630245446,0.0931953780629266,
0.144039899826871,0.200168007592049,0.270586701894404,0.345292422600176,
0.401891619292783,0.452964632776678,0.503347839955005,0.552485563142855,
0.605298848838406,0.665634056694974,0.749225542521231,0.811919156890923,
0.864445081089191,0.913828865898807,0.959856605631954,1.),.UNSPECIFIED.);
#11010=B_SPLINE_CURVE_WITH_KNOTS('',3,(#39080,#39081,#39082,#39083),
 .UNSPECIFIED.,.F.,.F.,(4,4),(0.,1.),.UNSPECIFIED.);
#11011=B_SPLINE_CURVE_WITH_KNOTS('',3,(#39085,#39086,#39087,#39088,#39089,
#39090,#39091,#39092,#39093,#39094,#39095,#39096,#39097,#39098,#39099,#39100,
#39101,#39102,#39103,#39104,#39105,#39106,#39107,#39108,#39109,#39110,#39111,
#39112,#39113,#39114,#39115,#39116,#39117,#39118,#39119,#39120,#39121,#39122,
#39123,#39124,#39125,#39126,#39127,#39128,#39129,#39130,#39131,#39132,#39133,
#39134,#39135,#39136,#39137,#39138,#39139),.UNSPECIFIED.,.F.,.F.,(4,3,3,
3,3,3,3,3,3,3,3,3,3,3,3,3,3,3,4),(0.,0.0454743571758869,0.0932006890496471,
0.144048574957122,0.200181673047726,0.270614812390508,0.345307027643179,
0.401906381576174,0.452980318796373,0.50337951950626,0.55251719630495,0.605331277143244,
0.665671120969541,0.749253340727156,0.811940005545367,0.864461351673143,
0.913841478931369,0.959866376897944,1.),.UNSPECIFIED.);
#11012=B_SPLINE_CURVE_WITH_KNOTS('',3,(#39166,#39167,#39168,#39169,#39170,
#39171),.UNSPECIFIED.,.F.,.F.,(4,1,1,4),(-1.75610615531806,-1.00348923161032,
-0.501744615805159,2.77555756156289E-17),.UNSPECIFIED.);
#11013=B_SPLINE_CURVE_WITH_KNOTS('',3,(#39174,#39175,#39176,#39177,#39178,
#39179),.UNSPECIFIED.,.F.,.F.,(4,1,1,4),(-2.77555756156289E-17,0.501744615805159,
1.00348923161032,1.75610615531806),.UNSPECIFIED.);
#11014=B_SPLINE_CURVE_WITH_KNOTS('',3,(#39228,#39229,#39230,#39231,#39232,
#39233,#39234,#39235,#39236,#39237,#39238,#39239,#39240,#39241,#39242,#39243,
#39244,#39245,#39246,#39247,#39248,#39249,#39250,#39251,#39252,#39253,#39254,
#39255,#39256,#39257,#39258,#39259,#39260,#39261,#39262,#39263,#39264,#39265,
#39266,#39267,#39268,#39269,#39270,#39271,#39272,#39273,#39274,#39275,#39276,
#39277,#39278,#39279,#39280,#39281,#39282),.UNSPECIFIED.,.F.,.F.,(4,3,3,
3,3,3,3,3,3,3,3,3,3,3,3,3,3,3,4),(0.,0.0454718630245446,0.0931953780629266,
0.144039899826871,0.200168007592049,0.270586701894404,0.345292422600176,
0.401891619292783,0.452964632776678,0.503347839955005,0.552485563142855,
0.605298848838406,0.665634056694974,0.749225542521231,0.811919156890923,
0.864445081089191,0.913828865898807,0.959856605631954,1.),.UNSPECIFIED.);
#11015=B_SPLINE_CURVE_WITH_KNOTS('',3,(#39284,#39285,#39286,#39287),
 .UNSPECIFIED.,.F.,.F.,(4,4),(0.,1.),.UNSPECIFIED.);
#11016=B_SPLINE_CURVE_WITH_KNOTS('',3,(#39289,#39290,#39291,#39292,#39293,
#39294,#39295,#39296,#39297,#39298,#39299,#39300,#39301,#39302,#39303,#39304,
#39305,#39306,#39307,#39308,#39309,#39310,#39311,#39312,#39313,#39314,#39315,
#39316,#39317,#39318,#39319,#39320,#39321,#39322,#39323,#39324,#39325,#39326,
#39327,#39328,#39329,#39330,#39331,#39332,#39333,#39334,#39335,#39336,#39337,
#39338,#39339,#39340,#39341,#39342,#39343),.UNSPECIFIED.,.F.,.F.,(4,3,3,
3,3,3,3,3,3,3,3,3,3,3,3,3,3,3,4),(0.,0.0454743571758869,0.0932006890496471,
0.144048574957122,0.200181673047726,0.270614812390508,0.345307027643179,
0.401906381576174,0.452980318796373,0.50337951950626,0.55251719630495,0.605331277143244,
0.665671120969541,0.749253340727156,0.811940005545367,0.864461351673143,
0.913841478931369,0.959866376897944,1.),.UNSPECIFIED.);
#11017=B_SPLINE_CURVE_WITH_KNOTS('',3,(#39370,#39371,#39372,#39373,#39374,
#39375),.UNSPECIFIED.,.F.,.F.,(4,1,1,4),(-1.75610615531806,-1.00348923161032,
-0.501744615805159,2.77555756156289E-17),.UNSPECIFIED.);
#11018=B_SPLINE_CURVE_WITH_KNOTS('',3,(#39378,#39379,#39380,#39381,#39382,
#39383),.UNSPECIFIED.,.F.,.F.,(4,1,1,4),(-2.77555756156289E-17,0.501744615805159,
1.00348923161032,1.75610615531806),.UNSPECIFIED.);
#11019=B_SPLINE_CURVE_WITH_KNOTS('',3,(#39404,#39405,#39406,#39407,#39408,
#39409),.UNSPECIFIED.,.F.,.F.,(4,1,1,4),(-1.75610615531806,-1.00348923161032,
-0.501744615805159,1.27116549159798E-31),.UNSPECIFIED.);
#11020=B_SPLINE_CURVE_WITH_KNOTS('',3,(#39410,#39411,#39412,#39413,#39414,
#39415,#39416,#39417,#39418,#39419,#39420,#39421,#39422,#39423,#39424,#39425,
#39426,#39427,#39428,#39429,#39430,#39431,#39432,#39433,#39434,#39435,#39436,
#39437,#39438,#39439,#39440,#39441,#39442,#39443,#39444,#39445,#39446,#39447,
#39448,#39449,#39450,#39451,#39452,#39453,#39454,#39455,#39456,#39457,#39458,
#39459,#39460,#39461,#39462,#39463,#39464),.UNSPECIFIED.,.F.,.F.,(4,3,3,
3,3,3,3,3,3,3,3,3,3,3,3,3,3,3,4),(0.,0.0454718630242959,0.0931953780625046,
0.144039899827041,0.200168007592975,0.270586701897097,0.345292422601312,
0.401891619293206,0.452964632777226,0.503347839955808,0.552485563143695,
0.60529884883852,0.665634056695758,0.749225542521819,0.811919156891364,
0.864445081089579,0.913828865899227,0.959856605632539,1.),.UNSPECIFIED.);
#11021=B_SPLINE_CURVE_WITH_KNOTS('',3,(#39494,#39495,#39496,#39497),
 .UNSPECIFIED.,.F.,.F.,(4,4),(0.,1.),.UNSPECIFIED.);
#11022=B_SPLINE_CURVE_WITH_KNOTS('',3,(#39498,#39499,#39500,#39501,#39502,
#39503,#39504,#39505,#39506,#39507,#39508,#39509,#39510,#39511,#39512,#39513,
#39514,#39515,#39516,#39517,#39518,#39519,#39520,#39521,#39522,#39523,#39524,
#39525,#39526,#39527,#39528,#39529,#39530,#39531,#39532,#39533,#39534,#39535,
#39536,#39537,#39538,#39539,#39540,#39541,#39542,#39543,#39544,#39545,#39546,
#39547,#39548,#39549,#39550,#39551,#39552),.UNSPECIFIED.,.F.,.F.,(4,3,3,
3,3,3,3,3,3,3,3,3,3,3,3,3,3,3,4),(0.,0.0454743571758223,0.0932006890496185,
0.144048574957236,0.200181673047968,0.270614812390343,0.34530702764307,
0.401906381576014,0.452980318796357,0.503379519506187,0.552517196304828,
0.605331277143297,0.665671120969503,0.749253340727127,0.811940005545345,
0.864461351673149,0.913841478931467,0.959866376898016,1.),.UNSPECIFIED.);
#11023=B_SPLINE_CURVE_WITH_KNOTS('',3,(#39579,#39580,#39581,#39582,#39583,
#39584),.UNSPECIFIED.,.F.,.F.,(4,1,1,4),(-1.27116549159798E-31,0.501744615805159,
1.00348923161032,1.75610615531806),.UNSPECIFIED.);
#11024=B_SPLINE_CURVE_WITH_KNOTS('',3,(#39592,#39593,#39594,#39595,#39596,
#39597,#39598,#39599,#39600,#39601),.UNSPECIFIED.,.F.,.F.,(4,2,2,2,4),(-0.226321012475095,
-0.169664342772315,-0.113007673069535,-0.0565038365347675,0.),
 .UNSPECIFIED.);
#11025=B_SPLINE_CURVE_WITH_KNOTS('',3,(#39632,#39633,#39634,#39635,#39636,
#39637,#39638,#39639,#39640,#39641,#39642,#39643,#39644,#39645,#39646,#39647,
#39648,#39649,#39650,#39651,#39652,#39653,#39654,#39655,#39656,#39657,#39658,
#39659,#39660,#39661,#39662,#39663,#39664,#39665,#39666,#39667,#39668,#39669,
#39670,#39671,#39672,#39673,#39674,#39675,#39676,#39677,#39678,#39679,#39680,
#39681,#39682,#39683,#39684,#39685,#39686),.UNSPECIFIED.,.F.,.F.,(4,3,3,
3,3,3,3,3,3,3,3,3,3,3,3,3,3,3,4),(0.,0.045471863024028,0.0931953780617352,
0.144039899826522,0.200168007592056,0.270586701896401,0.345292422600315,
0.401891619292387,0.452964632776744,0.503347839957351,0.552485563145081,
0.605298848840994,0.665634056697722,0.749225542523292,0.811919156892469,
0.864445081090302,0.913828865899915,0.959856605633197,1.),.UNSPECIFIED.);
#11026=B_SPLINE_CURVE_WITH_KNOTS('',3,(#39688,#39689,#39690,#39691),
 .UNSPECIFIED.,.F.,.F.,(4,4),(0.,1.),.UNSPECIFIED.);
#11027=B_SPLINE_CURVE_WITH_KNOTS('',3,(#39693,#39694,#39695,#39696,#39697,
#39698,#39699,#39700,#39701,#39702,#39703,#39704,#39705,#39706,#39707,#39708,
#39709,#39710,#39711,#39712,#39713,#39714,#39715,#39716,#39717,#39718,#39719,
#39720,#39721,#39722,#39723,#39724,#39725,#39726,#39727,#39728,#39729,#39730,
#39731,#39732,#39733,#39734,#39735,#39736,#39737,#39738,#39739,#39740,#39741,
#39742,#39743,#39744,#39745,#39746,#39747),.UNSPECIFIED.,.F.,.F.,(4,3,3,
3,3,3,3,3,3,3,3,3,3,3,3,3,3,3,4),(0.,0.0454743571758992,0.0932006890496849,
0.144048574957235,0.200181673047928,0.270614812390673,0.345307027643151,
0.401906381576126,0.452980318796356,0.503379519506263,0.552517196304882,
0.605331277143196,0.665671120969352,0.749253340727014,0.811940005545261,
0.864461351673037,0.913841478931272,0.959866376897846,1.),.UNSPECIFIED.);
#11028=B_SPLINE_CURVE_WITH_KNOTS('',3,(#39778,#39779,#39780,#39781,#39782,
#39783,#39784),.UNSPECIFIED.,.F.,.F.,(4,1,1,1,4),(-1.75610615531805,-1.25436153951289,
-0.752616923707736,-0.501744615805158,1.11022302462516E-16),
 .UNSPECIFIED.);
#11029=B_SPLINE_CURVE_WITH_KNOTS('',3,(#39787,#39788,#39789,#39790,#39791,
#39792,#39793),.UNSPECIFIED.,.F.,.F.,(4,1,1,1,4),(-1.11022302462516E-16,
0.501744615805158,0.752616923707736,1.25436153951289,1.75610615531805),
 .UNSPECIFIED.);
#11030=B_SPLINE_CURVE_WITH_KNOTS('',3,(#39814,#39815,#39816,#39817,#39818,
#39819,#39820),.UNSPECIFIED.,.F.,.F.,(4,1,1,1,4),(-1.75610615531806,-1.2543615395129,
-0.752616923707739,-0.501744615805159,4.10679309198325E-32),
 .UNSPECIFIED.);
#11031=B_SPLINE_CURVE_WITH_KNOTS('',3,(#39821,#39822,#39823,#39824,#39825,
#39826,#39827,#39828,#39829,#39830,#39831,#39832,#39833,#39834,#39835,#39836,
#39837,#39838,#39839,#39840,#39841,#39842,#39843,#39844,#39845,#39846,#39847,
#39848,#39849,#39850,#39851,#39852,#39853,#39854,#39855,#39856,#39857,#39858,
#39859,#39860,#39861,#39862,#39863,#39864,#39865,#39866,#39867,#39868,#39869,
#39870,#39871,#39872,#39873,#39874,#39875),.UNSPECIFIED.,.F.,.F.,(4,3,3,
3,3,3,3,3,3,3,3,3,3,3,3,3,3,3,4),(0.,0.0454718630243362,0.0931953780625649,
0.144039899826463,0.200168007592413,0.27058670189605,0.345292422599966,
0.401891619292168,0.452964632776254,0.503347839954095,0.552485563141883,
0.605298848836136,0.665634056692691,0.749225542519518,0.811919156889639,
0.864445081087949,0.913828865897587,0.959856605630922,1.),.UNSPECIFIED.);
#11032=B_SPLINE_CURVE_WITH_KNOTS('',3,(#39905,#39906,#39907,#39908),
 .UNSPECIFIED.,.F.,.F.,(4,4),(0.,1.),.UNSPECIFIED.);
#11033=B_SPLINE_CURVE_WITH_KNOTS('',3,(#39909,#39910,#39911,#39912,#39913,
#39914,#39915,#39916,#39917,#39918,#39919,#39920,#39921,#39922,#39923,#39924,
#39925,#39926,#39927,#39928,#39929,#39930,#39931,#39932,#39933,#39934,#39935,
#39936,#39937,#39938,#39939,#39940,#39941,#39942,#39943,#39944,#39945,#39946,
#39947,#39948,#39949,#39950,#39951,#39952,#39953,#39954,#39955,#39956,#39957,
#39958,#39959,#39960,#39961,#39962,#39963),.UNSPECIFIED.,.F.,.F.,(4,3,3,
3,3,3,3,3,3,3,3,3,3,3,3,3,3,3,4),(0.,0.0454743571757403,0.0932006890494696,
0.144048574956973,0.200181673047506,0.270614812390275,0.345307027643286,
0.401906381576242,0.452980318796464,0.503379519506601,0.552517196305261,
0.605331277143663,0.665671120969907,0.74925334072743,0.811940005545573,
0.864461351673319,0.91384147893155,0.95986637689812,1.),.UNSPECIFIED.);
#11034=B_SPLINE_CURVE_WITH_KNOTS('',3,(#39994,#39995,#39996,#39997,#39998,
#39999,#40000),.UNSPECIFIED.,.F.,.F.,(4,1,1,1,4),(-4.10679309198325E-32,
0.501744615805159,0.752616923707739,1.2543615395129,1.75610615531806),
 .UNSPECIFIED.);
#11035=B_SPLINE_CURVE_WITH_KNOTS('',3,(#40008,#40009,#40010,#40011,#40012,
#40013,#40014,#40015,#40016,#40017),.UNSPECIFIED.,.F.,.F.,(4,2,2,2,4),(-0.226321012475095,
-0.169664342772315,-0.113007673069535,-0.0565038365347676,0.),
 .UNSPECIFIED.);
#11036=B_SPLINE_CURVE_WITH_KNOTS('',3,(#40075,#40076,#40077,#40078,#40079,
#40080,#40081,#40082,#40083,#40084),.UNSPECIFIED.,.F.,.F.,(4,2,2,2,4),(0.,
0.0565038365347675,0.113007673069535,0.169664342772315,0.226321012475095),
 .UNSPECIFIED.);
#11037=B_SPLINE_CURVE_WITH_KNOTS('',3,(#40090,#40091,#40092,#40093,#40094,
#40095,#40096,#40097,#40098,#40099),.UNSPECIFIED.,.F.,.F.,(4,2,2,2,4),(0.,
0.0565038365347674,0.113007673069535,0.169664342772315,0.226321012475095),
 .UNSPECIFIED.);
#11038=B_SPLINE_CURVE_WITH_KNOTS('',2,(#40171,#40172,#40173),
 .UNSPECIFIED.,.F.,.F.,(3,3),(0.,1.),.UNSPECIFIED.);
#11039=B_SPLINE_CURVE_WITH_KNOTS('',2,(#40175,#40176,#40177),
 .UNSPECIFIED.,.F.,.F.,(3,3),(0.,1.),.UNSPECIFIED.);
#11040=B_SPLINE_CURVE_WITH_KNOTS('',2,(#40179,#40180,#40181),
 .UNSPECIFIED.,.F.,.F.,(3,3),(0.,1.),.UNSPECIFIED.);
#11041=B_SPLINE_CURVE_WITH_KNOTS('',2,(#40185,#40186,#40187),
 .UNSPECIFIED.,.F.,.F.,(3,3),(0.,1.),.UNSPECIFIED.);
#11042=B_SPLINE_CURVE_WITH_KNOTS('',2,(#40189,#40190,#40191),
 .UNSPECIFIED.,.F.,.F.,(3,3),(0.,1.),.UNSPECIFIED.);
#11043=B_SPLINE_CURVE_WITH_KNOTS('',2,(#40193,#40194,#40195),
 .UNSPECIFIED.,.F.,.F.,(3,3),(0.,1.),.UNSPECIFIED.);
#11044=B_SPLINE_CURVE_WITH_KNOTS('',2,(#40197,#40198,#40199),
 .UNSPECIFIED.,.F.,.F.,(3,3),(0.,1.),.UNSPECIFIED.);
#11045=B_SPLINE_CURVE_WITH_KNOTS('',2,(#40201,#40202,#40203),
 .UNSPECIFIED.,.F.,.F.,(3,3),(0.,1.),.UNSPECIFIED.);
#11046=B_SPLINE_CURVE_WITH_KNOTS('',2,(#40205,#40206,#40207),
 .UNSPECIFIED.,.F.,.F.,(3,3),(0.,1.),.UNSPECIFIED.);
#11047=B_SPLINE_CURVE_WITH_KNOTS('',2,(#40209,#40210,#40211),
 .UNSPECIFIED.,.F.,.F.,(3,3),(0.,1.),.UNSPECIFIED.);
#11048=B_SPLINE_CURVE_WITH_KNOTS('',2,(#40213,#40214,#40215),
 .UNSPECIFIED.,.F.,.F.,(3,3),(0.,1.),.UNSPECIFIED.);
#11049=B_SPLINE_CURVE_WITH_KNOTS('',2,(#40217,#40218,#40219),
 .UNSPECIFIED.,.F.,.F.,(3,3),(0.,1.),.UNSPECIFIED.);
#11050=B_SPLINE_CURVE_WITH_KNOTS('',2,(#40221,#40222,#40223),
 .UNSPECIFIED.,.F.,.F.,(3,3),(0.,1.),.UNSPECIFIED.);
#11051=B_SPLINE_CURVE_WITH_KNOTS('',2,(#40225,#40226,#40227),
 .UNSPECIFIED.,.F.,.F.,(3,3),(0.,1.),.UNSPECIFIED.);
#11052=B_SPLINE_CURVE_WITH_KNOTS('',2,(#40229,#40230,#40231),
 .UNSPECIFIED.,.F.,.F.,(3,3),(0.,1.),.UNSPECIFIED.);
#11053=B_SPLINE_CURVE_WITH_KNOTS('',2,(#40233,#40234,#40235),
 .UNSPECIFIED.,.F.,.F.,(3,3),(0.,1.),.UNSPECIFIED.);
#11054=B_SPLINE_CURVE_WITH_KNOTS('',2,(#40237,#40238,#40239),
 .UNSPECIFIED.,.F.,.F.,(3,3),(0.,1.),.UNSPECIFIED.);
#11055=B_SPLINE_CURVE_WITH_KNOTS('',2,(#40241,#40242,#40243),
 .UNSPECIFIED.,.F.,.F.,(3,3),(0.,1.),.UNSPECIFIED.);
#11056=B_SPLINE_CURVE_WITH_KNOTS('',2,(#40245,#40246,#40247),
 .UNSPECIFIED.,.F.,.F.,(3,3),(0.,1.),.UNSPECIFIED.);
#11057=B_SPLINE_CURVE_WITH_KNOTS('',2,(#40249,#40250,#40251),
 .UNSPECIFIED.,.F.,.F.,(3,3),(0.,1.),.UNSPECIFIED.);
#11058=B_SPLINE_CURVE_WITH_KNOTS('',2,(#40253,#40254,#40255),
 .UNSPECIFIED.,.F.,.F.,(3,3),(0.,1.),.UNSPECIFIED.);
#11059=B_SPLINE_CURVE_WITH_KNOTS('',2,(#40259,#40260,#40261),
 .UNSPECIFIED.,.F.,.F.,(3,3),(0.,1.),.UNSPECIFIED.);
#11060=B_SPLINE_CURVE_WITH_KNOTS('',2,(#40263,#40264,#40265),
 .UNSPECIFIED.,.F.,.F.,(3,3),(0.,1.),.UNSPECIFIED.);
#11061=B_SPLINE_CURVE_WITH_KNOTS('',2,(#40267,#40268,#40269),
 .UNSPECIFIED.,.F.,.F.,(3,3),(0.,1.),.UNSPECIFIED.);
#11062=B_SPLINE_CURVE_WITH_KNOTS('',2,(#40271,#40272,#40273),
 .UNSPECIFIED.,.F.,.F.,(3,3),(0.,1.),.UNSPECIFIED.);
#11063=B_SPLINE_CURVE_WITH_KNOTS('',2,(#40275,#40276,#40277),
 .UNSPECIFIED.,.F.,.F.,(3,3),(0.,1.),.UNSPECIFIED.);
#11064=B_SPLINE_CURVE_WITH_KNOTS('',2,(#40279,#40280,#40281),
 .UNSPECIFIED.,.F.,.F.,(3,3),(0.,1.),.UNSPECIFIED.);
#11065=B_SPLINE_CURVE_WITH_KNOTS('',2,(#40283,#40284,#40285),
 .UNSPECIFIED.,.F.,.F.,(3,3),(0.,1.),.UNSPECIFIED.);
#11066=B_SPLINE_CURVE_WITH_KNOTS('',2,(#40287,#40288,#40289),
 .UNSPECIFIED.,.F.,.F.,(3,3),(0.,1.),.UNSPECIFIED.);
#11067=B_SPLINE_CURVE_WITH_KNOTS('',2,(#40291,#40292,#40293),
 .UNSPECIFIED.,.F.,.F.,(3,3),(0.,1.),.UNSPECIFIED.);
#11068=B_SPLINE_CURVE_WITH_KNOTS('',2,(#40295,#40296,#40297),
 .UNSPECIFIED.,.F.,.F.,(3,3),(0.,1.),.UNSPECIFIED.);
#11069=B_SPLINE_CURVE_WITH_KNOTS('',2,(#40299,#40300,#40301),
 .UNSPECIFIED.,.F.,.F.,(3,3),(0.,1.),.UNSPECIFIED.);
#11070=B_SPLINE_CURVE_WITH_KNOTS('',2,(#40302,#40303,#40304),
 .UNSPECIFIED.,.F.,.F.,(3,3),(0.,1.),.UNSPECIFIED.);
#11071=B_SPLINE_CURVE_WITH_KNOTS('',2,(#40321,#40322,#40323),
 .UNSPECIFIED.,.F.,.F.,(3,3),(0.,1.),.UNSPECIFIED.);
#11072=B_SPLINE_CURVE_WITH_KNOTS('',2,(#40325,#40326,#40327),
 .UNSPECIFIED.,.F.,.F.,(3,3),(0.,1.),.UNSPECIFIED.);
#11073=B_SPLINE_CURVE_WITH_KNOTS('',2,(#40359,#40360,#40361),
 .UNSPECIFIED.,.F.,.F.,(3,3),(0.,1.),.UNSPECIFIED.);
#11074=B_SPLINE_CURVE_WITH_KNOTS('',2,(#40363,#40364,#40365),
 .UNSPECIFIED.,.F.,.F.,(3,3),(0.,1.),.UNSPECIFIED.);
#11075=B_SPLINE_CURVE_WITH_KNOTS('',2,(#40367,#40368,#40369),
 .UNSPECIFIED.,.F.,.F.,(3,3),(0.,1.),.UNSPECIFIED.);
#11076=B_SPLINE_CURVE_WITH_KNOTS('',2,(#40371,#40372,#40373),
 .UNSPECIFIED.,.F.,.F.,(3,3),(0.,1.),.UNSPECIFIED.);
#11077=B_SPLINE_CURVE_WITH_KNOTS('',2,(#40375,#40376,#40377),
 .UNSPECIFIED.,.F.,.F.,(3,3),(0.,1.),.UNSPECIFIED.);
#11078=B_SPLINE_CURVE_WITH_KNOTS('',2,(#40379,#40380,#40381),
 .UNSPECIFIED.,.F.,.F.,(3,3),(0.,1.),.UNSPECIFIED.);
#11079=B_SPLINE_CURVE_WITH_KNOTS('',2,(#40383,#40384,#40385),
 .UNSPECIFIED.,.F.,.F.,(3,3),(0.,1.),.UNSPECIFIED.);
#11080=B_SPLINE_CURVE_WITH_KNOTS('',2,(#40387,#40388,#40389),
 .UNSPECIFIED.,.F.,.F.,(3,3),(0.,1.),.UNSPECIFIED.);
#11081=B_SPLINE_CURVE_WITH_KNOTS('',2,(#40391,#40392,#40393),
 .UNSPECIFIED.,.F.,.F.,(3,3),(0.,1.),.UNSPECIFIED.);
#11082=B_SPLINE_CURVE_WITH_KNOTS('',2,(#40395,#40396,#40397),
 .UNSPECIFIED.,.F.,.F.,(3,3),(0.,1.),.UNSPECIFIED.);
#11083=B_SPLINE_CURVE_WITH_KNOTS('',2,(#40399,#40400,#40401),
 .UNSPECIFIED.,.F.,.F.,(3,3),(0.,1.),.UNSPECIFIED.);
#11084=B_SPLINE_CURVE_WITH_KNOTS('',2,(#40409,#40410,#40411),
 .UNSPECIFIED.,.F.,.F.,(3,3),(0.,1.),.UNSPECIFIED.);
#11085=B_SPLINE_CURVE_WITH_KNOTS('',2,(#40413,#40414,#40415),
 .UNSPECIFIED.,.F.,.F.,(3,3),(0.,1.),.UNSPECIFIED.);
#11086=B_SPLINE_CURVE_WITH_KNOTS('',2,(#40417,#40418,#40419),
 .UNSPECIFIED.,.F.,.F.,(3,3),(0.,1.),.UNSPECIFIED.);
#11087=B_SPLINE_CURVE_WITH_KNOTS('',2,(#40421,#40422,#40423),
 .UNSPECIFIED.,.F.,.F.,(3,3),(0.,1.),.UNSPECIFIED.);
#11088=B_SPLINE_CURVE_WITH_KNOTS('',2,(#40425,#40426,#40427),
 .UNSPECIFIED.,.F.,.F.,(3,3),(0.,1.),.UNSPECIFIED.);
#11089=B_SPLINE_CURVE_WITH_KNOTS('',2,(#40429,#40430,#40431),
 .UNSPECIFIED.,.F.,.F.,(3,3),(0.,1.),.UNSPECIFIED.);
#11090=B_SPLINE_CURVE_WITH_KNOTS('',2,(#40433,#40434,#40435),
 .UNSPECIFIED.,.F.,.F.,(3,3),(0.,1.),.UNSPECIFIED.);
#11091=B_SPLINE_CURVE_WITH_KNOTS('',2,(#40457,#40458,#40459),
 .UNSPECIFIED.,.F.,.F.,(3,3),(0.,1.),.UNSPECIFIED.);
#11092=B_SPLINE_CURVE_WITH_KNOTS('',2,(#40461,#40462,#40463),
 .UNSPECIFIED.,.F.,.F.,(3,3),(0.,1.),.UNSPECIFIED.);
#11093=B_SPLINE_CURVE_WITH_KNOTS('',2,(#40465,#40466,#40467),
 .UNSPECIFIED.,.F.,.F.,(3,3),(0.,1.),.UNSPECIFIED.);
#11094=B_SPLINE_CURVE_WITH_KNOTS('',2,(#40469,#40470,#40471),
 .UNSPECIFIED.,.F.,.F.,(3,3),(0.,1.),.UNSPECIFIED.);
#11095=B_SPLINE_CURVE_WITH_KNOTS('',3,(#40481,#40482,#40483,#40484,#40485,
#40486,#40487,#40488,#40489,#40490),.UNSPECIFIED.,.F.,.F.,(4,2,2,2,4),(0.,
0.0565038365347674,0.113007673069535,0.169664342772315,0.226321012475095),
 .UNSPECIFIED.);
#11096=B_SPLINE_CURVE_WITH_KNOTS('',3,(#40501,#40502,#40503,#40504,#40505,
#40506,#40507,#40508,#40509,#40510),.UNSPECIFIED.,.F.,.F.,(4,2,2,2,4),(-0.226321012475095,
-0.169664342772315,-0.113007673069535,-0.0565038365347675,0.),
 .UNSPECIFIED.);
#11097=B_SPLINE_CURVE_WITH_KNOTS('',3,(#40520,#40521,#40522,#40523,#40524,
#40525,#40526,#40527,#40528,#40529),.UNSPECIFIED.,.F.,.F.,(4,2,2,2,4),(0.,
0.0565038365347674,0.113007673069535,0.169664342772315,0.226321012475095),
 .UNSPECIFIED.);
#11098=B_SPLINE_CURVE_WITH_KNOTS('',3,(#40540,#40541,#40542,#40543,#40544,
#40545,#40546,#40547,#40548,#40549,#40550,#40551,#40552,#40553),
 .UNSPECIFIED.,.F.,.F.,(4,2,2,2,2,2,4),(-0.577484191975641,-0.576699234562216,
-0.508563556454706,-0.443999452377128,-0.379354331952853,-0.330847656983477,
-0.288349617279839),.UNSPECIFIED.);
#11099=B_SPLINE_CURVE_WITH_KNOTS('',3,(#40556,#40557,#40558,#40559,#40560,
#40561,#40562,#40563,#40564,#40565,#40566,#40567,#40568,#40569),
 .UNSPECIFIED.,.F.,.F.,(4,2,2,2,2,2,4),(-0.288349617199946,-0.245851577508476,
-0.19734490255298,-0.132699782147205,-0.0681356780881004,0.,0.000784957413179436),
 .UNSPECIFIED.);
#11100=B_SPLINE_CURVE_WITH_KNOTS('',3,(#40574,#40575,#40576,#40577,#40578,
#40579,#40580,#40581,#40582,#40583),.UNSPECIFIED.,.F.,.F.,(4,2,2,2,4),(0.452090436017012,
0.508593613016053,0.565096790015094,0.621605199566296,0.678113609117498),
 .UNSPECIFIED.);
#11101=B_SPLINE_CURVE_WITH_KNOTS('',3,(#40589,#40590,#40591,#40592,#40593,
#40594,#40595,#40596,#40597,#40598),.UNSPECIFIED.,.F.,.F.,(4,2,2,2,4),(0.226067262916527,
0.282575672467729,0.339084082018931,0.395587259017972,0.452090436017013),
 .UNSPECIFIED.);
#11102=B_SPLINE_CURVE_WITH_KNOTS('',3,(#40620,#40621,#40622,#40623),
 .UNSPECIFIED.,.F.,.F.,(4,4),(2.49844264446827,2.64149356559396),
 .UNSPECIFIED.);
#11103=B_SPLINE_CURVE_WITH_KNOTS('',3,(#40624,#40625,#40626,#40627),
 .UNSPECIFIED.,.F.,.F.,(4,4),(2.49844264446365,2.64149356558944),
 .UNSPECIFIED.);
#11104=B_SPLINE_CURVE_WITH_KNOTS('',3,(#40628,#40629,#40630,#40631),
 .UNSPECIFIED.,.F.,.F.,(4,4),(2.49844264445768,2.64149356558346),
 .UNSPECIFIED.);
#11105=B_SPLINE_CURVE_WITH_KNOTS('',3,(#40632,#40633,#40634,#40635),
 .UNSPECIFIED.,.F.,.F.,(4,4),(2.49844264445882,2.64149356558449),
 .UNSPECIFIED.);
#11106=B_SPLINE_CURVE_WITH_KNOTS('',3,(#40636,#40637,#40638,#40639),
 .UNSPECIFIED.,.F.,.F.,(4,4),(2.49844264444559,2.64149356557132),
 .UNSPECIFIED.);
#11107=B_SPLINE_CURVE_WITH_KNOTS('',3,(#40645,#40646,#40647,#40648),
 .UNSPECIFIED.,.F.,.F.,(4,4),(2.49844264448387,2.64149356560953),
 .UNSPECIFIED.);
#11108=B_SPLINE_CURVE_WITH_KNOTS('',3,(#40649,#40650,#40651,#40652),
 .UNSPECIFIED.,.F.,.F.,(4,4),(2.49844264446318,2.64149356558896),
 .UNSPECIFIED.);
#11109=B_SPLINE_CURVE_WITH_KNOTS('',3,(#40653,#40654,#40655,#40656),
 .UNSPECIFIED.,.F.,.F.,(4,4),(2.49844264447263,2.6414935655984),
 .UNSPECIFIED.);
#11110=B_SPLINE_CURVE_WITH_KNOTS('',2,(#40779,#40780,#40781),
 .UNSPECIFIED.,.F.,.F.,(3,3),(0.,1.),.UNSPECIFIED.);
#11111=B_SPLINE_CURVE_WITH_KNOTS('',2,(#40791,#40792,#40793),
 .UNSPECIFIED.,.F.,.F.,(3,3),(0.,1.),.UNSPECIFIED.);
#11112=B_SPLINE_CURVE_WITH_KNOTS('',2,(#40802,#40803,#40804),
 .UNSPECIFIED.,.F.,.F.,(3,3),(0.,1.),.UNSPECIFIED.);
#11113=B_SPLINE_CURVE_WITH_KNOTS('',2,(#40813,#40814,#40815),
 .UNSPECIFIED.,.F.,.F.,(3,3),(0.,1.),.UNSPECIFIED.);
#11114=B_SPLINE_CURVE_WITH_KNOTS('',2,(#40824,#40825,#40826),
 .UNSPECIFIED.,.F.,.F.,(3,3),(0.,1.),.UNSPECIFIED.);
#11115=B_SPLINE_CURVE_WITH_KNOTS('',2,(#40835,#40836,#40837),
 .UNSPECIFIED.,.F.,.F.,(3,3),(0.,1.),.UNSPECIFIED.);
#11116=B_SPLINE_CURVE_WITH_KNOTS('',2,(#40846,#40847,#40848),
 .UNSPECIFIED.,.F.,.F.,(3,3),(0.,1.),.UNSPECIFIED.);
#11117=B_SPLINE_CURVE_WITH_KNOTS('',2,(#40857,#40858,#40859),
 .UNSPECIFIED.,.F.,.F.,(3,3),(0.,1.),.UNSPECIFIED.);
#11118=B_SPLINE_CURVE_WITH_KNOTS('',2,(#40868,#40869,#40870),
 .UNSPECIFIED.,.F.,.F.,(3,3),(0.,1.),.UNSPECIFIED.);
#11119=B_SPLINE_CURVE_WITH_KNOTS('',2,(#40879,#40880,#40881),
 .UNSPECIFIED.,.F.,.F.,(3,3),(0.,1.),.UNSPECIFIED.);
#11120=B_SPLINE_CURVE_WITH_KNOTS('',2,(#40894,#40895,#40896),
 .UNSPECIFIED.,.F.,.F.,(3,3),(0.,1.),.UNSPECIFIED.);
#11121=B_SPLINE_CURVE_WITH_KNOTS('',2,(#40907,#40908,#40909),
 .UNSPECIFIED.,.F.,.F.,(3,3),(0.,1.),.UNSPECIFIED.);
#11122=B_SPLINE_CURVE_WITH_KNOTS('',2,(#40919,#40920,#40921),
 .UNSPECIFIED.,.F.,.F.,(3,3),(0.,1.),.UNSPECIFIED.);
#11123=B_SPLINE_CURVE_WITH_KNOTS('',2,(#40930,#40931,#40932),
 .UNSPECIFIED.,.F.,.F.,(3,3),(0.,1.),.UNSPECIFIED.);
#11124=B_SPLINE_CURVE_WITH_KNOTS('',2,(#40941,#40942,#40943),
 .UNSPECIFIED.,.F.,.F.,(3,3),(0.,1.),.UNSPECIFIED.);
#11125=B_SPLINE_CURVE_WITH_KNOTS('',2,(#40952,#40953,#40954),
 .UNSPECIFIED.,.F.,.F.,(3,3),(0.,1.),.UNSPECIFIED.);
#11126=B_SPLINE_CURVE_WITH_KNOTS('',2,(#40963,#40964,#40965),
 .UNSPECIFIED.,.F.,.F.,(3,3),(0.,1.),.UNSPECIFIED.);
#11127=B_SPLINE_CURVE_WITH_KNOTS('',2,(#40974,#40975,#40976),
 .UNSPECIFIED.,.F.,.F.,(3,3),(0.,1.),.UNSPECIFIED.);
#11128=B_SPLINE_CURVE_WITH_KNOTS('',2,(#40985,#40986,#40987),
 .UNSPECIFIED.,.F.,.F.,(3,3),(0.,1.),.UNSPECIFIED.);
#11129=B_SPLINE_CURVE_WITH_KNOTS('',2,(#40996,#40997,#40998),
 .UNSPECIFIED.,.F.,.F.,(3,3),(0.,1.),.UNSPECIFIED.);
#11130=B_SPLINE_CURVE_WITH_KNOTS('',2,(#41007,#41008,#41009),
 .UNSPECIFIED.,.F.,.F.,(3,3),(0.,1.),.UNSPECIFIED.);
#11131=B_SPLINE_CURVE_WITH_KNOTS('',2,(#41018,#41019,#41020),
 .UNSPECIFIED.,.F.,.F.,(3,3),(0.,1.),.UNSPECIFIED.);
#11132=B_SPLINE_CURVE_WITH_KNOTS('',2,(#41029,#41030,#41031),
 .UNSPECIFIED.,.F.,.F.,(3,3),(0.,1.),.UNSPECIFIED.);
#11133=B_SPLINE_CURVE_WITH_KNOTS('',2,(#41040,#41041,#41042),
 .UNSPECIFIED.,.F.,.F.,(3,3),(0.,1.),.UNSPECIFIED.);
#11134=B_SPLINE_CURVE_WITH_KNOTS('',2,(#41055,#41056,#41057),
 .UNSPECIFIED.,.F.,.F.,(3,3),(0.,1.),.UNSPECIFIED.);
#11135=B_SPLINE_CURVE_WITH_KNOTS('',2,(#41066,#41067,#41068),
 .UNSPECIFIED.,.F.,.F.,(3,3),(0.,1.),.UNSPECIFIED.);
#11136=B_SPLINE_CURVE_WITH_KNOTS('',2,(#41077,#41078,#41079),
 .UNSPECIFIED.,.F.,.F.,(3,3),(0.,1.),.UNSPECIFIED.);
#11137=B_SPLINE_CURVE_WITH_KNOTS('',2,(#41088,#41089,#41090),
 .UNSPECIFIED.,.F.,.F.,(3,3),(0.,1.),.UNSPECIFIED.);
#11138=B_SPLINE_CURVE_WITH_KNOTS('',2,(#41099,#41100,#41101),
 .UNSPECIFIED.,.F.,.F.,(3,3),(0.,1.),.UNSPECIFIED.);
#11139=B_SPLINE_CURVE_WITH_KNOTS('',2,(#41110,#41111,#41112),
 .UNSPECIFIED.,.F.,.F.,(3,3),(0.,1.),.UNSPECIFIED.);
#11140=B_SPLINE_CURVE_WITH_KNOTS('',2,(#41121,#41122,#41123),
 .UNSPECIFIED.,.F.,.F.,(3,3),(0.,1.),.UNSPECIFIED.);
#11141=B_SPLINE_CURVE_WITH_KNOTS('',2,(#41132,#41133,#41134),
 .UNSPECIFIED.,.F.,.F.,(3,3),(0.,1.),.UNSPECIFIED.);
#11142=B_SPLINE_CURVE_WITH_KNOTS('',2,(#41143,#41144,#41145),
 .UNSPECIFIED.,.F.,.F.,(3,3),(0.,1.),.UNSPECIFIED.);
#11143=B_SPLINE_CURVE_WITH_KNOTS('',2,(#41154,#41155,#41156),
 .UNSPECIFIED.,.F.,.F.,(3,3),(0.,1.),.UNSPECIFIED.);
#11144=B_SPLINE_CURVE_WITH_KNOTS('',2,(#41165,#41166,#41167),
 .UNSPECIFIED.,.F.,.F.,(3,3),(0.,1.),.UNSPECIFIED.);
#11145=B_SPLINE_CURVE_WITH_KNOTS('',2,(#41176,#41177,#41178),
 .UNSPECIFIED.,.F.,.F.,(3,3),(0.,1.),.UNSPECIFIED.);
#11146=B_SPLINE_CURVE_WITH_KNOTS('',2,(#41187,#41188,#41189),
 .UNSPECIFIED.,.F.,.F.,(3,3),(0.,1.),.UNSPECIFIED.);
#11147=B_SPLINE_CURVE_WITH_KNOTS('',2,(#41198,#41199,#41200),
 .UNSPECIFIED.,.F.,.F.,(3,3),(0.,1.),.UNSPECIFIED.);
#11148=B_SPLINE_CURVE_WITH_KNOTS('',2,(#41209,#41210,#41211),
 .UNSPECIFIED.,.F.,.F.,(3,3),(0.,1.),.UNSPECIFIED.);
#11149=B_SPLINE_CURVE_WITH_KNOTS('',2,(#41220,#41221,#41222),
 .UNSPECIFIED.,.F.,.F.,(3,3),(0.,1.),.UNSPECIFIED.);
#11150=B_SPLINE_CURVE_WITH_KNOTS('',2,(#41231,#41232,#41233),
 .UNSPECIFIED.,.F.,.F.,(3,3),(0.,1.),.UNSPECIFIED.);
#11151=B_SPLINE_CURVE_WITH_KNOTS('',2,(#41242,#41243,#41244),
 .UNSPECIFIED.,.F.,.F.,(3,3),(0.,1.),.UNSPECIFIED.);
#11152=B_SPLINE_CURVE_WITH_KNOTS('',2,(#41257,#41258,#41259),
 .UNSPECIFIED.,.F.,.F.,(3,3),(0.,1.),.UNSPECIFIED.);
#11153=B_SPLINE_CURVE_WITH_KNOTS('',2,(#41266,#41267,#41268),
 .UNSPECIFIED.,.F.,.F.,(3,3),(0.,1.),.UNSPECIFIED.);
#11154=B_SPLINE_CURVE_WITH_KNOTS('',2,(#41284,#41285,#41286),
 .UNSPECIFIED.,.F.,.F.,(3,3),(0.,1.),.UNSPECIFIED.);
#11155=B_SPLINE_CURVE_WITH_KNOTS('',2,(#41295,#41296,#41297),
 .UNSPECIFIED.,.F.,.F.,(3,3),(0.,1.),.UNSPECIFIED.);
#11156=B_SPLINE_CURVE_WITH_KNOTS('',2,(#41306,#41307,#41308),
 .UNSPECIFIED.,.F.,.F.,(3,3),(0.,1.),.UNSPECIFIED.);
#11157=B_SPLINE_CURVE_WITH_KNOTS('',2,(#41317,#41318,#41319),
 .UNSPECIFIED.,.F.,.F.,(3,3),(0.,1.),.UNSPECIFIED.);
#11158=B_SPLINE_CURVE_WITH_KNOTS('',2,(#41334,#41335,#41336),
 .UNSPECIFIED.,.F.,.F.,(3,3),(0.,1.),.UNSPECIFIED.);
#11159=B_SPLINE_CURVE_WITH_KNOTS('',2,(#41345,#41346,#41347),
 .UNSPECIFIED.,.F.,.F.,(3,3),(0.,1.),.UNSPECIFIED.);
#11160=B_SPLINE_CURVE_WITH_KNOTS('',2,(#41356,#41357,#41358),
 .UNSPECIFIED.,.F.,.F.,(3,3),(0.,1.),.UNSPECIFIED.);
#11161=B_SPLINE_CURVE_WITH_KNOTS('',2,(#41367,#41368,#41369),
 .UNSPECIFIED.,.F.,.F.,(3,3),(0.,1.),.UNSPECIFIED.);
#11162=B_SPLINE_CURVE_WITH_KNOTS('',2,(#41378,#41379,#41380),
 .UNSPECIFIED.,.F.,.F.,(3,3),(0.,1.),.UNSPECIFIED.);
#11163=B_SPLINE_CURVE_WITH_KNOTS('',2,(#41389,#41390,#41391),
 .UNSPECIFIED.,.F.,.F.,(3,3),(0.,1.),.UNSPECIFIED.);
#11164=B_SPLINE_CURVE_WITH_KNOTS('',2,(#41400,#41401,#41402),
 .UNSPECIFIED.,.F.,.F.,(3,3),(0.,1.),.UNSPECIFIED.);
#11165=B_SPLINE_CURVE_WITH_KNOTS('',2,(#41434,#41435,#41436),
 .UNSPECIFIED.,.F.,.F.,(3,3),(0.,1.),.UNSPECIFIED.);
#11166=B_SPLINE_CURVE_WITH_KNOTS('',2,(#41445,#41446,#41447),
 .UNSPECIFIED.,.F.,.F.,(3,3),(0.,1.),.UNSPECIFIED.);
#11672=VERTEX_POINT('',#38610);
#11673=VERTEX_POINT('',#38611);
#11674=VERTEX_POINT('',#38667);
#11675=VERTEX_POINT('',#38672);
#11676=VERTEX_POINT('',#38753);
#11677=VERTEX_POINT('',#38760);
#11678=VERTEX_POINT('',#38769);
#11679=VERTEX_POINT('',#38770);
#11680=VERTEX_POINT('',#38775);
#11681=VERTEX_POINT('',#38777);
#11682=VERTEX_POINT('',#38779);
#11683=VERTEX_POINT('',#38781);
#11684=VERTEX_POINT('',#38783);
#11685=VERTEX_POINT('',#38787);
#11686=VERTEX_POINT('',#38789);
#11687=VERTEX_POINT('',#38853);
#11688=VERTEX_POINT('',#38880);
#11689=VERTEX_POINT('',#38968);
#11690=VERTEX_POINT('',#38978);
#11691=VERTEX_POINT('',#38982);
#11692=VERTEX_POINT('',#38995);
#11693=VERTEX_POINT('',#39022);
#11694=VERTEX_POINT('',#39023);
#11695=VERTEX_POINT('',#39079);
#11696=VERTEX_POINT('',#39084);
#11697=VERTEX_POINT('',#39165);
#11698=VERTEX_POINT('',#39172);
#11699=VERTEX_POINT('',#39181);
#11700=VERTEX_POINT('',#39182);
#11701=VERTEX_POINT('',#39187);
#11702=VERTEX_POINT('',#39189);
#11703=VERTEX_POINT('',#39191);
#11704=VERTEX_POINT('',#39195);
#11705=VERTEX_POINT('',#39199);
#11706=VERTEX_POINT('',#39226);
#11707=VERTEX_POINT('',#39227);
#11708=VERTEX_POINT('',#39283);
#11709=VERTEX_POINT('',#39288);
#11710=VERTEX_POINT('',#39369);
#11711=VERTEX_POINT('',#39376);
#11712=VERTEX_POINT('',#39385);
#11713=VERTEX_POINT('',#39386);
#11714=VERTEX_POINT('',#39391);
#11715=VERTEX_POINT('',#39393);
#11716=VERTEX_POINT('',#39395);
#11717=VERTEX_POINT('',#39397);
#11718=VERTEX_POINT('',#39401);
#11719=VERTEX_POINT('',#39403);
#11720=VERTEX_POINT('',#39466);
#11721=VERTEX_POINT('',#39493);
#11722=VERTEX_POINT('',#39577);
#11723=VERTEX_POINT('',#39586);
#11724=VERTEX_POINT('',#39590);
#11725=VERTEX_POINT('',#39603);
#11726=VERTEX_POINT('',#39630);
#11727=VERTEX_POINT('',#39631);
#11728=VERTEX_POINT('',#39687);
#11729=VERTEX_POINT('',#39692);
#11730=VERTEX_POINT('',#39777);
#11731=VERTEX_POINT('',#39785);
#11732=VERTEX_POINT('',#39795);
#11733=VERTEX_POINT('',#39796);
#11734=VERTEX_POINT('',#39801);
#11735=VERTEX_POINT('',#39803);
#11736=VERTEX_POINT('',#39805);
#11737=VERTEX_POINT('',#39807);
#11738=VERTEX_POINT('',#39811);
#11739=VERTEX_POINT('',#39813);
#11740=VERTEX_POINT('',#39877);
#11741=VERTEX_POINT('',#39904);
#11742=VERTEX_POINT('',#39992);
#11743=VERTEX_POINT('',#40002);
#11744=VERTEX_POINT('',#40006);
#11745=VERTEX_POINT('',#40019);
#11746=VERTEX_POINT('',#40023);
#11747=VERTEX_POINT('',#40025);
#11748=VERTEX_POINT('',#40029);
#11749=VERTEX_POINT('',#40033);
#11750=VERTEX_POINT('',#40037);
#11751=VERTEX_POINT('',#40041);
#11752=VERTEX_POINT('',#40043);
#11753=VERTEX_POINT('',#40045);
#11754=VERTEX_POINT('',#40047);
#11755=VERTEX_POINT('',#40049);
#11756=VERTEX_POINT('',#40051);
#11757=VERTEX_POINT('',#40053);
#11758=VERTEX_POINT('',#40055);
#11759=VERTEX_POINT('',#40057);
#11760=VERTEX_POINT('',#40059);
#11761=VERTEX_POINT('',#40061);
#11762=VERTEX_POINT('',#40064);
#11763=VERTEX_POINT('',#40067);
#11764=VERTEX_POINT('',#40070);
#11765=VERTEX_POINT('',#40074);
#11766=VERTEX_POINT('',#40089);
#11767=VERTEX_POINT('',#40104);
#11768=VERTEX_POINT('',#40108);
#11769=VERTEX_POINT('',#40109);
#11770=VERTEX_POINT('',#40111);
#11771=VERTEX_POINT('',#40113);
#11772=VERTEX_POINT('',#40115);
#11773=VERTEX_POINT('',#40117);
#11774=VERTEX_POINT('',#40119);
#11775=VERTEX_POINT('',#40121);
#11776=VERTEX_POINT('',#40123);
#11777=VERTEX_POINT('',#40125);
#11778=VERTEX_POINT('',#40127);
#11779=VERTEX_POINT('',#40129);
#11780=VERTEX_POINT('',#40131);
#11781=VERTEX_POINT('',#40133);
#11782=VERTEX_POINT('',#40135);
#11783=VERTEX_POINT('',#40137);
#11784=VERTEX_POINT('',#40139);
#11785=VERTEX_POINT('',#40141);
#11786=VERTEX_POINT('',#40143);
#11787=VERTEX_POINT('',#40145);
#11788=VERTEX_POINT('',#40147);
#11789=VERTEX_POINT('',#40149);
#11790=VERTEX_POINT('',#40151);
#11791=VERTEX_POINT('',#40153);
#11792=VERTEX_POINT('',#40155);
#11793=VERTEX_POINT('',#40159);
#11794=VERTEX_POINT('',#40161);
#11795=VERTEX_POINT('',#40165);
#11796=VERTEX_POINT('',#40169);
#11797=VERTEX_POINT('',#40170);
#11798=VERTEX_POINT('',#40174);
#11799=VERTEX_POINT('',#40178);
#11800=VERTEX_POINT('',#40182);
#11801=VERTEX_POINT('',#40184);
#11802=VERTEX_POINT('',#40188);
#11803=VERTEX_POINT('',#40192);
#11804=VERTEX_POINT('',#40196);
#11805=VERTEX_POINT('',#40200);
#11806=VERTEX_POINT('',#40204);
#11807=VERTEX_POINT('',#40208);
#11808=VERTEX_POINT('',#40212);
#11809=VERTEX_POINT('',#40216);
#11810=VERTEX_POINT('',#40220);
#11811=VERTEX_POINT('',#40224);
#11812=VERTEX_POINT('',#40228);
#11813=VERTEX_POINT('',#40232);
#11814=VERTEX_POINT('',#40236);
#11815=VERTEX_POINT('',#40240);
#11816=VERTEX_POINT('',#40244);
#11817=VERTEX_POINT('',#40248);
#11818=VERTEX_POINT('',#40252);
#11819=VERTEX_POINT('',#40256);
#11820=VERTEX_POINT('',#40258);
#11821=VERTEX_POINT('',#40262);
#11822=VERTEX_POINT('',#40266);
#11823=VERTEX_POINT('',#40270);
#11824=VERTEX_POINT('',#40274);
#11825=VERTEX_POINT('',#40278);
#11826=VERTEX_POINT('',#40282);
#11827=VERTEX_POINT('',#40286);
#11828=VERTEX_POINT('',#40290);
#11829=VERTEX_POINT('',#40294);
#11830=VERTEX_POINT('',#40298);
#11831=VERTEX_POINT('',#40305);
#11832=VERTEX_POINT('',#40306);
#11833=VERTEX_POINT('',#40308);
#11834=VERTEX_POINT('',#40310);
#11835=VERTEX_POINT('',#40312);
#11836=VERTEX_POINT('',#40314);
#11837=VERTEX_POINT('',#40316);
#11838=VERTEX_POINT('',#40318);
#11839=VERTEX_POINT('',#40320);
#11840=VERTEX_POINT('',#40324);
#11841=VERTEX_POINT('',#40328);
#11842=VERTEX_POINT('',#40331);
#11843=VERTEX_POINT('',#40332);
#11844=VERTEX_POINT('',#40334);
#11845=VERTEX_POINT('',#40336);
#11846=VERTEX_POINT('',#40338);
#11847=VERTEX_POINT('',#40340);
#11848=VERTEX_POINT('',#40342);
#11849=VERTEX_POINT('',#40344);
#11850=VERTEX_POINT('',#40346);
#11851=VERTEX_POINT('',#40348);
#11852=VERTEX_POINT('',#40350);
#11853=VERTEX_POINT('',#40352);
#11854=VERTEX_POINT('',#40355);
#11855=VERTEX_POINT('',#40356);
#11856=VERTEX_POINT('',#40358);
#11857=VERTEX_POINT('',#40362);
#11858=VERTEX_POINT('',#40366);
#11859=VERTEX_POINT('',#40370);
#11860=VERTEX_POINT('',#40374);
#11861=VERTEX_POINT('',#40378);
#11862=VERTEX_POINT('',#40382);
#11863=VERTEX_POINT('',#40386);
#11864=VERTEX_POINT('',#40390);
#11865=VERTEX_POINT('',#40394);
#11866=VERTEX_POINT('',#40398);
#11867=VERTEX_POINT('',#40402);
#11868=VERTEX_POINT('',#40405);
#11869=VERTEX_POINT('',#40406);
#11870=VERTEX_POINT('',#40408);
#11871=VERTEX_POINT('',#40412);
#11872=VERTEX_POINT('',#40416);
#11873=VERTEX_POINT('',#40420);
#11874=VERTEX_POINT('',#40424);
#11875=VERTEX_POINT('',#40428);
#11876=VERTEX_POINT('',#40432);
#11877=VERTEX_POINT('',#40436);
#11878=VERTEX_POINT('',#40438);
#11879=VERTEX_POINT('',#40440);
#11880=VERTEX_POINT('',#40442);
#11881=VERTEX_POINT('',#40444);
#11882=VERTEX_POINT('',#40446);
#11883=VERTEX_POINT('',#40448);
#11884=VERTEX_POINT('',#40450);
#11885=VERTEX_POINT('',#40452);
#11886=VERTEX_POINT('',#40454);
#11887=VERTEX_POINT('',#40456);
#11888=VERTEX_POINT('',#40460);
#11889=VERTEX_POINT('',#40464);
#11890=VERTEX_POINT('',#40468);
#11891=VERTEX_POINT('',#40472);
#11892=VERTEX_POINT('',#40474);
#11893=VERTEX_POINT('',#40476);
#11894=VERTEX_POINT('',#40480);
#11895=VERTEX_POINT('',#40493);
#11896=VERTEX_POINT('',#40499);
#11897=VERTEX_POINT('',#40514);
#11898=VERTEX_POINT('',#40518);
#11899=VERTEX_POINT('',#40536);
#11900=VERTEX_POINT('',#40537);
#11901=VERTEX_POINT('',#40539);
#11902=VERTEX_POINT('',#40554);
#11903=VERTEX_POINT('',#40571);
#11904=VERTEX_POINT('',#40573);
#11905=VERTEX_POINT('',#40586);
#11906=VERTEX_POINT('',#40588);
#11907=VERTEX_POINT('',#40603);
#11908=VERTEX_POINT('',#40604);
#11909=VERTEX_POINT('',#40607);
#11910=VERTEX_POINT('',#40611);
#11911=VERTEX_POINT('',#40613);
#11912=VERTEX_POINT('',#40616);
#11913=VERTEX_POINT('',#40640);
#11914=VERTEX_POINT('',#40642);
#11915=VERTEX_POINT('',#40666);
#11916=VERTEX_POINT('',#40670);
#11917=VERTEX_POINT('',#40672);
#11918=VERTEX_POINT('',#40676);
#11919=VERTEX_POINT('',#40678);
#11920=VERTEX_POINT('',#40682);
#11921=VERTEX_POINT('',#40684);
#11922=VERTEX_POINT('',#40688);
#11923=VERTEX_POINT('',#40690);
#11924=VERTEX_POINT('',#40692);
#11925=VERTEX_POINT('',#40696);
#11926=VERTEX_POINT('',#40698);
#11927=VERTEX_POINT('',#40702);
#11928=VERTEX_POINT('',#40704);
#11929=VERTEX_POINT('',#40708);
#11930=VERTEX_POINT('',#40716);
#11931=VERTEX_POINT('',#40719);
#11932=VERTEX_POINT('',#40721);
#11933=VERTEX_POINT('',#40728);
#11934=VERTEX_POINT('',#40730);
#11935=VERTEX_POINT('',#40734);
#11936=VERTEX_POINT('',#40738);
#11937=VERTEX_POINT('',#40742);
#11938=VERTEX_POINT('',#40746);
#11939=VERTEX_POINT('',#40750);
#11940=VERTEX_POINT('',#40754);
#11941=VERTEX_POINT('',#40758);
#11942=VERTEX_POINT('',#40764);
#11943=VERTEX_POINT('',#40776);
#11944=VERTEX_POINT('',#40778);
#11945=VERTEX_POINT('',#40789);
#11946=VERTEX_POINT('',#40800);
#11947=VERTEX_POINT('',#40811);
#11948=VERTEX_POINT('',#40822);
#11949=VERTEX_POINT('',#40833);
#11950=VERTEX_POINT('',#40844);
#11951=VERTEX_POINT('',#40855);
#11952=VERTEX_POINT('',#40866);
#11953=VERTEX_POINT('',#40877);
#11954=VERTEX_POINT('',#40885);
#11955=VERTEX_POINT('',#40904);
#11956=VERTEX_POINT('',#40906);
#11957=VERTEX_POINT('',#40917);
#11958=VERTEX_POINT('',#40928);
#11959=VERTEX_POINT('',#40939);
#11960=VERTEX_POINT('',#40950);
#11961=VERTEX_POINT('',#40961);
#11962=VERTEX_POINT('',#40972);
#11963=VERTEX_POINT('',#40983);
#11964=VERTEX_POINT('',#40994);
#11965=VERTEX_POINT('',#41005);
#11966=VERTEX_POINT('',#41016);
#11967=VERTEX_POINT('',#41027);
#11968=VERTEX_POINT('',#41038);
#11969=VERTEX_POINT('',#41044);
#11970=VERTEX_POINT('',#41053);
#11971=VERTEX_POINT('',#41064);
#11972=VERTEX_POINT('',#41075);
#11973=VERTEX_POINT('',#41086);
#11974=VERTEX_POINT('',#41097);
#11975=VERTEX_POINT('',#41108);
#11976=VERTEX_POINT('',#41119);
#11977=VERTEX_POINT('',#41130);
#11978=VERTEX_POINT('',#41141);
#11979=VERTEX_POINT('',#41152);
#11980=VERTEX_POINT('',#41163);
#11981=VERTEX_POINT('',#41174);
#11982=VERTEX_POINT('',#41185);
#11983=VERTEX_POINT('',#41196);
#11984=VERTEX_POINT('',#41207);
#11985=VERTEX_POINT('',#41218);
#11986=VERTEX_POINT('',#41229);
#11987=VERTEX_POINT('',#41240);
#11988=VERTEX_POINT('',#41246);
#11989=VERTEX_POINT('',#41255);
#11990=VERTEX_POINT('',#41271);
#11991=VERTEX_POINT('',#41273);
#11992=VERTEX_POINT('',#41282);
#11993=VERTEX_POINT('',#41293);
#11994=VERTEX_POINT('',#41304);
#11995=VERTEX_POINT('',#41315);
#11996=VERTEX_POINT('',#41323);
#11997=VERTEX_POINT('',#41332);
#11998=VERTEX_POINT('',#41343);
#11999=VERTEX_POINT('',#41354);
#12000=VERTEX_POINT('',#41365);
#12001=VERTEX_POINT('',#41376);
#12002=VERTEX_POINT('',#41387);
#12003=VERTEX_POINT('',#41398);
#12004=VERTEX_POINT('',#41406);
#12005=VERTEX_POINT('',#41413);
#12006=VERTEX_POINT('',#41415);
#12007=VERTEX_POINT('',#41419);
#12008=VERTEX_POINT('',#41423);
#12009=VERTEX_POINT('',#41432);
#12010=VERTEX_POINT('',#41443);
#12011=VERTEX_POINT('',#41449);
#12012=VERTEX_POINT('',#41453);
#12013=VERTEX_POINT('',#41457);
#12014=VERTEX_POINT('',#41461);
#12015=VERTEX_POINT('',#41465);
#12016=VERTEX_POINT('',#41481);
#12017=VERTEX_POINT('',#41483);
#14250=EDGE_CURVE('',#11672,#11673,#10998,.T.);
#14251=EDGE_CURVE('',#11674,#11673,#10999,.T.);
#14252=EDGE_CURVE('',#11674,#11675,#11000,.T.);
#14253=EDGE_CURVE('',#11675,#11672,#1899,.T.);
#14254=EDGE_CURVE('',#11673,#11676,#11001,.T.);
#14255=EDGE_CURVE('',#11676,#11677,#1900,.T.);
#14256=EDGE_CURVE('',#11677,#11674,#11002,.T.);
#14257=EDGE_CURVE('',#11678,#11679,#1901,.F.);
#14258=EDGE_CURVE('',#11679,#11677,#1902,.T.);
#14259=EDGE_CURVE('',#11676,#11678,#1903,.T.);
#14260=EDGE_CURVE('',#11680,#11675,#1904,.T.);
#14261=EDGE_CURVE('',#11681,#11680,#1905,.T.);
#14262=EDGE_CURVE('',#11682,#11681,#1906,.T.);
#14263=EDGE_CURVE('',#11683,#11682,#10303,.T.);
#14264=EDGE_CURVE('',#11684,#11683,#10304,.T.);
#14265=EDGE_CURVE('',#11672,#11684,#1907,.T.);
#14266=EDGE_CURVE('',#11677,#11685,#1908,.T.);
#14267=EDGE_CURVE('',#11686,#11685,#11003,.T.);
#14268=EDGE_CURVE('',#11680,#11686,#11004,.T.);
#14269=EDGE_CURVE('',#11687,#11679,#1909,.T.);
#14270=EDGE_CURVE('',#11685,#11687,#1910,.T.);
#14271=EDGE_CURVE('',#11688,#11686,#11005,.T.);
#14272=EDGE_CURVE('',#11688,#11681,#11006,.T.);
#14273=EDGE_CURVE('',#11685,#11689,#1911,.T.);
#14274=EDGE_CURVE('',#11689,#11688,#11007,.T.);
#14275=EDGE_CURVE('',#11687,#11690,#1912,.F.);
#14276=EDGE_CURVE('',#11690,#11689,#1913,.T.);
#14277=EDGE_CURVE('',#11689,#11691,#1914,.T.);
#14278=EDGE_CURVE('',#11691,#11682,#11008,.F.);
#14279=EDGE_CURVE('',#11692,#11690,#1915,.T.);
#14280=EDGE_CURVE('',#11691,#11692,#1916,.T.);
#14281=EDGE_CURVE('',#11693,#11694,#11009,.T.);
#14282=EDGE_CURVE('',#11695,#11694,#11010,.T.);
#14283=EDGE_CURVE('',#11695,#11696,#11011,.T.);
#14284=EDGE_CURVE('',#11696,#11693,#1917,.T.);
#14285=EDGE_CURVE('',#11694,#11697,#11012,.T.);
#14286=EDGE_CURVE('',#11697,#11698,#1918,.T.);
#14287=EDGE_CURVE('',#11698,#11695,#11013,.T.);
#14288=EDGE_CURVE('',#11699,#11700,#1919,.F.);
#14289=EDGE_CURVE('',#11700,#11698,#1920,.T.);
#14290=EDGE_CURVE('',#11697,#11699,#1921,.T.);
#14291=EDGE_CURVE('',#11701,#11696,#1922,.T.);
#14292=EDGE_CURVE('',#11702,#11701,#1923,.T.);
#14293=EDGE_CURVE('',#11703,#11702,#10305,.T.);
#14294=EDGE_CURVE('',#11693,#11703,#1924,.T.);
#14295=EDGE_CURVE('',#11698,#11704,#1925,.T.);
#14296=EDGE_CURVE('',#11704,#11701,#10306,.T.);
#14297=EDGE_CURVE('',#11705,#11700,#1926,.T.);
#14298=EDGE_CURVE('',#11704,#11705,#1927,.T.);
#14299=EDGE_CURVE('',#11706,#11707,#11014,.T.);
#14300=EDGE_CURVE('',#11708,#11707,#11015,.T.);
#14301=EDGE_CURVE('',#11708,#11709,#11016,.T.);
#14302=EDGE_CURVE('',#11709,#11706,#1928,.T.);
#14303=EDGE_CURVE('',#11707,#11710,#11017,.T.);
#14304=EDGE_CURVE('',#11710,#11711,#1929,.T.);
#14305=EDGE_CURVE('',#11711,#11708,#11018,.T.);
#14306=EDGE_CURVE('',#11712,#11713,#1930,.F.);
#14307=EDGE_CURVE('',#11713,#11711,#1931,.T.);
#14308=EDGE_CURVE('',#11710,#11712,#1932,.T.);
#14309=EDGE_CURVE('',#11714,#11709,#1933,.T.);
#14310=EDGE_CURVE('',#11715,#11714,#1934,.T.);
#14311=EDGE_CURVE('',#11716,#11715,#1935,.T.);
#14312=EDGE_CURVE('',#11717,#11716,#10307,.T.);
#14313=EDGE_CURVE('',#11706,#11717,#1936,.T.);
#14314=EDGE_CURVE('',#11711,#11718,#1937,.T.);
#14315=EDGE_CURVE('',#11719,#11718,#11019,.T.);
#14316=EDGE_CURVE('',#11714,#11719,#11020,.T.);
#14317=EDGE_CURVE('',#11720,#11713,#1938,.T.);
#14318=EDGE_CURVE('',#11718,#11720,#1939,.T.);
#14319=EDGE_CURVE('',#11721,#11719,#11021,.T.);
#14320=EDGE_CURVE('',#11721,#11715,#11022,.T.);
#14321=EDGE_CURVE('',#11718,#11722,#1940,.T.);
#14322=EDGE_CURVE('',#11722,#11721,#11023,.T.);
#14323=EDGE_CURVE('',#11720,#11723,#1941,.F.);
#14324=EDGE_CURVE('',#11723,#11722,#1942,.T.);
#14325=EDGE_CURVE('',#11722,#11724,#1943,.T.);
#14326=EDGE_CURVE('',#11724,#11716,#11024,.F.);
#14327=EDGE_CURVE('',#11725,#11723,#1944,.T.);
#14328=EDGE_CURVE('',#11724,#11725,#1945,.T.);
#14329=EDGE_CURVE('',#11726,#11727,#11025,.T.);
#14330=EDGE_CURVE('',#11728,#11727,#11026,.T.);
#14331=EDGE_CURVE('',#11728,#11729,#11027,.T.);
#14332=EDGE_CURVE('',#11729,#11726,#1946,.T.);
#14333=EDGE_CURVE('',#11727,#11730,#11028,.T.);
#14334=EDGE_CURVE('',#11730,#11731,#1947,.T.);
#14335=EDGE_CURVE('',#11731,#11728,#11029,.T.);
#14336=EDGE_CURVE('',#11732,#11733,#1948,.F.);
#14337=EDGE_CURVE('',#11733,#11731,#1949,.T.);
#14338=EDGE_CURVE('',#11730,#11732,#1950,.T.);
#14339=EDGE_CURVE('',#11734,#11729,#1951,.T.);
#14340=EDGE_CURVE('',#11735,#11734,#1952,.T.);
#14341=EDGE_CURVE('',#11736,#11735,#1953,.T.);
#14342=EDGE_CURVE('',#11737,#11736,#10308,.T.);
#14343=EDGE_CURVE('',#11726,#11737,#1954,.T.);
#14344=EDGE_CURVE('',#11731,#11738,#1955,.T.);
#14345=EDGE_CURVE('',#11739,#11738,#11030,.T.);
#14346=EDGE_CURVE('',#11734,#11739,#11031,.T.);
#14347=EDGE_CURVE('',#11740,#11733,#1956,.T.);
#14348=EDGE_CURVE('',#11738,#11740,#1957,.T.);
#14349=EDGE_CURVE('',#11741,#11739,#11032,.T.);
#14350=EDGE_CURVE('',#11741,#11735,#11033,.T.);
#14351=EDGE_CURVE('',#11738,#11742,#1958,.T.);
#14352=EDGE_CURVE('',#11742,#11741,#11034,.T.);
#14353=EDGE_CURVE('',#11740,#11743,#1959,.F.);
#14354=EDGE_CURVE('',#11743,#11742,#1960,.T.);
#14355=EDGE_CURVE('',#11742,#11744,#1961,.T.);
#14356=EDGE_CURVE('',#11744,#11736,#11035,.F.);
#14357=EDGE_CURVE('',#11745,#11743,#1962,.T.);
#14358=EDGE_CURVE('',#11744,#11745,#1963,.T.);
#14359=EDGE_CURVE('',#11746,#11746,#10309,.T.);
#14360=EDGE_CURVE('',#11746,#11747,#10310,.T.);
#14361=EDGE_CURVE('',#11747,#11747,#10311,.T.);
#14362=EDGE_CURVE('',#11747,#11748,#1964,.T.);
#14363=EDGE_CURVE('',#11748,#11748,#10312,.T.);
#14364=EDGE_CURVE('',#11749,#11749,#10313,.T.);
#14365=EDGE_CURVE('',#11749,#11746,#1965,.T.);
#14366=EDGE_CURVE('',#11748,#11750,#10314,.T.);
#14367=EDGE_CURVE('',#11750,#11750,#10315,.T.);
#14368=EDGE_CURVE('',#11751,#11751,#10316,.T.);
#14369=EDGE_CURVE('',#11752,#11752,#10317,.T.);
#14370=EDGE_CURVE('',#11753,#11753,#10318,.T.);
#14371=EDGE_CURVE('',#11754,#11754,#10319,.T.);
#14372=EDGE_CURVE('',#11755,#11755,#10320,.T.);
#14373=EDGE_CURVE('',#11756,#11756,#10321,.T.);
#14374=EDGE_CURVE('',#11757,#11757,#10322,.T.);
#14375=EDGE_CURVE('',#11758,#11758,#10323,.T.);
#14376=EDGE_CURVE('',#11678,#11759,#1966,.T.);
#14377=EDGE_CURVE('',#11759,#11760,#10324,.T.);
#14378=EDGE_CURVE('',#11760,#11761,#1967,.T.);
#14379=EDGE_CURVE('',#11705,#11761,#10325,.F.);
#14380=EDGE_CURVE('',#11699,#11762,#1968,.T.);
#14381=EDGE_CURVE('',#11762,#11725,#10326,.T.);
#14382=EDGE_CURVE('',#11712,#11763,#1969,.T.);
#14383=EDGE_CURVE('',#11763,#11745,#10327,.T.);
#14384=EDGE_CURVE('',#11732,#11764,#1970,.T.);
#14385=EDGE_CURVE('',#11764,#11692,#10328,.T.);
#14386=EDGE_CURVE('',#11737,#11765,#11036,.F.);
#14387=EDGE_CURVE('',#11765,#11730,#1971,.T.);
#14388=EDGE_CURVE('',#11764,#11765,#1972,.T.);
#14389=EDGE_CURVE('',#11717,#11766,#11037,.F.);
#14390=EDGE_CURVE('',#11766,#11710,#1973,.T.);
#14391=EDGE_CURVE('',#11763,#11766,#1974,.T.);
#14392=EDGE_CURVE('',#11767,#11767,#10329,.T.);
#14393=EDGE_CURVE('',#11767,#11749,#10330,.T.);
#14394=EDGE_CURVE('',#11768,#11769,#10331,.T.);
#14395=EDGE_CURVE('',#11768,#11770,#10332,.T.);
#14396=EDGE_CURVE('',#11770,#11771,#10333,.T.);
#14397=EDGE_CURVE('',#11772,#11771,#10334,.T.);
#14398=EDGE_CURVE('',#11772,#11773,#10335,.T.);
#14399=EDGE_CURVE('',#11773,#11774,#10336,.T.);
#14400=EDGE_CURVE('',#11775,#11774,#10337,.T.);
#14401=EDGE_CURVE('',#11775,#11776,#10338,.T.);
#14402=EDGE_CURVE('',#11776,#11777,#10339,.T.);
#14403=EDGE_CURVE('',#11778,#11777,#10340,.T.);
#14404=EDGE_CURVE('',#11778,#11779,#10341,.T.);
#14405=EDGE_CURVE('',#11779,#11780,#10342,.T.);
#14406=EDGE_CURVE('',#11781,#11780,#10343,.T.);
#14407=EDGE_CURVE('',#11781,#11782,#10344,.T.);
#14408=EDGE_CURVE('',#11782,#11783,#10345,.T.);
#14409=EDGE_CURVE('',#11784,#11783,#10346,.T.);
#14410=EDGE_CURVE('',#11784,#11785,#10347,.T.);
#14411=EDGE_CURVE('',#11785,#11786,#10348,.T.);
#14412=EDGE_CURVE('',#11787,#11786,#10349,.T.);
#14413=EDGE_CURVE('',#11788,#11787,#10350,.T.);
#14414=EDGE_CURVE('',#11788,#11789,#10351,.T.);
#14415=EDGE_CURVE('',#11789,#11790,#10352,.T.);
#14416=EDGE_CURVE('',#11791,#11790,#10353,.T.);
#14417=EDGE_CURVE('',#11791,#11792,#10354,.T.);
#14418=EDGE_CURVE('',#11792,#11769,#10355,.T.);
#14419=EDGE_CURVE('',#11793,#11793,#10356,.T.);
#14420=EDGE_CURVE('',#11793,#11794,#10357,.T.);
#14421=EDGE_CURVE('',#11794,#11794,#10358,.T.);
#14422=EDGE_CURVE('',#11795,#11795,#10359,.T.);
#14423=EDGE_CURVE('',#11795,#11793,#1975,.T.);
#14424=EDGE_CURVE('',#11796,#11797,#11038,.T.);
#14425=EDGE_CURVE('',#11797,#11798,#11039,.T.);
#14426=EDGE_CURVE('',#11798,#11799,#11040,.T.);
#14427=EDGE_CURVE('',#11799,#11800,#1976,.T.);
#14428=EDGE_CURVE('',#11800,#11801,#11041,.T.);
#14429=EDGE_CURVE('',#11801,#11802,#11042,.T.);
#14430=EDGE_CURVE('',#11802,#11803,#11043,.T.);
#14431=EDGE_CURVE('',#11803,#11804,#11044,.T.);
#14432=EDGE_CURVE('',#11804,#11805,#11045,.T.);
#14433=EDGE_CURVE('',#11805,#11806,#11046,.T.);
#14434=EDGE_CURVE('',#11806,#11807,#11047,.T.);
#14435=EDGE_CURVE('',#11807,#11808,#11048,.T.);
#14436=EDGE_CURVE('',#11808,#11809,#11049,.T.);
#14437=EDGE_CURVE('',#11809,#11810,#11050,.T.);
#14438=EDGE_CURVE('',#11810,#11811,#11051,.T.);
#14439=EDGE_CURVE('',#11811,#11812,#11052,.T.);
#14440=EDGE_CURVE('',#11812,#11813,#11053,.T.);
#14441=EDGE_CURVE('',#11813,#11814,#11054,.T.);
#14442=EDGE_CURVE('',#11814,#11815,#11055,.T.);
#14443=EDGE_CURVE('',#11815,#11816,#11056,.T.);
#14444=EDGE_CURVE('',#11816,#11817,#11057,.T.);
#14445=EDGE_CURVE('',#11817,#11818,#11058,.T.);
#14446=EDGE_CURVE('',#11818,#11819,#1977,.T.);
#14447=EDGE_CURVE('',#11819,#11820,#11059,.T.);
#14448=EDGE_CURVE('',#11820,#11821,#11060,.T.);
#14449=EDGE_CURVE('',#11821,#11822,#11061,.T.);
#14450=EDGE_CURVE('',#11822,#11823,#11062,.T.);
#14451=EDGE_CURVE('',#11823,#11824,#11063,.T.);
#14452=EDGE_CURVE('',#11824,#11825,#11064,.T.);
#14453=EDGE_CURVE('',#11825,#11826,#11065,.T.);
#14454=EDGE_CURVE('',#11826,#11827,#11066,.T.);
#14455=EDGE_CURVE('',#11827,#11828,#11067,.T.);
#14456=EDGE_CURVE('',#11828,#11829,#11068,.T.);
#14457=EDGE_CURVE('',#11829,#11830,#11069,.T.);
#14458=EDGE_CURVE('',#11830,#11796,#11070,.T.);
#14459=EDGE_CURVE('',#11831,#11832,#1978,.T.);
#14460=EDGE_CURVE('',#11832,#11833,#1979,.T.);
#14461=EDGE_CURVE('',#11833,#11834,#1980,.T.);
#14462=EDGE_CURVE('',#11834,#11835,#1981,.T.);
#14463=EDGE_CURVE('',#11835,#11836,#1982,.T.);
#14464=EDGE_CURVE('',#11836,#11837,#1983,.T.);
#14465=EDGE_CURVE('',#11837,#11838,#1984,.T.);
#14466=EDGE_CURVE('',#11838,#11839,#11071,.T.);
#14467=EDGE_CURVE('',#11839,#11840,#11072,.T.);
#14468=EDGE_CURVE('',#11840,#11841,#1985,.T.);
#14469=EDGE_CURVE('',#11841,#11831,#1986,.T.);
#14470=EDGE_CURVE('',#11842,#11843,#1987,.T.);
#14471=EDGE_CURVE('',#11843,#11844,#1988,.T.);
#14472=EDGE_CURVE('',#11844,#11845,#1989,.T.);
#14473=EDGE_CURVE('',#11845,#11846,#1990,.T.);
#14474=EDGE_CURVE('',#11846,#11847,#1991,.T.);
#14475=EDGE_CURVE('',#11847,#11848,#1992,.T.);
#14476=EDGE_CURVE('',#11848,#11849,#1993,.T.);
#14477=EDGE_CURVE('',#11849,#11850,#1994,.T.);
#14478=EDGE_CURVE('',#11850,#11851,#1995,.T.);
#14479=EDGE_CURVE('',#11851,#11852,#1996,.T.);
#14480=EDGE_CURVE('',#11853,#11852,#1997,.T.);
#14481=EDGE_CURVE('',#11842,#11853,#1998,.T.);
#14482=EDGE_CURVE('',#11854,#11855,#1999,.T.);
#14483=EDGE_CURVE('',#11855,#11856,#11073,.T.);
#14484=EDGE_CURVE('',#11856,#11857,#11074,.T.);
#14485=EDGE_CURVE('',#11857,#11858,#11075,.T.);
#14486=EDGE_CURVE('',#11858,#11859,#11076,.T.);
#14487=EDGE_CURVE('',#11859,#11860,#11077,.T.);
#14488=EDGE_CURVE('',#11860,#11861,#11078,.T.);
#14489=EDGE_CURVE('',#11861,#11862,#11079,.T.);
#14490=EDGE_CURVE('',#11862,#11863,#11080,.T.);
#14491=EDGE_CURVE('',#11863,#11864,#11081,.T.);
#14492=EDGE_CURVE('',#11864,#11865,#11082,.T.);
#14493=EDGE_CURVE('',#11865,#11866,#11083,.T.);
#14494=EDGE_CURVE('',#11867,#11866,#2000,.T.);
#14495=EDGE_CURVE('',#11854,#11867,#2001,.T.);
#14496=EDGE_CURVE('',#11868,#11869,#2002,.T.);
#14497=EDGE_CURVE('',#11869,#11870,#11084,.T.);
#14498=EDGE_CURVE('',#11870,#11871,#11085,.T.);
#14499=EDGE_CURVE('',#11871,#11872,#11086,.T.);
#14500=EDGE_CURVE('',#11872,#11873,#11087,.T.);
#14501=EDGE_CURVE('',#11873,#11874,#11088,.T.);
#14502=EDGE_CURVE('',#11874,#11875,#11089,.T.);
#14503=EDGE_CURVE('',#11875,#11876,#11090,.T.);
#14504=EDGE_CURVE('',#11876,#11877,#2003,.T.);
#14505=EDGE_CURVE('',#11878,#11877,#2004,.T.);
#14506=EDGE_CURVE('',#11879,#11878,#2005,.T.);
#14507=EDGE_CURVE('',#11880,#11879,#2006,.T.);
#14508=EDGE_CURVE('',#11880,#11881,#2007,.T.);
#14509=EDGE_CURVE('',#11881,#11882,#2008,.T.);
#14510=EDGE_CURVE('',#11882,#11883,#2009,.T.);
#14511=EDGE_CURVE('',#11883,#11884,#2010,.T.);
#14512=EDGE_CURVE('',#11884,#11885,#2011,.T.);
#14513=EDGE_CURVE('',#11885,#11886,#2012,.T.);
#14514=EDGE_CURVE('',#11886,#11887,#11091,.T.);
#14515=EDGE_CURVE('',#11887,#11888,#11092,.T.);
#14516=EDGE_CURVE('',#11888,#11889,#11093,.T.);
#14517=EDGE_CURVE('',#11889,#11890,#11094,.T.);
#14518=EDGE_CURVE('',#11890,#11891,#2013,.T.);
#14519=EDGE_CURVE('',#11891,#11892,#2014,.T.);
#14520=EDGE_CURVE('',#11893,#11892,#2015,.T.);
#14521=EDGE_CURVE('',#11868,#11893,#2016,.T.);
#14522=EDGE_CURVE('',#11703,#11894,#11095,.F.);
#14523=EDGE_CURVE('',#11894,#11697,#2017,.T.);
#14524=EDGE_CURVE('',#11895,#11704,#10360,.T.);
#14525=EDGE_CURVE('',#11761,#11895,#2018,.T.);
#14526=EDGE_CURVE('',#11895,#11701,#10361,.T.);
#14527=EDGE_CURVE('',#11895,#11896,#2019,.T.);
#14528=EDGE_CURVE('',#11896,#11702,#11096,.F.);
#14529=EDGE_CURVE('',#11896,#11760,#2020,.T.);
#14530=EDGE_CURVE('',#11897,#11897,#10362,.T.);
#14531=EDGE_CURVE('',#11897,#11795,#10363,.T.);
#14532=EDGE_CURVE('',#11759,#11898,#2021,.T.);
#14533=EDGE_CURVE('',#11684,#11898,#11097,.F.);
#14534=EDGE_CURVE('',#11683,#11897,#2022,.T.);
#14535=EDGE_CURVE('',#11762,#11894,#2023,.T.);
#14536=EDGE_CURVE('',#11898,#11676,#2024,.T.);
#14537=EDGE_CURVE('',#11899,#11900,#10364,.T.);
#14538=EDGE_CURVE('',#11900,#11901,#11098,.T.);
#14539=EDGE_CURVE('',#11901,#11902,#10365,.T.);
#14540=EDGE_CURVE('',#11902,#11899,#11099,.T.);
#14541=EDGE_CURVE('',#11900,#11903,#2025,.T.);
#14542=EDGE_CURVE('',#11903,#11904,#11100,.F.);
#14543=EDGE_CURVE('',#11904,#11901,#2026,.T.);
#14544=EDGE_CURVE('',#11902,#11905,#2027,.T.);
#14545=EDGE_CURVE('',#11905,#11906,#11101,.F.);
#14546=EDGE_CURVE('',#11906,#11899,#2028,.T.);
#14547=EDGE_CURVE('',#11906,#11903,#10366,.T.);
#14548=EDGE_CURVE('',#11907,#11908,#10367,.T.);
#14549=EDGE_CURVE('',#11908,#11907,#10368,.T.);
#14550=EDGE_CURVE('',#11907,#11909,#10369,.T.);
#14551=EDGE_CURVE('',#11909,#11909,#10370,.T.);
#14552=EDGE_CURVE('',#11905,#11910,#2029,.T.);
#14553=EDGE_CURVE('',#11910,#11911,#10371,.T.);
#14554=EDGE_CURVE('',#11911,#11908,#2030,.T.);
#14555=EDGE_CURVE('',#11911,#11912,#10372,.T.);
#14556=EDGE_CURVE('',#11904,#11912,#2031,.T.);
#14557=EDGE_CURVE('',#11777,#11775,#11102,.T.);
#14558=EDGE_CURVE('',#11774,#11772,#11103,.T.);
#14559=EDGE_CURVE('',#11771,#11768,#11104,.T.);
#14560=EDGE_CURVE('',#11769,#11791,#11105,.T.);
#14561=EDGE_CURVE('',#11790,#11788,#11106,.T.);
#14562=EDGE_CURVE('',#11787,#11913,#10373,.T.);
#14563=EDGE_CURVE('',#11913,#11914,#10374,.T.);
#14564=EDGE_CURVE('',#11914,#11913,#10375,.T.);
#14565=EDGE_CURVE('',#11786,#11784,#11107,.T.);
#14566=EDGE_CURVE('',#11783,#11781,#11108,.T.);
#14567=EDGE_CURVE('',#11780,#11778,#11109,.T.);
#14568=EDGE_CURVE('',#11752,#11770,#2032,.T.);
#14569=EDGE_CURVE('',#11757,#11773,#2033,.T.);
#14570=EDGE_CURVE('',#11751,#11776,#2034,.T.);
#14571=EDGE_CURVE('',#11758,#11779,#2035,.T.);
#14572=EDGE_CURVE('',#11915,#11915,#10376,.T.);
#14573=EDGE_CURVE('',#11915,#11914,#2036,.T.);
#14574=EDGE_CURVE('',#11868,#11916,#10377,.T.);
#14575=EDGE_CURVE('',#11893,#11917,#10378,.F.);
#14576=EDGE_CURVE('',#11917,#11916,#2037,.T.);
#14577=EDGE_CURVE('',#11854,#11918,#10379,.T.);
#14578=EDGE_CURVE('',#11867,#11919,#10380,.F.);
#14579=EDGE_CURVE('',#11919,#11918,#2038,.T.);
#14580=EDGE_CURVE('',#11842,#11920,#10381,.T.);
#14581=EDGE_CURVE('',#11853,#11921,#10382,.F.);
#14582=EDGE_CURVE('',#11921,#11920,#2039,.T.);
#14583=EDGE_CURVE('',#11878,#11922,#197,.T.);
#14584=EDGE_CURVE('',#11877,#11923,#198,.T.);
#14585=EDGE_CURVE('',#11923,#11924,#199,.F.);
#14586=EDGE_CURVE('',#11924,#11922,#2040,.T.);
#14587=EDGE_CURVE('',#11880,#11925,#200,.T.);
#14588=EDGE_CURVE('',#11879,#11926,#201,.F.);
#14589=EDGE_CURVE('',#11926,#11925,#2041,.T.);
#14590=EDGE_CURVE('',#11882,#11927,#2042,.T.);
#14591=EDGE_CURVE('',#11927,#11928,#2043,.T.);
#14592=EDGE_CURVE('',#11883,#11928,#2044,.T.);
#14593=EDGE_CURVE('',#11881,#11929,#2045,.T.);
#14594=EDGE_CURVE('',#11929,#11927,#2046,.T.);
#14595=EDGE_CURVE('',#11925,#11929,#2047,.T.);
#14596=EDGE_CURVE('',#11922,#11926,#2048,.T.);
#14597=EDGE_CURVE('',#11884,#11930,#2049,.T.);
#14598=EDGE_CURVE('',#11930,#11924,#2050,.T.);
#14599=EDGE_CURVE('',#11923,#11931,#2051,.T.);
#14600=EDGE_CURVE('',#11931,#11932,#2052,.T.);
#14601=EDGE_CURVE('',#11885,#11932,#2053,.T.);
#14602=EDGE_CURVE('',#11928,#11930,#2054,.T.);
#14603=EDGE_CURVE('',#11850,#11933,#2055,.T.);
#14604=EDGE_CURVE('',#11933,#11934,#2056,.T.);
#14605=EDGE_CURVE('',#11851,#11934,#2057,.T.);
#14606=EDGE_CURVE('',#11849,#11935,#2058,.T.);
#14607=EDGE_CURVE('',#11935,#11933,#2059,.T.);
#14608=EDGE_CURVE('',#11848,#11936,#2060,.T.);
#14609=EDGE_CURVE('',#11936,#11935,#2061,.T.);
#14610=EDGE_CURVE('',#11847,#11937,#2062,.T.);
#14611=EDGE_CURVE('',#11937,#11936,#2063,.T.);
#14612=EDGE_CURVE('',#11846,#11938,#2064,.T.);
#14613=EDGE_CURVE('',#11938,#11937,#2065,.T.);
#14614=EDGE_CURVE('',#11845,#11939,#2066,.T.);
#14615=EDGE_CURVE('',#11939,#11938,#2067,.T.);
#14616=EDGE_CURVE('',#11844,#11940,#2068,.T.);
#14617=EDGE_CURVE('',#11940,#11939,#2069,.T.);
#14618=EDGE_CURVE('',#11843,#11941,#2070,.T.);
#14619=EDGE_CURVE('',#11941,#11940,#2071,.T.);
#14620=EDGE_CURVE('',#11920,#11941,#2072,.T.);
#14621=EDGE_CURVE('',#11852,#11942,#2073,.T.);
#14622=EDGE_CURVE('',#11942,#11921,#2074,.T.);
#14623=EDGE_CURVE('',#11934,#11942,#2075,.T.);
#14624=EDGE_CURVE('',#11864,#11943,#2076,.T.);
#14625=EDGE_CURVE('',#11943,#11944,#11110,.T.);
#14626=EDGE_CURVE('',#11865,#11944,#2077,.T.);
#14627=EDGE_CURVE('',#11863,#11945,#2078,.T.);
#14628=EDGE_CURVE('',#11945,#11943,#11111,.T.);
#14629=EDGE_CURVE('',#11862,#11946,#2079,.T.);
#14630=EDGE_CURVE('',#11946,#11945,#11112,.T.);
#14631=EDGE_CURVE('',#11861,#11947,#2080,.T.);
#14632=EDGE_CURVE('',#11947,#11946,#11113,.T.);
#14633=EDGE_CURVE('',#11860,#11948,#2081,.T.);
#14634=EDGE_CURVE('',#11948,#11947,#11114,.T.);
#14635=EDGE_CURVE('',#11859,#11949,#2082,.T.);
#14636=EDGE_CURVE('',#11949,#11948,#11115,.T.);
#14637=EDGE_CURVE('',#11858,#11950,#2083,.T.);
#14638=EDGE_CURVE('',#11950,#11949,#11116,.T.);
#14639=EDGE_CURVE('',#11857,#11951,#2084,.T.);
#14640=EDGE_CURVE('',#11951,#11950,#11117,.T.);
#14641=EDGE_CURVE('',#11856,#11952,#2085,.T.);
#14642=EDGE_CURVE('',#11952,#11951,#11118,.T.);
#14643=EDGE_CURVE('',#11855,#11953,#2086,.T.);
#14644=EDGE_CURVE('',#11953,#11952,#11119,.T.);
#14645=EDGE_CURVE('',#11918,#11953,#2087,.T.);
#14646=EDGE_CURVE('',#11866,#11954,#2088,.T.);
#14647=EDGE_CURVE('',#11954,#11919,#2089,.T.);
#14648=EDGE_CURVE('',#11944,#11954,#11120,.T.);
#14649=EDGE_CURVE('',#11796,#11955,#2090,.T.);
#14650=EDGE_CURVE('',#11955,#11956,#11121,.T.);
#14651=EDGE_CURVE('',#11797,#11956,#2091,.T.);
#14652=EDGE_CURVE('',#11830,#11957,#2092,.T.);
#14653=EDGE_CURVE('',#11957,#11955,#11122,.T.);
#14654=EDGE_CURVE('',#11829,#11958,#2093,.T.);
#14655=EDGE_CURVE('',#11958,#11957,#11123,.T.);
#14656=EDGE_CURVE('',#11828,#11959,#2094,.T.);
#14657=EDGE_CURVE('',#11959,#11958,#11124,.T.);
#14658=EDGE_CURVE('',#11827,#11960,#2095,.T.);
#14659=EDGE_CURVE('',#11960,#11959,#11125,.T.);
#14660=EDGE_CURVE('',#11826,#11961,#2096,.T.);
#14661=EDGE_CURVE('',#11961,#11960,#11126,.T.);
#14662=EDGE_CURVE('',#11825,#11962,#2097,.T.);
#14663=EDGE_CURVE('',#11962,#11961,#11127,.T.);
#14664=EDGE_CURVE('',#11824,#11963,#2098,.T.);
#14665=EDGE_CURVE('',#11963,#11962,#11128,.T.);
#14666=EDGE_CURVE('',#11823,#11964,#2099,.T.);
#14667=EDGE_CURVE('',#11964,#11963,#11129,.T.);
#14668=EDGE_CURVE('',#11822,#11965,#2100,.T.);
#14669=EDGE_CURVE('',#11965,#11964,#11130,.T.);
#14670=EDGE_CURVE('',#11821,#11966,#2101,.T.);
#14671=EDGE_CURVE('',#11966,#11965,#11131,.T.);
#14672=EDGE_CURVE('',#11820,#11967,#2102,.T.);
#14673=EDGE_CURVE('',#11967,#11966,#11132,.T.);
#14674=EDGE_CURVE('',#11819,#11968,#2103,.T.);
#14675=EDGE_CURVE('',#11968,#11967,#11133,.T.);
#14676=EDGE_CURVE('',#11818,#11969,#2104,.T.);
#14677=EDGE_CURVE('',#11969,#11968,#2105,.T.);
#14678=EDGE_CURVE('',#11817,#11970,#2106,.T.);
#14679=EDGE_CURVE('',#11970,#11969,#11134,.T.);
#14680=EDGE_CURVE('',#11816,#11971,#2107,.T.);
#14681=EDGE_CURVE('',#11971,#11970,#11135,.T.);
#14682=EDGE_CURVE('',#11815,#11972,#2108,.T.);
#14683=EDGE_CURVE('',#11972,#11971,#11136,.T.);
#14684=EDGE_CURVE('',#11814,#11973,#2109,.T.);
#14685=EDGE_CURVE('',#11973,#11972,#11137,.T.);
#14686=EDGE_CURVE('',#11813,#11974,#2110,.T.);
#14687=EDGE_CURVE('',#11974,#11973,#11138,.T.);
#14688=EDGE_CURVE('',#11812,#11975,#2111,.T.);
#14689=EDGE_CURVE('',#11975,#11974,#11139,.T.);
#14690=EDGE_CURVE('',#11811,#11976,#2112,.T.);
#14691=EDGE_CURVE('',#11976,#11975,#11140,.T.);
#14692=EDGE_CURVE('',#11810,#11977,#2113,.T.);
#14693=EDGE_CURVE('',#11977,#11976,#11141,.T.);
#14694=EDGE_CURVE('',#11809,#11978,#2114,.T.);
#14695=EDGE_CURVE('',#11978,#11977,#11142,.T.);
#14696=EDGE_CURVE('',#11808,#11979,#2115,.T.);
#14697=EDGE_CURVE('',#11979,#11978,#11143,.T.);
#14698=EDGE_CURVE('',#11807,#11980,#2116,.T.);
#14699=EDGE_CURVE('',#11980,#11979,#11144,.T.);
#14700=EDGE_CURVE('',#11806,#11981,#2117,.T.);
#14701=EDGE_CURVE('',#11981,#11980,#11145,.T.);
#14702=EDGE_CURVE('',#11805,#11982,#2118,.T.);
#14703=EDGE_CURVE('',#11982,#11981,#11146,.T.);
#14704=EDGE_CURVE('',#11804,#11983,#2119,.T.);
#14705=EDGE_CURVE('',#11983,#11982,#11147,.T.);
#14706=EDGE_CURVE('',#11803,#11984,#2120,.T.);
#14707=EDGE_CURVE('',#11984,#11983,#11148,.T.);
#14708=EDGE_CURVE('',#11802,#11985,#2121,.T.);
#14709=EDGE_CURVE('',#11985,#11984,#11149,.T.);
#14710=EDGE_CURVE('',#11801,#11986,#2122,.T.);
#14711=EDGE_CURVE('',#11986,#11985,#11150,.T.);
#14712=EDGE_CURVE('',#11800,#11987,#2123,.T.);
#14713=EDGE_CURVE('',#11987,#11986,#11151,.T.);
#14714=EDGE_CURVE('',#11799,#11988,#2124,.T.);
#14715=EDGE_CURVE('',#11988,#11987,#2125,.T.);
#14716=EDGE_CURVE('',#11798,#11989,#2126,.T.);
#14717=EDGE_CURVE('',#11989,#11988,#11152,.T.);
#14718=EDGE_CURVE('',#11956,#11989,#11153,.T.);
#14719=EDGE_CURVE('',#11890,#11990,#2127,.T.);
#14720=EDGE_CURVE('',#11990,#11991,#2128,.T.);
#14721=EDGE_CURVE('',#11891,#11991,#2129,.T.);
#14722=EDGE_CURVE('',#11889,#11992,#2130,.T.);
#14723=EDGE_CURVE('',#11992,#11990,#11154,.T.);
#14724=EDGE_CURVE('',#11888,#11993,#2131,.T.);
#14725=EDGE_CURVE('',#11993,#11992,#11155,.T.);
#14726=EDGE_CURVE('',#11887,#11994,#2132,.T.);
#14727=EDGE_CURVE('',#11994,#11993,#11156,.T.);
#14728=EDGE_CURVE('',#11886,#11995,#2133,.T.);
#14729=EDGE_CURVE('',#11995,#11994,#11157,.T.);
#14730=EDGE_CURVE('',#11932,#11995,#2134,.T.);
#14731=EDGE_CURVE('',#11876,#11996,#2135,.T.);
#14732=EDGE_CURVE('',#11996,#11931,#2136,.T.);
#14733=EDGE_CURVE('',#11875,#11997,#2137,.T.);
#14734=EDGE_CURVE('',#11997,#11996,#11158,.T.);
#14735=EDGE_CURVE('',#11874,#11998,#2138,.T.);
#14736=EDGE_CURVE('',#11998,#11997,#11159,.T.);
#14737=EDGE_CURVE('',#11873,#11999,#2139,.T.);
#14738=EDGE_CURVE('',#11999,#11998,#11160,.T.);
#14739=EDGE_CURVE('',#11872,#12000,#2140,.T.);
#14740=EDGE_CURVE('',#12000,#11999,#11161,.T.);
#14741=EDGE_CURVE('',#11871,#12001,#2141,.T.);
#14742=EDGE_CURVE('',#12001,#12000,#11162,.T.);
#14743=EDGE_CURVE('',#11870,#12002,#2142,.T.);
#14744=EDGE_CURVE('',#12002,#12001,#11163,.T.);
#14745=EDGE_CURVE('',#11869,#12003,#2143,.T.);
#14746=EDGE_CURVE('',#12003,#12002,#11164,.T.);
#14747=EDGE_CURVE('',#11916,#12003,#2144,.T.);
#14748=EDGE_CURVE('',#11892,#12004,#2145,.T.);
#14749=EDGE_CURVE('',#12004,#11917,#2146,.T.);
#14750=EDGE_CURVE('',#11991,#12004,#2147,.T.);
#14751=EDGE_CURVE('',#11831,#12005,#2148,.T.);
#14752=EDGE_CURVE('',#12005,#12006,#2149,.T.);
#14753=EDGE_CURVE('',#11832,#12006,#2150,.T.);
#14754=EDGE_CURVE('',#11841,#12007,#2151,.T.);
#14755=EDGE_CURVE('',#12007,#12005,#2152,.T.);
#14756=EDGE_CURVE('',#11840,#12008,#2153,.T.);
#14757=EDGE_CURVE('',#12008,#12007,#2154,.T.);
#14758=EDGE_CURVE('',#11839,#12009,#2155,.T.);
#14759=EDGE_CURVE('',#12009,#12008,#11165,.T.);
#14760=EDGE_CURVE('',#11838,#12010,#2156,.T.);
#14761=EDGE_CURVE('',#12010,#12009,#11166,.T.);
#14762=EDGE_CURVE('',#11837,#12011,#2157,.T.);
#14763=EDGE_CURVE('',#12011,#12010,#2158,.T.);
#14764=EDGE_CURVE('',#11836,#12012,#2159,.T.);
#14765=EDGE_CURVE('',#12012,#12011,#2160,.T.);
#14766=EDGE_CURVE('',#11835,#12013,#2161,.T.);
#14767=EDGE_CURVE('',#12013,#12012,#2162,.T.);
#14768=EDGE_CURVE('',#11834,#12014,#2163,.T.);
#14769=EDGE_CURVE('',#12014,#12013,#2164,.T.);
#14770=EDGE_CURVE('',#11833,#12015,#2165,.T.);
#14771=EDGE_CURVE('',#12015,#12014,#2166,.T.);
#14772=EDGE_CURVE('',#12006,#12015,#2167,.T.);
#14773=EDGE_CURVE('',#11753,#11792,#2168,.T.);
#14774=EDGE_CURVE('',#11754,#11785,#2169,.T.);
#14775=EDGE_CURVE('',#11755,#11789,#2170,.T.);
#14776=EDGE_CURVE('',#11756,#11782,#2171,.T.);
#14777=EDGE_CURVE('',#11901,#12016,#2172,.T.);
#14778=EDGE_CURVE('',#12016,#12017,#10383,.T.);
#14779=EDGE_CURVE('',#11902,#12017,#2173,.T.);
#14780=EDGE_CURVE('',#11912,#12016,#2174,.T.);
#14781=EDGE_CURVE('',#12017,#11910,#2175,.T.);
#18492=ORIENTED_EDGE('',*,*,#14250,.T.);
#18493=ORIENTED_EDGE('',*,*,#14251,.F.);
#18494=ORIENTED_EDGE('',*,*,#14252,.T.);
#18495=ORIENTED_EDGE('',*,*,#14253,.T.);
#18496=ORIENTED_EDGE('',*,*,#14251,.T.);
#18497=ORIENTED_EDGE('',*,*,#14254,.T.);
#18498=ORIENTED_EDGE('',*,*,#14255,.T.);
#18499=ORIENTED_EDGE('',*,*,#14256,.T.);
#18500=ORIENTED_EDGE('',*,*,#14257,.T.);
#18501=ORIENTED_EDGE('',*,*,#14258,.T.);
#18502=ORIENTED_EDGE('',*,*,#14255,.F.);
#18503=ORIENTED_EDGE('',*,*,#14259,.T.);
#18504=ORIENTED_EDGE('',*,*,#14253,.F.);
#18505=ORIENTED_EDGE('',*,*,#14260,.F.);
#18506=ORIENTED_EDGE('',*,*,#14261,.F.);
#18507=ORIENTED_EDGE('',*,*,#14262,.F.);
#18508=ORIENTED_EDGE('',*,*,#14263,.F.);
#18509=ORIENTED_EDGE('',*,*,#14264,.F.);
#18510=ORIENTED_EDGE('',*,*,#14265,.F.);
#18511=ORIENTED_EDGE('',*,*,#14252,.F.);
#18512=ORIENTED_EDGE('',*,*,#14256,.F.);
#18513=ORIENTED_EDGE('',*,*,#14266,.T.);
#18514=ORIENTED_EDGE('',*,*,#14267,.F.);
#18515=ORIENTED_EDGE('',*,*,#14268,.F.);
#18516=ORIENTED_EDGE('',*,*,#14260,.T.);
#18517=ORIENTED_EDGE('',*,*,#14258,.F.);
#18518=ORIENTED_EDGE('',*,*,#14269,.F.);
#18519=ORIENTED_EDGE('',*,*,#14270,.F.);
#18520=ORIENTED_EDGE('',*,*,#14266,.F.);
#18521=ORIENTED_EDGE('',*,*,#14268,.T.);
#18522=ORIENTED_EDGE('',*,*,#14271,.F.);
#18523=ORIENTED_EDGE('',*,*,#14272,.T.);
#18524=ORIENTED_EDGE('',*,*,#14261,.T.);
#18525=ORIENTED_EDGE('',*,*,#14271,.T.);
#18526=ORIENTED_EDGE('',*,*,#14267,.T.);
#18527=ORIENTED_EDGE('',*,*,#14273,.T.);
#18528=ORIENTED_EDGE('',*,*,#14274,.T.);
#18529=ORIENTED_EDGE('',*,*,#14275,.T.);
#18530=ORIENTED_EDGE('',*,*,#14276,.T.);
#18531=ORIENTED_EDGE('',*,*,#14273,.F.);
#18532=ORIENTED_EDGE('',*,*,#14270,.T.);
#18533=ORIENTED_EDGE('',*,*,#14272,.F.);
#18534=ORIENTED_EDGE('',*,*,#14274,.F.);
#18535=ORIENTED_EDGE('',*,*,#14277,.T.);
#18536=ORIENTED_EDGE('',*,*,#14278,.T.);
#18537=ORIENTED_EDGE('',*,*,#14262,.T.);
#18538=ORIENTED_EDGE('',*,*,#14276,.F.);
#18539=ORIENTED_EDGE('',*,*,#14279,.F.);
#18540=ORIENTED_EDGE('',*,*,#14280,.F.);
#18541=ORIENTED_EDGE('',*,*,#14277,.F.);
#18542=ORIENTED_EDGE('',*,*,#14281,.T.);
#18543=ORIENTED_EDGE('',*,*,#14282,.F.);
#18544=ORIENTED_EDGE('',*,*,#14283,.T.);
#18545=ORIENTED_EDGE('',*,*,#14284,.T.);
#18546=ORIENTED_EDGE('',*,*,#14282,.T.);
#18547=ORIENTED_EDGE('',*,*,#14285,.T.);
#18548=ORIENTED_EDGE('',*,*,#14286,.T.);
#18549=ORIENTED_EDGE('',*,*,#14287,.T.);
#18550=ORIENTED_EDGE('',*,*,#14288,.T.);
#18551=ORIENTED_EDGE('',*,*,#14289,.T.);
#18552=ORIENTED_EDGE('',*,*,#14286,.F.);
#18553=ORIENTED_EDGE('',*,*,#14290,.T.);
#18554=ORIENTED_EDGE('',*,*,#14284,.F.);
#18555=ORIENTED_EDGE('',*,*,#14291,.F.);
#18556=ORIENTED_EDGE('',*,*,#14292,.F.);
#18557=ORIENTED_EDGE('',*,*,#14293,.F.);
#18558=ORIENTED_EDGE('',*,*,#14294,.F.);
#18559=ORIENTED_EDGE('',*,*,#14283,.F.);
#18560=ORIENTED_EDGE('',*,*,#14287,.F.);
#18561=ORIENTED_EDGE('',*,*,#14295,.T.);
#18562=ORIENTED_EDGE('',*,*,#14296,.T.);
#18563=ORIENTED_EDGE('',*,*,#14291,.T.);
#18564=ORIENTED_EDGE('',*,*,#14289,.F.);
#18565=ORIENTED_EDGE('',*,*,#14297,.F.);
#18566=ORIENTED_EDGE('',*,*,#14298,.F.);
#18567=ORIENTED_EDGE('',*,*,#14295,.F.);
#18568=ORIENTED_EDGE('',*,*,#14299,.T.);
#18569=ORIENTED_EDGE('',*,*,#14300,.F.);
#18570=ORIENTED_EDGE('',*,*,#14301,.T.);
#18571=ORIENTED_EDGE('',*,*,#14302,.T.);
#18572=ORIENTED_EDGE('',*,*,#14300,.T.);
#18573=ORIENTED_EDGE('',*,*,#14303,.T.);
#18574=ORIENTED_EDGE('',*,*,#14304,.T.);
#18575=ORIENTED_EDGE('',*,*,#14305,.T.);
#18576=ORIENTED_EDGE('',*,*,#14306,.T.);
#18577=ORIENTED_EDGE('',*,*,#14307,.T.);
#18578=ORIENTED_EDGE('',*,*,#14304,.F.);
#18579=ORIENTED_EDGE('',*,*,#14308,.T.);
#18580=ORIENTED_EDGE('',*,*,#14302,.F.);
#18581=ORIENTED_EDGE('',*,*,#14309,.F.);
#18582=ORIENTED_EDGE('',*,*,#14310,.F.);
#18583=ORIENTED_EDGE('',*,*,#14311,.F.);
#18584=ORIENTED_EDGE('',*,*,#14312,.F.);
#18585=ORIENTED_EDGE('',*,*,#14313,.F.);
#18586=ORIENTED_EDGE('',*,*,#14301,.F.);
#18587=ORIENTED_EDGE('',*,*,#14305,.F.);
#18588=ORIENTED_EDGE('',*,*,#14314,.T.);
#18589=ORIENTED_EDGE('',*,*,#14315,.F.);
#18590=ORIENTED_EDGE('',*,*,#14316,.F.);
#18591=ORIENTED_EDGE('',*,*,#14309,.T.);
#18592=ORIENTED_EDGE('',*,*,#14307,.F.);
#18593=ORIENTED_EDGE('',*,*,#14317,.F.);
#18594=ORIENTED_EDGE('',*,*,#14318,.F.);
#18595=ORIENTED_EDGE('',*,*,#14314,.F.);
#18596=ORIENTED_EDGE('',*,*,#14316,.T.);
#18597=ORIENTED_EDGE('',*,*,#14319,.F.);
#18598=ORIENTED_EDGE('',*,*,#14320,.T.);
#18599=ORIENTED_EDGE('',*,*,#14310,.T.);
#18600=ORIENTED_EDGE('',*,*,#14319,.T.);
#18601=ORIENTED_EDGE('',*,*,#14315,.T.);
#18602=ORIENTED_EDGE('',*,*,#14321,.T.);
#18603=ORIENTED_EDGE('',*,*,#14322,.T.);
#18604=ORIENTED_EDGE('',*,*,#14323,.T.);
#18605=ORIENTED_EDGE('',*,*,#14324,.T.);
#18606=ORIENTED_EDGE('',*,*,#14321,.F.);
#18607=ORIENTED_EDGE('',*,*,#14318,.T.);
#18608=ORIENTED_EDGE('',*,*,#14320,.F.);
#18609=ORIENTED_EDGE('',*,*,#14322,.F.);
#18610=ORIENTED_EDGE('',*,*,#14325,.T.);
#18611=ORIENTED_EDGE('',*,*,#14326,.T.);
#18612=ORIENTED_EDGE('',*,*,#14311,.T.);
#18613=ORIENTED_EDGE('',*,*,#14324,.F.);
#18614=ORIENTED_EDGE('',*,*,#14327,.F.);
#18615=ORIENTED_EDGE('',*,*,#14328,.F.);
#18616=ORIENTED_EDGE('',*,*,#14325,.F.);
#18617=ORIENTED_EDGE('',*,*,#14329,.T.);
#18618=ORIENTED_EDGE('',*,*,#14330,.F.);
#18619=ORIENTED_EDGE('',*,*,#14331,.T.);
#18620=ORIENTED_EDGE('',*,*,#14332,.T.);
#18621=ORIENTED_EDGE('',*,*,#14330,.T.);
#18622=ORIENTED_EDGE('',*,*,#14333,.T.);
#18623=ORIENTED_EDGE('',*,*,#14334,.T.);
#18624=ORIENTED_EDGE('',*,*,#14335,.T.);
#18625=ORIENTED_EDGE('',*,*,#14336,.T.);
#18626=ORIENTED_EDGE('',*,*,#14337,.T.);
#18627=ORIENTED_EDGE('',*,*,#14334,.F.);
#18628=ORIENTED_EDGE('',*,*,#14338,.T.);
#18629=ORIENTED_EDGE('',*,*,#14332,.F.);
#18630=ORIENTED_EDGE('',*,*,#14339,.F.);
#18631=ORIENTED_EDGE('',*,*,#14340,.F.);
#18632=ORIENTED_EDGE('',*,*,#14341,.F.);
#18633=ORIENTED_EDGE('',*,*,#14342,.F.);
#18634=ORIENTED_EDGE('',*,*,#14343,.F.);
#18635=ORIENTED_EDGE('',*,*,#14331,.F.);
#18636=ORIENTED_EDGE('',*,*,#14335,.F.);
#18637=ORIENTED_EDGE('',*,*,#14344,.T.);
#18638=ORIENTED_EDGE('',*,*,#14345,.F.);
#18639=ORIENTED_EDGE('',*,*,#14346,.F.);
#18640=ORIENTED_EDGE('',*,*,#14339,.T.);
#18641=ORIENTED_EDGE('',*,*,#14337,.F.);
#18642=ORIENTED_EDGE('',*,*,#14347,.F.);
#18643=ORIENTED_EDGE('',*,*,#14348,.F.);
#18644=ORIENTED_EDGE('',*,*,#14344,.F.);
#18645=ORIENTED_EDGE('',*,*,#14346,.T.);
#18646=ORIENTED_EDGE('',*,*,#14349,.F.);
#18647=ORIENTED_EDGE('',*,*,#14350,.T.);
#18648=ORIENTED_EDGE('',*,*,#14340,.T.);
#18649=ORIENTED_EDGE('',*,*,#14349,.T.);
#18650=ORIENTED_EDGE('',*,*,#14345,.T.);
#18651=ORIENTED_EDGE('',*,*,#14351,.T.);
#18652=ORIENTED_EDGE('',*,*,#14352,.T.);
#18653=ORIENTED_EDGE('',*,*,#14353,.T.);
#18654=ORIENTED_EDGE('',*,*,#14354,.T.);
#18655=ORIENTED_EDGE('',*,*,#14351,.F.);
#18656=ORIENTED_EDGE('',*,*,#14348,.T.);
#18657=ORIENTED_EDGE('',*,*,#14350,.F.);
#18658=ORIENTED_EDGE('',*,*,#14352,.F.);
#18659=ORIENTED_EDGE('',*,*,#14355,.T.);
#18660=ORIENTED_EDGE('',*,*,#14356,.T.);
#18661=ORIENTED_EDGE('',*,*,#14341,.T.);
#18662=ORIENTED_EDGE('',*,*,#14354,.F.);
#18663=ORIENTED_EDGE('',*,*,#14357,.F.);
#18664=ORIENTED_EDGE('',*,*,#14358,.F.);
#18665=ORIENTED_EDGE('',*,*,#14355,.F.);
#18666=ORIENTED_EDGE('',*,*,#14359,.T.);
#18667=ORIENTED_EDGE('',*,*,#14360,.T.);
#18668=ORIENTED_EDGE('',*,*,#14361,.T.);
#18669=ORIENTED_EDGE('',*,*,#14360,.F.);
#18670=ORIENTED_EDGE('',*,*,#14361,.F.);
#18671=ORIENTED_EDGE('',*,*,#14362,.T.);
#18672=ORIENTED_EDGE('',*,*,#14363,.F.);
#18673=ORIENTED_EDGE('',*,*,#14362,.F.);
#18674=ORIENTED_EDGE('',*,*,#14364,.F.);
#18675=ORIENTED_EDGE('',*,*,#14365,.T.);
#18676=ORIENTED_EDGE('',*,*,#14359,.F.);
#18677=ORIENTED_EDGE('',*,*,#14365,.F.);
#18678=ORIENTED_EDGE('',*,*,#14363,.T.);
#18679=ORIENTED_EDGE('',*,*,#14366,.T.);
#18680=ORIENTED_EDGE('',*,*,#14367,.T.);
#18681=ORIENTED_EDGE('',*,*,#14366,.F.);
#18682=ORIENTED_EDGE('',*,*,#14367,.F.);
#18683=ORIENTED_EDGE('',*,*,#14368,.T.);
#18684=ORIENTED_EDGE('',*,*,#14369,.T.);
#18685=ORIENTED_EDGE('',*,*,#14370,.T.);
#18686=ORIENTED_EDGE('',*,*,#14371,.T.);
#18687=ORIENTED_EDGE('',*,*,#14372,.T.);
#18688=ORIENTED_EDGE('',*,*,#14373,.T.);
#18689=ORIENTED_EDGE('',*,*,#14374,.T.);
#18690=ORIENTED_EDGE('',*,*,#14375,.T.);
#18691=ORIENTED_EDGE('',*,*,#14376,.T.);
#18692=ORIENTED_EDGE('',*,*,#14377,.T.);
#18693=ORIENTED_EDGE('',*,*,#14378,.T.);
#18694=ORIENTED_EDGE('',*,*,#14379,.F.);
#18695=ORIENTED_EDGE('',*,*,#14297,.T.);
#18696=ORIENTED_EDGE('',*,*,#14288,.F.);
#18697=ORIENTED_EDGE('',*,*,#14380,.T.);
#18698=ORIENTED_EDGE('',*,*,#14381,.T.);
#18699=ORIENTED_EDGE('',*,*,#14327,.T.);
#18700=ORIENTED_EDGE('',*,*,#14323,.F.);
#18701=ORIENTED_EDGE('',*,*,#14317,.T.);
#18702=ORIENTED_EDGE('',*,*,#14306,.F.);
#18703=ORIENTED_EDGE('',*,*,#14382,.T.);
#18704=ORIENTED_EDGE('',*,*,#14383,.T.);
#18705=ORIENTED_EDGE('',*,*,#14357,.T.);
#18706=ORIENTED_EDGE('',*,*,#14353,.F.);
#18707=ORIENTED_EDGE('',*,*,#14347,.T.);
#18708=ORIENTED_EDGE('',*,*,#14336,.F.);
#18709=ORIENTED_EDGE('',*,*,#14384,.T.);
#18710=ORIENTED_EDGE('',*,*,#14385,.T.);
#18711=ORIENTED_EDGE('',*,*,#14279,.T.);
#18712=ORIENTED_EDGE('',*,*,#14275,.F.);
#18713=ORIENTED_EDGE('',*,*,#14269,.T.);
#18714=ORIENTED_EDGE('',*,*,#14257,.F.);
#18715=ORIENTED_EDGE('',*,*,#14329,.F.);
#18716=ORIENTED_EDGE('',*,*,#14343,.T.);
#18717=ORIENTED_EDGE('',*,*,#14386,.T.);
#18718=ORIENTED_EDGE('',*,*,#14387,.T.);
#18719=ORIENTED_EDGE('',*,*,#14333,.F.);
#18720=ORIENTED_EDGE('',*,*,#14338,.F.);
#18721=ORIENTED_EDGE('',*,*,#14387,.F.);
#18722=ORIENTED_EDGE('',*,*,#14388,.F.);
#18723=ORIENTED_EDGE('',*,*,#14384,.F.);
#18724=ORIENTED_EDGE('',*,*,#14299,.F.);
#18725=ORIENTED_EDGE('',*,*,#14313,.T.);
#18726=ORIENTED_EDGE('',*,*,#14389,.T.);
#18727=ORIENTED_EDGE('',*,*,#14390,.T.);
#18728=ORIENTED_EDGE('',*,*,#14303,.F.);
#18729=ORIENTED_EDGE('',*,*,#14308,.F.);
#18730=ORIENTED_EDGE('',*,*,#14390,.F.);
#18731=ORIENTED_EDGE('',*,*,#14391,.F.);
#18732=ORIENTED_EDGE('',*,*,#14382,.F.);
#18733=ORIENTED_EDGE('',*,*,#14392,.T.);
#18734=ORIENTED_EDGE('',*,*,#14393,.T.);
#18735=ORIENTED_EDGE('',*,*,#14364,.T.);
#18736=ORIENTED_EDGE('',*,*,#14393,.F.);
#18737=ORIENTED_EDGE('',*,*,#14392,.F.);
#18738=ORIENTED_EDGE('',*,*,#14394,.F.);
#18739=ORIENTED_EDGE('',*,*,#14395,.T.);
#18740=ORIENTED_EDGE('',*,*,#14396,.T.);
#18741=ORIENTED_EDGE('',*,*,#14397,.F.);
#18742=ORIENTED_EDGE('',*,*,#14398,.T.);
#18743=ORIENTED_EDGE('',*,*,#14399,.T.);
#18744=ORIENTED_EDGE('',*,*,#14400,.F.);
#18745=ORIENTED_EDGE('',*,*,#14401,.T.);
#18746=ORIENTED_EDGE('',*,*,#14402,.T.);
#18747=ORIENTED_EDGE('',*,*,#14403,.F.);
#18748=ORIENTED_EDGE('',*,*,#14404,.T.);
#18749=ORIENTED_EDGE('',*,*,#14405,.T.);
#18750=ORIENTED_EDGE('',*,*,#14406,.F.);
#18751=ORIENTED_EDGE('',*,*,#14407,.T.);
#18752=ORIENTED_EDGE('',*,*,#14408,.T.);
#18753=ORIENTED_EDGE('',*,*,#14409,.F.);
#18754=ORIENTED_EDGE('',*,*,#14410,.T.);
#18755=ORIENTED_EDGE('',*,*,#14411,.T.);
#18756=ORIENTED_EDGE('',*,*,#14412,.F.);
#18757=ORIENTED_EDGE('',*,*,#14413,.F.);
#18758=ORIENTED_EDGE('',*,*,#14414,.T.);
#18759=ORIENTED_EDGE('',*,*,#14415,.T.);
#18760=ORIENTED_EDGE('',*,*,#14416,.F.);
#18761=ORIENTED_EDGE('',*,*,#14417,.T.);
#18762=ORIENTED_EDGE('',*,*,#14418,.T.);
#18763=ORIENTED_EDGE('',*,*,#14419,.T.);
#18764=ORIENTED_EDGE('',*,*,#14420,.T.);
#18765=ORIENTED_EDGE('',*,*,#14421,.T.);
#18766=ORIENTED_EDGE('',*,*,#14420,.F.);
#18767=ORIENTED_EDGE('',*,*,#14422,.F.);
#18768=ORIENTED_EDGE('',*,*,#14423,.T.);
#18769=ORIENTED_EDGE('',*,*,#14419,.F.);
#18770=ORIENTED_EDGE('',*,*,#14423,.F.);
#18771=ORIENTED_EDGE('',*,*,#14421,.F.);
#18772=ORIENTED_EDGE('',*,*,#14424,.T.);
#18773=ORIENTED_EDGE('',*,*,#14425,.T.);
#18774=ORIENTED_EDGE('',*,*,#14426,.T.);
#18775=ORIENTED_EDGE('',*,*,#14427,.T.);
#18776=ORIENTED_EDGE('',*,*,#14428,.T.);
#18777=ORIENTED_EDGE('',*,*,#14429,.T.);
#18778=ORIENTED_EDGE('',*,*,#14430,.T.);
#18779=ORIENTED_EDGE('',*,*,#14431,.T.);
#18780=ORIENTED_EDGE('',*,*,#14432,.T.);
#18781=ORIENTED_EDGE('',*,*,#14433,.T.);
#18782=ORIENTED_EDGE('',*,*,#14434,.T.);
#18783=ORIENTED_EDGE('',*,*,#14435,.T.);
#18784=ORIENTED_EDGE('',*,*,#14436,.T.);
#18785=ORIENTED_EDGE('',*,*,#14437,.T.);
#18786=ORIENTED_EDGE('',*,*,#14438,.T.);
#18787=ORIENTED_EDGE('',*,*,#14439,.T.);
#18788=ORIENTED_EDGE('',*,*,#14440,.T.);
#18789=ORIENTED_EDGE('',*,*,#14441,.T.);
#18790=ORIENTED_EDGE('',*,*,#14442,.T.);
#18791=ORIENTED_EDGE('',*,*,#14443,.T.);
#18792=ORIENTED_EDGE('',*,*,#14444,.T.);
#18793=ORIENTED_EDGE('',*,*,#14445,.T.);
#18794=ORIENTED_EDGE('',*,*,#14446,.T.);
#18795=ORIENTED_EDGE('',*,*,#14447,.T.);
#18796=ORIENTED_EDGE('',*,*,#14448,.T.);
#18797=ORIENTED_EDGE('',*,*,#14449,.T.);
#18798=ORIENTED_EDGE('',*,*,#14450,.T.);
#18799=ORIENTED_EDGE('',*,*,#14451,.T.);
#18800=ORIENTED_EDGE('',*,*,#14452,.T.);
#18801=ORIENTED_EDGE('',*,*,#14453,.T.);
#18802=ORIENTED_EDGE('',*,*,#14454,.T.);
#18803=ORIENTED_EDGE('',*,*,#14455,.T.);
#18804=ORIENTED_EDGE('',*,*,#14456,.T.);
#18805=ORIENTED_EDGE('',*,*,#14457,.T.);
#18806=ORIENTED_EDGE('',*,*,#14458,.T.);
#18807=ORIENTED_EDGE('',*,*,#14459,.T.);
#18808=ORIENTED_EDGE('',*,*,#14460,.T.);
#18809=ORIENTED_EDGE('',*,*,#14461,.T.);
#18810=ORIENTED_EDGE('',*,*,#14462,.T.);
#18811=ORIENTED_EDGE('',*,*,#14463,.T.);
#18812=ORIENTED_EDGE('',*,*,#14464,.T.);
#18813=ORIENTED_EDGE('',*,*,#14465,.T.);
#18814=ORIENTED_EDGE('',*,*,#14466,.T.);
#18815=ORIENTED_EDGE('',*,*,#14467,.T.);
#18816=ORIENTED_EDGE('',*,*,#14468,.T.);
#18817=ORIENTED_EDGE('',*,*,#14469,.T.);
#18818=ORIENTED_EDGE('',*,*,#14470,.T.);
#18819=ORIENTED_EDGE('',*,*,#14471,.T.);
#18820=ORIENTED_EDGE('',*,*,#14472,.T.);
#18821=ORIENTED_EDGE('',*,*,#14473,.T.);
#18822=ORIENTED_EDGE('',*,*,#14474,.T.);
#18823=ORIENTED_EDGE('',*,*,#14475,.T.);
#18824=ORIENTED_EDGE('',*,*,#14476,.T.);
#18825=ORIENTED_EDGE('',*,*,#14477,.T.);
#18826=ORIENTED_EDGE('',*,*,#14478,.T.);
#18827=ORIENTED_EDGE('',*,*,#14479,.T.);
#18828=ORIENTED_EDGE('',*,*,#14480,.F.);
#18829=ORIENTED_EDGE('',*,*,#14481,.F.);
#18830=ORIENTED_EDGE('',*,*,#14482,.T.);
#18831=ORIENTED_EDGE('',*,*,#14483,.T.);
#18832=ORIENTED_EDGE('',*,*,#14484,.T.);
#18833=ORIENTED_EDGE('',*,*,#14485,.T.);
#18834=ORIENTED_EDGE('',*,*,#14486,.T.);
#18835=ORIENTED_EDGE('',*,*,#14487,.T.);
#18836=ORIENTED_EDGE('',*,*,#14488,.T.);
#18837=ORIENTED_EDGE('',*,*,#14489,.T.);
#18838=ORIENTED_EDGE('',*,*,#14490,.T.);
#18839=ORIENTED_EDGE('',*,*,#14491,.T.);
#18840=ORIENTED_EDGE('',*,*,#14492,.T.);
#18841=ORIENTED_EDGE('',*,*,#14493,.T.);
#18842=ORIENTED_EDGE('',*,*,#14494,.F.);
#18843=ORIENTED_EDGE('',*,*,#14495,.F.);
#18844=ORIENTED_EDGE('',*,*,#14496,.T.);
#18845=ORIENTED_EDGE('',*,*,#14497,.T.);
#18846=ORIENTED_EDGE('',*,*,#14498,.T.);
#18847=ORIENTED_EDGE('',*,*,#14499,.T.);
#18848=ORIENTED_EDGE('',*,*,#14500,.T.);
#18849=ORIENTED_EDGE('',*,*,#14501,.T.);
#18850=ORIENTED_EDGE('',*,*,#14502,.T.);
#18851=ORIENTED_EDGE('',*,*,#14503,.T.);
#18852=ORIENTED_EDGE('',*,*,#14504,.T.);
#18853=ORIENTED_EDGE('',*,*,#14505,.F.);
#18854=ORIENTED_EDGE('',*,*,#14506,.F.);
#18855=ORIENTED_EDGE('',*,*,#14507,.F.);
#18856=ORIENTED_EDGE('',*,*,#14508,.T.);
#18857=ORIENTED_EDGE('',*,*,#14509,.T.);
#18858=ORIENTED_EDGE('',*,*,#14510,.T.);
#18859=ORIENTED_EDGE('',*,*,#14511,.T.);
#18860=ORIENTED_EDGE('',*,*,#14512,.T.);
#18861=ORIENTED_EDGE('',*,*,#14513,.T.);
#18862=ORIENTED_EDGE('',*,*,#14514,.T.);
#18863=ORIENTED_EDGE('',*,*,#14515,.T.);
#18864=ORIENTED_EDGE('',*,*,#14516,.T.);
#18865=ORIENTED_EDGE('',*,*,#14517,.T.);
#18866=ORIENTED_EDGE('',*,*,#14518,.T.);
#18867=ORIENTED_EDGE('',*,*,#14519,.T.);
#18868=ORIENTED_EDGE('',*,*,#14520,.F.);
#18869=ORIENTED_EDGE('',*,*,#14521,.F.);
#18870=ORIENTED_EDGE('',*,*,#14281,.F.);
#18871=ORIENTED_EDGE('',*,*,#14294,.T.);
#18872=ORIENTED_EDGE('',*,*,#14522,.T.);
#18873=ORIENTED_EDGE('',*,*,#14523,.T.);
#18874=ORIENTED_EDGE('',*,*,#14285,.F.);
#18875=ORIENTED_EDGE('',*,*,#14524,.T.);
#18876=ORIENTED_EDGE('',*,*,#14298,.T.);
#18877=ORIENTED_EDGE('',*,*,#14379,.T.);
#18878=ORIENTED_EDGE('',*,*,#14525,.T.);
#18879=ORIENTED_EDGE('',*,*,#14524,.F.);
#18880=ORIENTED_EDGE('',*,*,#14526,.T.);
#18881=ORIENTED_EDGE('',*,*,#14296,.F.);
#18882=ORIENTED_EDGE('',*,*,#14526,.F.);
#18883=ORIENTED_EDGE('',*,*,#14527,.T.);
#18884=ORIENTED_EDGE('',*,*,#14528,.T.);
#18885=ORIENTED_EDGE('',*,*,#14292,.T.);
#18886=ORIENTED_EDGE('',*,*,#14525,.F.);
#18887=ORIENTED_EDGE('',*,*,#14378,.F.);
#18888=ORIENTED_EDGE('',*,*,#14529,.F.);
#18889=ORIENTED_EDGE('',*,*,#14527,.F.);
#18890=ORIENTED_EDGE('',*,*,#14530,.T.);
#18891=ORIENTED_EDGE('',*,*,#14531,.T.);
#18892=ORIENTED_EDGE('',*,*,#14422,.T.);
#18893=ORIENTED_EDGE('',*,*,#14531,.F.);
#18894=ORIENTED_EDGE('',*,*,#14532,.T.);
#18895=ORIENTED_EDGE('',*,*,#14533,.F.);
#18896=ORIENTED_EDGE('',*,*,#14264,.T.);
#18897=ORIENTED_EDGE('',*,*,#14534,.T.);
#18898=ORIENTED_EDGE('',*,*,#14530,.F.);
#18899=ORIENTED_EDGE('',*,*,#14534,.F.);
#18900=ORIENTED_EDGE('',*,*,#14263,.T.);
#18901=ORIENTED_EDGE('',*,*,#14278,.F.);
#18902=ORIENTED_EDGE('',*,*,#14280,.T.);
#18903=ORIENTED_EDGE('',*,*,#14385,.F.);
#18904=ORIENTED_EDGE('',*,*,#14388,.T.);
#18905=ORIENTED_EDGE('',*,*,#14386,.F.);
#18906=ORIENTED_EDGE('',*,*,#14342,.T.);
#18907=ORIENTED_EDGE('',*,*,#14356,.F.);
#18908=ORIENTED_EDGE('',*,*,#14358,.T.);
#18909=ORIENTED_EDGE('',*,*,#14383,.F.);
#18910=ORIENTED_EDGE('',*,*,#14391,.T.);
#18911=ORIENTED_EDGE('',*,*,#14389,.F.);
#18912=ORIENTED_EDGE('',*,*,#14312,.T.);
#18913=ORIENTED_EDGE('',*,*,#14326,.F.);
#18914=ORIENTED_EDGE('',*,*,#14328,.T.);
#18915=ORIENTED_EDGE('',*,*,#14381,.F.);
#18916=ORIENTED_EDGE('',*,*,#14535,.T.);
#18917=ORIENTED_EDGE('',*,*,#14522,.F.);
#18918=ORIENTED_EDGE('',*,*,#14293,.T.);
#18919=ORIENTED_EDGE('',*,*,#14528,.F.);
#18920=ORIENTED_EDGE('',*,*,#14529,.T.);
#18921=ORIENTED_EDGE('',*,*,#14377,.F.);
#18922=ORIENTED_EDGE('',*,*,#14250,.F.);
#18923=ORIENTED_EDGE('',*,*,#14265,.T.);
#18924=ORIENTED_EDGE('',*,*,#14533,.T.);
#18925=ORIENTED_EDGE('',*,*,#14536,.T.);
#18926=ORIENTED_EDGE('',*,*,#14254,.F.);
#18927=ORIENTED_EDGE('',*,*,#14259,.F.);
#18928=ORIENTED_EDGE('',*,*,#14536,.F.);
#18929=ORIENTED_EDGE('',*,*,#14532,.F.);
#18930=ORIENTED_EDGE('',*,*,#14376,.F.);
#18931=ORIENTED_EDGE('',*,*,#14537,.T.);
#18932=ORIENTED_EDGE('',*,*,#14538,.T.);
#18933=ORIENTED_EDGE('',*,*,#14539,.T.);
#18934=ORIENTED_EDGE('',*,*,#14540,.T.);
#18935=ORIENTED_EDGE('',*,*,#14541,.T.);
#18936=ORIENTED_EDGE('',*,*,#14542,.T.);
#18937=ORIENTED_EDGE('',*,*,#14543,.T.);
#18938=ORIENTED_EDGE('',*,*,#14538,.F.);
#18939=ORIENTED_EDGE('',*,*,#14544,.T.);
#18940=ORIENTED_EDGE('',*,*,#14545,.T.);
#18941=ORIENTED_EDGE('',*,*,#14546,.T.);
#18942=ORIENTED_EDGE('',*,*,#14540,.F.);
#18943=ORIENTED_EDGE('',*,*,#14541,.F.);
#18944=ORIENTED_EDGE('',*,*,#14537,.F.);
#18945=ORIENTED_EDGE('',*,*,#14546,.F.);
#18946=ORIENTED_EDGE('',*,*,#14547,.T.);
#18947=ORIENTED_EDGE('',*,*,#14548,.T.);
#18948=ORIENTED_EDGE('',*,*,#14549,.T.);
#18949=ORIENTED_EDGE('',*,*,#14550,.T.);
#18950=ORIENTED_EDGE('',*,*,#14551,.T.);
#18951=ORIENTED_EDGE('',*,*,#14550,.F.);
#18952=ORIENTED_EDGE('',*,*,#14545,.F.);
#18953=ORIENTED_EDGE('',*,*,#14552,.T.);
#18954=ORIENTED_EDGE('',*,*,#14553,.T.);
#18955=ORIENTED_EDGE('',*,*,#14554,.T.);
#18956=ORIENTED_EDGE('',*,*,#14548,.F.);
#18957=ORIENTED_EDGE('',*,*,#14549,.F.);
#18958=ORIENTED_EDGE('',*,*,#14554,.F.);
#18959=ORIENTED_EDGE('',*,*,#14555,.T.);
#18960=ORIENTED_EDGE('',*,*,#14556,.F.);
#18961=ORIENTED_EDGE('',*,*,#14542,.F.);
#18962=ORIENTED_EDGE('',*,*,#14547,.F.);
#18963=ORIENTED_EDGE('',*,*,#14557,.T.);
#18964=ORIENTED_EDGE('',*,*,#14400,.T.);
#18965=ORIENTED_EDGE('',*,*,#14558,.T.);
#18966=ORIENTED_EDGE('',*,*,#14397,.T.);
#18967=ORIENTED_EDGE('',*,*,#14559,.T.);
#18968=ORIENTED_EDGE('',*,*,#14394,.T.);
#18969=ORIENTED_EDGE('',*,*,#14560,.T.);
#18970=ORIENTED_EDGE('',*,*,#14416,.T.);
#18971=ORIENTED_EDGE('',*,*,#14561,.T.);
#18972=ORIENTED_EDGE('',*,*,#14413,.T.);
#18973=ORIENTED_EDGE('',*,*,#14562,.T.);
#18974=ORIENTED_EDGE('',*,*,#14563,.T.);
#18975=ORIENTED_EDGE('',*,*,#14564,.T.);
#18976=ORIENTED_EDGE('',*,*,#14562,.F.);
#18977=ORIENTED_EDGE('',*,*,#14412,.T.);
#18978=ORIENTED_EDGE('',*,*,#14565,.T.);
#18979=ORIENTED_EDGE('',*,*,#14409,.T.);
#18980=ORIENTED_EDGE('',*,*,#14566,.T.);
#18981=ORIENTED_EDGE('',*,*,#14406,.T.);
#18982=ORIENTED_EDGE('',*,*,#14567,.T.);
#18983=ORIENTED_EDGE('',*,*,#14403,.T.);
#18984=ORIENTED_EDGE('',*,*,#14369,.F.);
#18985=ORIENTED_EDGE('',*,*,#14568,.T.);
#18986=ORIENTED_EDGE('',*,*,#14395,.F.);
#18987=ORIENTED_EDGE('',*,*,#14559,.F.);
#18988=ORIENTED_EDGE('',*,*,#14396,.F.);
#18989=ORIENTED_EDGE('',*,*,#14568,.F.);
#18990=ORIENTED_EDGE('',*,*,#14374,.F.);
#18991=ORIENTED_EDGE('',*,*,#14569,.T.);
#18992=ORIENTED_EDGE('',*,*,#14398,.F.);
#18993=ORIENTED_EDGE('',*,*,#14558,.F.);
#18994=ORIENTED_EDGE('',*,*,#14399,.F.);
#18995=ORIENTED_EDGE('',*,*,#14569,.F.);
#18996=ORIENTED_EDGE('',*,*,#14368,.F.);
#18997=ORIENTED_EDGE('',*,*,#14570,.T.);
#18998=ORIENTED_EDGE('',*,*,#14401,.F.);
#18999=ORIENTED_EDGE('',*,*,#14557,.F.);
#19000=ORIENTED_EDGE('',*,*,#14402,.F.);
#19001=ORIENTED_EDGE('',*,*,#14570,.F.);
#19002=ORIENTED_EDGE('',*,*,#14375,.F.);
#19003=ORIENTED_EDGE('',*,*,#14571,.T.);
#19004=ORIENTED_EDGE('',*,*,#14404,.F.);
#19005=ORIENTED_EDGE('',*,*,#14567,.F.);
#19006=ORIENTED_EDGE('',*,*,#14405,.F.);
#19007=ORIENTED_EDGE('',*,*,#14571,.F.);
#19008=ORIENTED_EDGE('',*,*,#14572,.F.);
#19009=ORIENTED_EDGE('',*,*,#14573,.T.);
#19010=ORIENTED_EDGE('',*,*,#14563,.F.);
#19011=ORIENTED_EDGE('',*,*,#14564,.F.);
#19012=ORIENTED_EDGE('',*,*,#14573,.F.);
#19013=ORIENTED_EDGE('',*,*,#14574,.F.);
#19014=ORIENTED_EDGE('',*,*,#14521,.T.);
#19015=ORIENTED_EDGE('',*,*,#14575,.T.);
#19016=ORIENTED_EDGE('',*,*,#14576,.T.);
#19017=ORIENTED_EDGE('',*,*,#14577,.F.);
#19018=ORIENTED_EDGE('',*,*,#14495,.T.);
#19019=ORIENTED_EDGE('',*,*,#14578,.T.);
#19020=ORIENTED_EDGE('',*,*,#14579,.T.);
#19021=ORIENTED_EDGE('',*,*,#14580,.F.);
#19022=ORIENTED_EDGE('',*,*,#14481,.T.);
#19023=ORIENTED_EDGE('',*,*,#14581,.T.);
#19024=ORIENTED_EDGE('',*,*,#14582,.T.);
#19025=ORIENTED_EDGE('',*,*,#14583,.F.);
#19026=ORIENTED_EDGE('',*,*,#14505,.T.);
#19027=ORIENTED_EDGE('',*,*,#14584,.T.);
#19028=ORIENTED_EDGE('',*,*,#14585,.T.);
#19029=ORIENTED_EDGE('',*,*,#14586,.T.);
#19030=ORIENTED_EDGE('',*,*,#14587,.F.);
#19031=ORIENTED_EDGE('',*,*,#14507,.T.);
#19032=ORIENTED_EDGE('',*,*,#14588,.T.);
#19033=ORIENTED_EDGE('',*,*,#14589,.T.);
#19034=ORIENTED_EDGE('',*,*,#14510,.F.);
#19035=ORIENTED_EDGE('',*,*,#14590,.T.);
#19036=ORIENTED_EDGE('',*,*,#14591,.T.);
#19037=ORIENTED_EDGE('',*,*,#14592,.F.);
#19038=ORIENTED_EDGE('',*,*,#14509,.F.);
#19039=ORIENTED_EDGE('',*,*,#14593,.T.);
#19040=ORIENTED_EDGE('',*,*,#14594,.T.);
#19041=ORIENTED_EDGE('',*,*,#14590,.F.);
#19042=ORIENTED_EDGE('',*,*,#14508,.F.);
#19043=ORIENTED_EDGE('',*,*,#14587,.T.);
#19044=ORIENTED_EDGE('',*,*,#14595,.T.);
#19045=ORIENTED_EDGE('',*,*,#14593,.F.);
#19046=ORIENTED_EDGE('',*,*,#14506,.T.);
#19047=ORIENTED_EDGE('',*,*,#14583,.T.);
#19048=ORIENTED_EDGE('',*,*,#14596,.T.);
#19049=ORIENTED_EDGE('',*,*,#14588,.F.);
#19050=ORIENTED_EDGE('',*,*,#14512,.F.);
#19051=ORIENTED_EDGE('',*,*,#14597,.T.);
#19052=ORIENTED_EDGE('',*,*,#14598,.T.);
#19053=ORIENTED_EDGE('',*,*,#14585,.F.);
#19054=ORIENTED_EDGE('',*,*,#14599,.T.);
#19055=ORIENTED_EDGE('',*,*,#14600,.T.);
#19056=ORIENTED_EDGE('',*,*,#14601,.F.);
#19057=ORIENTED_EDGE('',*,*,#14511,.F.);
#19058=ORIENTED_EDGE('',*,*,#14592,.T.);
#19059=ORIENTED_EDGE('',*,*,#14602,.T.);
#19060=ORIENTED_EDGE('',*,*,#14597,.F.);
#19061=ORIENTED_EDGE('',*,*,#14602,.F.);
#19062=ORIENTED_EDGE('',*,*,#14591,.F.);
#19063=ORIENTED_EDGE('',*,*,#14594,.F.);
#19064=ORIENTED_EDGE('',*,*,#14595,.F.);
#19065=ORIENTED_EDGE('',*,*,#14589,.F.);
#19066=ORIENTED_EDGE('',*,*,#14596,.F.);
#19067=ORIENTED_EDGE('',*,*,#14586,.F.);
#19068=ORIENTED_EDGE('',*,*,#14598,.F.);
#19069=ORIENTED_EDGE('',*,*,#14478,.F.);
#19070=ORIENTED_EDGE('',*,*,#14603,.T.);
#19071=ORIENTED_EDGE('',*,*,#14604,.T.);
#19072=ORIENTED_EDGE('',*,*,#14605,.F.);
#19073=ORIENTED_EDGE('',*,*,#14477,.F.);
#19074=ORIENTED_EDGE('',*,*,#14606,.T.);
#19075=ORIENTED_EDGE('',*,*,#14607,.T.);
#19076=ORIENTED_EDGE('',*,*,#14603,.F.);
#19077=ORIENTED_EDGE('',*,*,#14476,.F.);
#19078=ORIENTED_EDGE('',*,*,#14608,.T.);
#19079=ORIENTED_EDGE('',*,*,#14609,.T.);
#19080=ORIENTED_EDGE('',*,*,#14606,.F.);
#19081=ORIENTED_EDGE('',*,*,#14475,.F.);
#19082=ORIENTED_EDGE('',*,*,#14610,.T.);
#19083=ORIENTED_EDGE('',*,*,#14611,.T.);
#19084=ORIENTED_EDGE('',*,*,#14608,.F.);
#19085=ORIENTED_EDGE('',*,*,#14474,.F.);
#19086=ORIENTED_EDGE('',*,*,#14612,.T.);
#19087=ORIENTED_EDGE('',*,*,#14613,.T.);
#19088=ORIENTED_EDGE('',*,*,#14610,.F.);
#19089=ORIENTED_EDGE('',*,*,#14473,.F.);
#19090=ORIENTED_EDGE('',*,*,#14614,.T.);
#19091=ORIENTED_EDGE('',*,*,#14615,.T.);
#19092=ORIENTED_EDGE('',*,*,#14612,.F.);
#19093=ORIENTED_EDGE('',*,*,#14472,.F.);
#19094=ORIENTED_EDGE('',*,*,#14616,.T.);
#19095=ORIENTED_EDGE('',*,*,#14617,.T.);
#19096=ORIENTED_EDGE('',*,*,#14614,.F.);
#19097=ORIENTED_EDGE('',*,*,#14471,.F.);
#19098=ORIENTED_EDGE('',*,*,#14618,.T.);
#19099=ORIENTED_EDGE('',*,*,#14619,.T.);
#19100=ORIENTED_EDGE('',*,*,#14616,.F.);
#19101=ORIENTED_EDGE('',*,*,#14470,.F.);
#19102=ORIENTED_EDGE('',*,*,#14580,.T.);
#19103=ORIENTED_EDGE('',*,*,#14620,.T.);
#19104=ORIENTED_EDGE('',*,*,#14618,.F.);
#19105=ORIENTED_EDGE('',*,*,#14480,.T.);
#19106=ORIENTED_EDGE('',*,*,#14621,.T.);
#19107=ORIENTED_EDGE('',*,*,#14622,.T.);
#19108=ORIENTED_EDGE('',*,*,#14581,.F.);
#19109=ORIENTED_EDGE('',*,*,#14479,.F.);
#19110=ORIENTED_EDGE('',*,*,#14605,.T.);
#19111=ORIENTED_EDGE('',*,*,#14623,.T.);
#19112=ORIENTED_EDGE('',*,*,#14621,.F.);
#19113=ORIENTED_EDGE('',*,*,#14623,.F.);
#19114=ORIENTED_EDGE('',*,*,#14604,.F.);
#19115=ORIENTED_EDGE('',*,*,#14607,.F.);
#19116=ORIENTED_EDGE('',*,*,#14609,.F.);
#19117=ORIENTED_EDGE('',*,*,#14611,.F.);
#19118=ORIENTED_EDGE('',*,*,#14613,.F.);
#19119=ORIENTED_EDGE('',*,*,#14615,.F.);
#19120=ORIENTED_EDGE('',*,*,#14617,.F.);
#19121=ORIENTED_EDGE('',*,*,#14619,.F.);
#19122=ORIENTED_EDGE('',*,*,#14620,.F.);
#19123=ORIENTED_EDGE('',*,*,#14582,.F.);
#19124=ORIENTED_EDGE('',*,*,#14622,.F.);
#19125=ORIENTED_EDGE('',*,*,#14492,.F.);
#19126=ORIENTED_EDGE('',*,*,#14624,.T.);
#19127=ORIENTED_EDGE('',*,*,#14625,.T.);
#19128=ORIENTED_EDGE('',*,*,#14626,.F.);
#19129=ORIENTED_EDGE('',*,*,#14491,.F.);
#19130=ORIENTED_EDGE('',*,*,#14627,.T.);
#19131=ORIENTED_EDGE('',*,*,#14628,.T.);
#19132=ORIENTED_EDGE('',*,*,#14624,.F.);
#19133=ORIENTED_EDGE('',*,*,#14490,.F.);
#19134=ORIENTED_EDGE('',*,*,#14629,.T.);
#19135=ORIENTED_EDGE('',*,*,#14630,.T.);
#19136=ORIENTED_EDGE('',*,*,#14627,.F.);
#19137=ORIENTED_EDGE('',*,*,#14489,.F.);
#19138=ORIENTED_EDGE('',*,*,#14631,.T.);
#19139=ORIENTED_EDGE('',*,*,#14632,.T.);
#19140=ORIENTED_EDGE('',*,*,#14629,.F.);
#19141=ORIENTED_EDGE('',*,*,#14488,.F.);
#19142=ORIENTED_EDGE('',*,*,#14633,.T.);
#19143=ORIENTED_EDGE('',*,*,#14634,.T.);
#19144=ORIENTED_EDGE('',*,*,#14631,.F.);
#19145=ORIENTED_EDGE('',*,*,#14487,.F.);
#19146=ORIENTED_EDGE('',*,*,#14635,.T.);
#19147=ORIENTED_EDGE('',*,*,#14636,.T.);
#19148=ORIENTED_EDGE('',*,*,#14633,.F.);
#19149=ORIENTED_EDGE('',*,*,#14486,.F.);
#19150=ORIENTED_EDGE('',*,*,#14637,.T.);
#19151=ORIENTED_EDGE('',*,*,#14638,.T.);
#19152=ORIENTED_EDGE('',*,*,#14635,.F.);
#19153=ORIENTED_EDGE('',*,*,#14485,.F.);
#19154=ORIENTED_EDGE('',*,*,#14639,.T.);
#19155=ORIENTED_EDGE('',*,*,#14640,.T.);
#19156=ORIENTED_EDGE('',*,*,#14637,.F.);
#19157=ORIENTED_EDGE('',*,*,#14484,.F.);
#19158=ORIENTED_EDGE('',*,*,#14641,.T.);
#19159=ORIENTED_EDGE('',*,*,#14642,.T.);
#19160=ORIENTED_EDGE('',*,*,#14639,.F.);
#19161=ORIENTED_EDGE('',*,*,#14483,.F.);
#19162=ORIENTED_EDGE('',*,*,#14643,.T.);
#19163=ORIENTED_EDGE('',*,*,#14644,.T.);
#19164=ORIENTED_EDGE('',*,*,#14641,.F.);
#19165=ORIENTED_EDGE('',*,*,#14482,.F.);
#19166=ORIENTED_EDGE('',*,*,#14577,.T.);
#19167=ORIENTED_EDGE('',*,*,#14645,.T.);
#19168=ORIENTED_EDGE('',*,*,#14643,.F.);
#19169=ORIENTED_EDGE('',*,*,#14494,.T.);
#19170=ORIENTED_EDGE('',*,*,#14646,.T.);
#19171=ORIENTED_EDGE('',*,*,#14647,.T.);
#19172=ORIENTED_EDGE('',*,*,#14578,.F.);
#19173=ORIENTED_EDGE('',*,*,#14493,.F.);
#19174=ORIENTED_EDGE('',*,*,#14626,.T.);
#19175=ORIENTED_EDGE('',*,*,#14648,.T.);
#19176=ORIENTED_EDGE('',*,*,#14646,.F.);
#19177=ORIENTED_EDGE('',*,*,#14648,.F.);
#19178=ORIENTED_EDGE('',*,*,#14625,.F.);
#19179=ORIENTED_EDGE('',*,*,#14628,.F.);
#19180=ORIENTED_EDGE('',*,*,#14630,.F.);
#19181=ORIENTED_EDGE('',*,*,#14632,.F.);
#19182=ORIENTED_EDGE('',*,*,#14634,.F.);
#19183=ORIENTED_EDGE('',*,*,#14636,.F.);
#19184=ORIENTED_EDGE('',*,*,#14638,.F.);
#19185=ORIENTED_EDGE('',*,*,#14640,.F.);
#19186=ORIENTED_EDGE('',*,*,#14642,.F.);
#19187=ORIENTED_EDGE('',*,*,#14644,.F.);
#19188=ORIENTED_EDGE('',*,*,#14645,.F.);
#19189=ORIENTED_EDGE('',*,*,#14579,.F.);
#19190=ORIENTED_EDGE('',*,*,#14647,.F.);
#19191=ORIENTED_EDGE('',*,*,#14424,.F.);
#19192=ORIENTED_EDGE('',*,*,#14649,.T.);
#19193=ORIENTED_EDGE('',*,*,#14650,.T.);
#19194=ORIENTED_EDGE('',*,*,#14651,.F.);
#19195=ORIENTED_EDGE('',*,*,#14458,.F.);
#19196=ORIENTED_EDGE('',*,*,#14652,.T.);
#19197=ORIENTED_EDGE('',*,*,#14653,.T.);
#19198=ORIENTED_EDGE('',*,*,#14649,.F.);
#19199=ORIENTED_EDGE('',*,*,#14457,.F.);
#19200=ORIENTED_EDGE('',*,*,#14654,.T.);
#19201=ORIENTED_EDGE('',*,*,#14655,.T.);
#19202=ORIENTED_EDGE('',*,*,#14652,.F.);
#19203=ORIENTED_EDGE('',*,*,#14456,.F.);
#19204=ORIENTED_EDGE('',*,*,#14656,.T.);
#19205=ORIENTED_EDGE('',*,*,#14657,.T.);
#19206=ORIENTED_EDGE('',*,*,#14654,.F.);
#19207=ORIENTED_EDGE('',*,*,#14455,.F.);
#19208=ORIENTED_EDGE('',*,*,#14658,.T.);
#19209=ORIENTED_EDGE('',*,*,#14659,.T.);
#19210=ORIENTED_EDGE('',*,*,#14656,.F.);
#19211=ORIENTED_EDGE('',*,*,#14454,.F.);
#19212=ORIENTED_EDGE('',*,*,#14660,.T.);
#19213=ORIENTED_EDGE('',*,*,#14661,.T.);
#19214=ORIENTED_EDGE('',*,*,#14658,.F.);
#19215=ORIENTED_EDGE('',*,*,#14453,.F.);
#19216=ORIENTED_EDGE('',*,*,#14662,.T.);
#19217=ORIENTED_EDGE('',*,*,#14663,.T.);
#19218=ORIENTED_EDGE('',*,*,#14660,.F.);
#19219=ORIENTED_EDGE('',*,*,#14452,.F.);
#19220=ORIENTED_EDGE('',*,*,#14664,.T.);
#19221=ORIENTED_EDGE('',*,*,#14665,.T.);
#19222=ORIENTED_EDGE('',*,*,#14662,.F.);
#19223=ORIENTED_EDGE('',*,*,#14451,.F.);
#19224=ORIENTED_EDGE('',*,*,#14666,.T.);
#19225=ORIENTED_EDGE('',*,*,#14667,.T.);
#19226=ORIENTED_EDGE('',*,*,#14664,.F.);
#19227=ORIENTED_EDGE('',*,*,#14450,.F.);
#19228=ORIENTED_EDGE('',*,*,#14668,.T.);
#19229=ORIENTED_EDGE('',*,*,#14669,.T.);
#19230=ORIENTED_EDGE('',*,*,#14666,.F.);
#19231=ORIENTED_EDGE('',*,*,#14449,.F.);
#19232=ORIENTED_EDGE('',*,*,#14670,.T.);
#19233=ORIENTED_EDGE('',*,*,#14671,.T.);
#19234=ORIENTED_EDGE('',*,*,#14668,.F.);
#19235=ORIENTED_EDGE('',*,*,#14448,.F.);
#19236=ORIENTED_EDGE('',*,*,#14672,.T.);
#19237=ORIENTED_EDGE('',*,*,#14673,.T.);
#19238=ORIENTED_EDGE('',*,*,#14670,.F.);
#19239=ORIENTED_EDGE('',*,*,#14447,.F.);
#19240=ORIENTED_EDGE('',*,*,#14674,.T.);
#19241=ORIENTED_EDGE('',*,*,#14675,.T.);
#19242=ORIENTED_EDGE('',*,*,#14672,.F.);
#19243=ORIENTED_EDGE('',*,*,#14446,.F.);
#19244=ORIENTED_EDGE('',*,*,#14676,.T.);
#19245=ORIENTED_EDGE('',*,*,#14677,.T.);
#19246=ORIENTED_EDGE('',*,*,#14674,.F.);
#19247=ORIENTED_EDGE('',*,*,#14445,.F.);
#19248=ORIENTED_EDGE('',*,*,#14678,.T.);
#19249=ORIENTED_EDGE('',*,*,#14679,.T.);
#19250=ORIENTED_EDGE('',*,*,#14676,.F.);
#19251=ORIENTED_EDGE('',*,*,#14444,.F.);
#19252=ORIENTED_EDGE('',*,*,#14680,.T.);
#19253=ORIENTED_EDGE('',*,*,#14681,.T.);
#19254=ORIENTED_EDGE('',*,*,#14678,.F.);
#19255=ORIENTED_EDGE('',*,*,#14443,.F.);
#19256=ORIENTED_EDGE('',*,*,#14682,.T.);
#19257=ORIENTED_EDGE('',*,*,#14683,.T.);
#19258=ORIENTED_EDGE('',*,*,#14680,.F.);
#19259=ORIENTED_EDGE('',*,*,#14442,.F.);
#19260=ORIENTED_EDGE('',*,*,#14684,.T.);
#19261=ORIENTED_EDGE('',*,*,#14685,.T.);
#19262=ORIENTED_EDGE('',*,*,#14682,.F.);
#19263=ORIENTED_EDGE('',*,*,#14441,.F.);
#19264=ORIENTED_EDGE('',*,*,#14686,.T.);
#19265=ORIENTED_EDGE('',*,*,#14687,.T.);
#19266=ORIENTED_EDGE('',*,*,#14684,.F.);
#19267=ORIENTED_EDGE('',*,*,#14440,.F.);
#19268=ORIENTED_EDGE('',*,*,#14688,.T.);
#19269=ORIENTED_EDGE('',*,*,#14689,.T.);
#19270=ORIENTED_EDGE('',*,*,#14686,.F.);
#19271=ORIENTED_EDGE('',*,*,#14439,.F.);
#19272=ORIENTED_EDGE('',*,*,#14690,.T.);
#19273=ORIENTED_EDGE('',*,*,#14691,.T.);
#19274=ORIENTED_EDGE('',*,*,#14688,.F.);
#19275=ORIENTED_EDGE('',*,*,#14438,.F.);
#19276=ORIENTED_EDGE('',*,*,#14692,.T.);
#19277=ORIENTED_EDGE('',*,*,#14693,.T.);
#19278=ORIENTED_EDGE('',*,*,#14690,.F.);
#19279=ORIENTED_EDGE('',*,*,#14437,.F.);
#19280=ORIENTED_EDGE('',*,*,#14694,.T.);
#19281=ORIENTED_EDGE('',*,*,#14695,.T.);
#19282=ORIENTED_EDGE('',*,*,#14692,.F.);
#19283=ORIENTED_EDGE('',*,*,#14436,.F.);
#19284=ORIENTED_EDGE('',*,*,#14696,.T.);
#19285=ORIENTED_EDGE('',*,*,#14697,.T.);
#19286=ORIENTED_EDGE('',*,*,#14694,.F.);
#19287=ORIENTED_EDGE('',*,*,#14435,.F.);
#19288=ORIENTED_EDGE('',*,*,#14698,.T.);
#19289=ORIENTED_EDGE('',*,*,#14699,.T.);
#19290=ORIENTED_EDGE('',*,*,#14696,.F.);
#19291=ORIENTED_EDGE('',*,*,#14434,.F.);
#19292=ORIENTED_EDGE('',*,*,#14700,.T.);
#19293=ORIENTED_EDGE('',*,*,#14701,.T.);
#19294=ORIENTED_EDGE('',*,*,#14698,.F.);
#19295=ORIENTED_EDGE('',*,*,#14433,.F.);
#19296=ORIENTED_EDGE('',*,*,#14702,.T.);
#19297=ORIENTED_EDGE('',*,*,#14703,.T.);
#19298=ORIENTED_EDGE('',*,*,#14700,.F.);
#19299=ORIENTED_EDGE('',*,*,#14432,.F.);
#19300=ORIENTED_EDGE('',*,*,#14704,.T.);
#19301=ORIENTED_EDGE('',*,*,#14705,.T.);
#19302=ORIENTED_EDGE('',*,*,#14702,.F.);
#19303=ORIENTED_EDGE('',*,*,#14431,.F.);
#19304=ORIENTED_EDGE('',*,*,#14706,.T.);
#19305=ORIENTED_EDGE('',*,*,#14707,.T.);
#19306=ORIENTED_EDGE('',*,*,#14704,.F.);
#19307=ORIENTED_EDGE('',*,*,#14430,.F.);
#19308=ORIENTED_EDGE('',*,*,#14708,.T.);
#19309=ORIENTED_EDGE('',*,*,#14709,.T.);
#19310=ORIENTED_EDGE('',*,*,#14706,.F.);
#19311=ORIENTED_EDGE('',*,*,#14429,.F.);
#19312=ORIENTED_EDGE('',*,*,#14710,.T.);
#19313=ORIENTED_EDGE('',*,*,#14711,.T.);
#19314=ORIENTED_EDGE('',*,*,#14708,.F.);
#19315=ORIENTED_EDGE('',*,*,#14428,.F.);
#19316=ORIENTED_EDGE('',*,*,#14712,.T.);
#19317=ORIENTED_EDGE('',*,*,#14713,.T.);
#19318=ORIENTED_EDGE('',*,*,#14710,.F.);
#19319=ORIENTED_EDGE('',*,*,#14427,.F.);
#19320=ORIENTED_EDGE('',*,*,#14714,.T.);
#19321=ORIENTED_EDGE('',*,*,#14715,.T.);
#19322=ORIENTED_EDGE('',*,*,#14712,.F.);
#19323=ORIENTED_EDGE('',*,*,#14426,.F.);
#19324=ORIENTED_EDGE('',*,*,#14716,.T.);
#19325=ORIENTED_EDGE('',*,*,#14717,.T.);
#19326=ORIENTED_EDGE('',*,*,#14714,.F.);
#19327=ORIENTED_EDGE('',*,*,#14425,.F.);
#19328=ORIENTED_EDGE('',*,*,#14651,.T.);
#19329=ORIENTED_EDGE('',*,*,#14718,.T.);
#19330=ORIENTED_EDGE('',*,*,#14716,.F.);
#19331=ORIENTED_EDGE('',*,*,#14718,.F.);
#19332=ORIENTED_EDGE('',*,*,#14650,.F.);
#19333=ORIENTED_EDGE('',*,*,#14653,.F.);
#19334=ORIENTED_EDGE('',*,*,#14655,.F.);
#19335=ORIENTED_EDGE('',*,*,#14657,.F.);
#19336=ORIENTED_EDGE('',*,*,#14659,.F.);
#19337=ORIENTED_EDGE('',*,*,#14661,.F.);
#19338=ORIENTED_EDGE('',*,*,#14663,.F.);
#19339=ORIENTED_EDGE('',*,*,#14665,.F.);
#19340=ORIENTED_EDGE('',*,*,#14667,.F.);
#19341=ORIENTED_EDGE('',*,*,#14669,.F.);
#19342=ORIENTED_EDGE('',*,*,#14671,.F.);
#19343=ORIENTED_EDGE('',*,*,#14673,.F.);
#19344=ORIENTED_EDGE('',*,*,#14675,.F.);
#19345=ORIENTED_EDGE('',*,*,#14677,.F.);
#19346=ORIENTED_EDGE('',*,*,#14679,.F.);
#19347=ORIENTED_EDGE('',*,*,#14681,.F.);
#19348=ORIENTED_EDGE('',*,*,#14683,.F.);
#19349=ORIENTED_EDGE('',*,*,#14685,.F.);
#19350=ORIENTED_EDGE('',*,*,#14687,.F.);
#19351=ORIENTED_EDGE('',*,*,#14689,.F.);
#19352=ORIENTED_EDGE('',*,*,#14691,.F.);
#19353=ORIENTED_EDGE('',*,*,#14693,.F.);
#19354=ORIENTED_EDGE('',*,*,#14695,.F.);
#19355=ORIENTED_EDGE('',*,*,#14697,.F.);
#19356=ORIENTED_EDGE('',*,*,#14699,.F.);
#19357=ORIENTED_EDGE('',*,*,#14701,.F.);
#19358=ORIENTED_EDGE('',*,*,#14703,.F.);
#19359=ORIENTED_EDGE('',*,*,#14705,.F.);
#19360=ORIENTED_EDGE('',*,*,#14707,.F.);
#19361=ORIENTED_EDGE('',*,*,#14709,.F.);
#19362=ORIENTED_EDGE('',*,*,#14711,.F.);
#19363=ORIENTED_EDGE('',*,*,#14713,.F.);
#19364=ORIENTED_EDGE('',*,*,#14715,.F.);
#19365=ORIENTED_EDGE('',*,*,#14717,.F.);
#19366=ORIENTED_EDGE('',*,*,#14518,.F.);
#19367=ORIENTED_EDGE('',*,*,#14719,.T.);
#19368=ORIENTED_EDGE('',*,*,#14720,.T.);
#19369=ORIENTED_EDGE('',*,*,#14721,.F.);
#19370=ORIENTED_EDGE('',*,*,#14517,.F.);
#19371=ORIENTED_EDGE('',*,*,#14722,.T.);
#19372=ORIENTED_EDGE('',*,*,#14723,.T.);
#19373=ORIENTED_EDGE('',*,*,#14719,.F.);
#19374=ORIENTED_EDGE('',*,*,#14516,.F.);
#19375=ORIENTED_EDGE('',*,*,#14724,.T.);
#19376=ORIENTED_EDGE('',*,*,#14725,.T.);
#19377=ORIENTED_EDGE('',*,*,#14722,.F.);
#19378=ORIENTED_EDGE('',*,*,#14515,.F.);
#19379=ORIENTED_EDGE('',*,*,#14726,.T.);
#19380=ORIENTED_EDGE('',*,*,#14727,.T.);
#19381=ORIENTED_EDGE('',*,*,#14724,.F.);
#19382=ORIENTED_EDGE('',*,*,#14514,.F.);
#19383=ORIENTED_EDGE('',*,*,#14728,.T.);
#19384=ORIENTED_EDGE('',*,*,#14729,.T.);
#19385=ORIENTED_EDGE('',*,*,#14726,.F.);
#19386=ORIENTED_EDGE('',*,*,#14513,.F.);
#19387=ORIENTED_EDGE('',*,*,#14601,.T.);
#19388=ORIENTED_EDGE('',*,*,#14730,.T.);
#19389=ORIENTED_EDGE('',*,*,#14728,.F.);
#19390=ORIENTED_EDGE('',*,*,#14584,.F.);
#19391=ORIENTED_EDGE('',*,*,#14504,.F.);
#19392=ORIENTED_EDGE('',*,*,#14731,.T.);
#19393=ORIENTED_EDGE('',*,*,#14732,.T.);
#19394=ORIENTED_EDGE('',*,*,#14599,.F.);
#19395=ORIENTED_EDGE('',*,*,#14503,.F.);
#19396=ORIENTED_EDGE('',*,*,#14733,.T.);
#19397=ORIENTED_EDGE('',*,*,#14734,.T.);
#19398=ORIENTED_EDGE('',*,*,#14731,.F.);
#19399=ORIENTED_EDGE('',*,*,#14502,.F.);
#19400=ORIENTED_EDGE('',*,*,#14735,.T.);
#19401=ORIENTED_EDGE('',*,*,#14736,.T.);
#19402=ORIENTED_EDGE('',*,*,#14733,.F.);
#19403=ORIENTED_EDGE('',*,*,#14501,.F.);
#19404=ORIENTED_EDGE('',*,*,#14737,.T.);
#19405=ORIENTED_EDGE('',*,*,#14738,.T.);
#19406=ORIENTED_EDGE('',*,*,#14735,.F.);
#19407=ORIENTED_EDGE('',*,*,#14500,.F.);
#19408=ORIENTED_EDGE('',*,*,#14739,.T.);
#19409=ORIENTED_EDGE('',*,*,#14740,.T.);
#19410=ORIENTED_EDGE('',*,*,#14737,.F.);
#19411=ORIENTED_EDGE('',*,*,#14499,.F.);
#19412=ORIENTED_EDGE('',*,*,#14741,.T.);
#19413=ORIENTED_EDGE('',*,*,#14742,.T.);
#19414=ORIENTED_EDGE('',*,*,#14739,.F.);
#19415=ORIENTED_EDGE('',*,*,#14498,.F.);
#19416=ORIENTED_EDGE('',*,*,#14743,.T.);
#19417=ORIENTED_EDGE('',*,*,#14744,.T.);
#19418=ORIENTED_EDGE('',*,*,#14741,.F.);
#19419=ORIENTED_EDGE('',*,*,#14497,.F.);
#19420=ORIENTED_EDGE('',*,*,#14745,.T.);
#19421=ORIENTED_EDGE('',*,*,#14746,.T.);
#19422=ORIENTED_EDGE('',*,*,#14743,.F.);
#19423=ORIENTED_EDGE('',*,*,#14496,.F.);
#19424=ORIENTED_EDGE('',*,*,#14574,.T.);
#19425=ORIENTED_EDGE('',*,*,#14747,.T.);
#19426=ORIENTED_EDGE('',*,*,#14745,.F.);
#19427=ORIENTED_EDGE('',*,*,#14520,.T.);
#19428=ORIENTED_EDGE('',*,*,#14748,.T.);
#19429=ORIENTED_EDGE('',*,*,#14749,.T.);
#19430=ORIENTED_EDGE('',*,*,#14575,.F.);
#19431=ORIENTED_EDGE('',*,*,#14519,.F.);
#19432=ORIENTED_EDGE('',*,*,#14721,.T.);
#19433=ORIENTED_EDGE('',*,*,#14750,.T.);
#19434=ORIENTED_EDGE('',*,*,#14748,.F.);
#19435=ORIENTED_EDGE('',*,*,#14750,.F.);
#19436=ORIENTED_EDGE('',*,*,#14720,.F.);
#19437=ORIENTED_EDGE('',*,*,#14723,.F.);
#19438=ORIENTED_EDGE('',*,*,#14725,.F.);
#19439=ORIENTED_EDGE('',*,*,#14727,.F.);
#19440=ORIENTED_EDGE('',*,*,#14729,.F.);
#19441=ORIENTED_EDGE('',*,*,#14730,.F.);
#19442=ORIENTED_EDGE('',*,*,#14600,.F.);
#19443=ORIENTED_EDGE('',*,*,#14732,.F.);
#19444=ORIENTED_EDGE('',*,*,#14734,.F.);
#19445=ORIENTED_EDGE('',*,*,#14736,.F.);
#19446=ORIENTED_EDGE('',*,*,#14738,.F.);
#19447=ORIENTED_EDGE('',*,*,#14740,.F.);
#19448=ORIENTED_EDGE('',*,*,#14742,.F.);
#19449=ORIENTED_EDGE('',*,*,#14744,.F.);
#19450=ORIENTED_EDGE('',*,*,#14746,.F.);
#19451=ORIENTED_EDGE('',*,*,#14747,.F.);
#19452=ORIENTED_EDGE('',*,*,#14576,.F.);
#19453=ORIENTED_EDGE('',*,*,#14749,.F.);
#19454=ORIENTED_EDGE('',*,*,#14459,.F.);
#19455=ORIENTED_EDGE('',*,*,#14751,.T.);
#19456=ORIENTED_EDGE('',*,*,#14752,.T.);
#19457=ORIENTED_EDGE('',*,*,#14753,.F.);
#19458=ORIENTED_EDGE('',*,*,#14469,.F.);
#19459=ORIENTED_EDGE('',*,*,#14754,.T.);
#19460=ORIENTED_EDGE('',*,*,#14755,.T.);
#19461=ORIENTED_EDGE('',*,*,#14751,.F.);
#19462=ORIENTED_EDGE('',*,*,#14468,.F.);
#19463=ORIENTED_EDGE('',*,*,#14756,.T.);
#19464=ORIENTED_EDGE('',*,*,#14757,.T.);
#19465=ORIENTED_EDGE('',*,*,#14754,.F.);
#19466=ORIENTED_EDGE('',*,*,#14467,.F.);
#19467=ORIENTED_EDGE('',*,*,#14758,.T.);
#19468=ORIENTED_EDGE('',*,*,#14759,.T.);
#19469=ORIENTED_EDGE('',*,*,#14756,.F.);
#19470=ORIENTED_EDGE('',*,*,#14466,.F.);
#19471=ORIENTED_EDGE('',*,*,#14760,.T.);
#19472=ORIENTED_EDGE('',*,*,#14761,.T.);
#19473=ORIENTED_EDGE('',*,*,#14758,.F.);
#19474=ORIENTED_EDGE('',*,*,#14465,.F.);
#19475=ORIENTED_EDGE('',*,*,#14762,.T.);
#19476=ORIENTED_EDGE('',*,*,#14763,.T.);
#19477=ORIENTED_EDGE('',*,*,#14760,.F.);
#19478=ORIENTED_EDGE('',*,*,#14464,.F.);
#19479=ORIENTED_EDGE('',*,*,#14764,.T.);
#19480=ORIENTED_EDGE('',*,*,#14765,.T.);
#19481=ORIENTED_EDGE('',*,*,#14762,.F.);
#19482=ORIENTED_EDGE('',*,*,#14463,.F.);
#19483=ORIENTED_EDGE('',*,*,#14766,.T.);
#19484=ORIENTED_EDGE('',*,*,#14767,.T.);
#19485=ORIENTED_EDGE('',*,*,#14764,.F.);
#19486=ORIENTED_EDGE('',*,*,#14462,.F.);
#19487=ORIENTED_EDGE('',*,*,#14768,.T.);
#19488=ORIENTED_EDGE('',*,*,#14769,.T.);
#19489=ORIENTED_EDGE('',*,*,#14766,.F.);
#19490=ORIENTED_EDGE('',*,*,#14461,.F.);
#19491=ORIENTED_EDGE('',*,*,#14770,.T.);
#19492=ORIENTED_EDGE('',*,*,#14771,.T.);
#19493=ORIENTED_EDGE('',*,*,#14768,.F.);
#19494=ORIENTED_EDGE('',*,*,#14460,.F.);
#19495=ORIENTED_EDGE('',*,*,#14753,.T.);
#19496=ORIENTED_EDGE('',*,*,#14772,.T.);
#19497=ORIENTED_EDGE('',*,*,#14770,.F.);
#19498=ORIENTED_EDGE('',*,*,#14772,.F.);
#19499=ORIENTED_EDGE('',*,*,#14752,.F.);
#19500=ORIENTED_EDGE('',*,*,#14755,.F.);
#19501=ORIENTED_EDGE('',*,*,#14757,.F.);
#19502=ORIENTED_EDGE('',*,*,#14759,.F.);
#19503=ORIENTED_EDGE('',*,*,#14761,.F.);
#19504=ORIENTED_EDGE('',*,*,#14763,.F.);
#19505=ORIENTED_EDGE('',*,*,#14765,.F.);
#19506=ORIENTED_EDGE('',*,*,#14767,.F.);
#19507=ORIENTED_EDGE('',*,*,#14769,.F.);
#19508=ORIENTED_EDGE('',*,*,#14771,.F.);
#19509=ORIENTED_EDGE('',*,*,#14370,.F.);
#19510=ORIENTED_EDGE('',*,*,#14773,.T.);
#19511=ORIENTED_EDGE('',*,*,#14417,.F.);
#19512=ORIENTED_EDGE('',*,*,#14560,.F.);
#19513=ORIENTED_EDGE('',*,*,#14418,.F.);
#19514=ORIENTED_EDGE('',*,*,#14773,.F.);
#19515=ORIENTED_EDGE('',*,*,#14371,.F.);
#19516=ORIENTED_EDGE('',*,*,#14774,.T.);
#19517=ORIENTED_EDGE('',*,*,#14410,.F.);
#19518=ORIENTED_EDGE('',*,*,#14565,.F.);
#19519=ORIENTED_EDGE('',*,*,#14411,.F.);
#19520=ORIENTED_EDGE('',*,*,#14774,.F.);
#19521=ORIENTED_EDGE('',*,*,#14372,.F.);
#19522=ORIENTED_EDGE('',*,*,#14775,.T.);
#19523=ORIENTED_EDGE('',*,*,#14414,.F.);
#19524=ORIENTED_EDGE('',*,*,#14561,.F.);
#19525=ORIENTED_EDGE('',*,*,#14415,.F.);
#19526=ORIENTED_EDGE('',*,*,#14775,.F.);
#19527=ORIENTED_EDGE('',*,*,#14373,.F.);
#19528=ORIENTED_EDGE('',*,*,#14776,.T.);
#19529=ORIENTED_EDGE('',*,*,#14407,.F.);
#19530=ORIENTED_EDGE('',*,*,#14566,.F.);
#19531=ORIENTED_EDGE('',*,*,#14408,.F.);
#19532=ORIENTED_EDGE('',*,*,#14776,.F.);
#19533=ORIENTED_EDGE('',*,*,#14572,.T.);
#19534=ORIENTED_EDGE('',*,*,#14551,.F.);
#19535=ORIENTED_EDGE('',*,*,#14539,.F.);
#19536=ORIENTED_EDGE('',*,*,#14777,.T.);
#19537=ORIENTED_EDGE('',*,*,#14778,.T.);
#19538=ORIENTED_EDGE('',*,*,#14779,.F.);
#19539=ORIENTED_EDGE('',*,*,#14543,.F.);
#19540=ORIENTED_EDGE('',*,*,#14556,.T.);
#19541=ORIENTED_EDGE('',*,*,#14780,.T.);
#19542=ORIENTED_EDGE('',*,*,#14777,.F.);
#19543=ORIENTED_EDGE('',*,*,#14544,.F.);
#19544=ORIENTED_EDGE('',*,*,#14779,.T.);
#19545=ORIENTED_EDGE('',*,*,#14781,.T.);
#19546=ORIENTED_EDGE('',*,*,#14552,.F.);
#19547=ORIENTED_EDGE('',*,*,#14781,.F.);
#19548=ORIENTED_EDGE('',*,*,#14778,.F.);
#19549=ORIENTED_EDGE('',*,*,#14780,.F.);
#19550=ORIENTED_EDGE('',*,*,#14555,.F.);
#19551=ORIENTED_EDGE('',*,*,#14553,.F.);
#19552=ORIENTED_EDGE('',*,*,#14290,.F.);
#19553=ORIENTED_EDGE('',*,*,#14523,.F.);
#19554=ORIENTED_EDGE('',*,*,#14535,.F.);
#19555=ORIENTED_EDGE('',*,*,#14380,.F.);
#25611=TOROIDAL_SURFACE('',#27817,90.5,1.5);
#25612=TOROIDAL_SURFACE('',#27825,90.3786796564403,1.5);
#25613=TOROIDAL_SURFACE('',#27846,90.5,1.5);
#25614=TOROIDAL_SURFACE('',#27875,54.8786796564404,1.5);
#25615=TOROIDAL_SURFACE('',#27889,55.,1.5);
#25616=TOROIDAL_SURFACE('',#27895,55.5,1.5);
#25617=TOROIDAL_SURFACE('',#27902,71.7,1.5);
#25618=TOROIDAL_SURFACE('',#27910,76.55,1.5);
#25808=ADVANCED_FACE('',(#6984),#496,.T.);
#25809=ADVANCED_FACE('',(#6985),#497,.T.);
#25810=ADVANCED_FACE('',(#6986),#810,.T.);
#25811=ADVANCED_FACE('',(#6987),#811,.T.);
#25812=ADVANCED_FACE('',(#6988),#6569,.T.);
#25813=ADVANCED_FACE('',(#6989),#812,.T.);
#25814=ADVANCED_FACE('',(#6990),#498,.T.);
#25815=ADVANCED_FACE('',(#6991),#499,.T.);
#25816=ADVANCED_FACE('',(#6992),#813,.T.);
#25817=ADVANCED_FACE('',(#6993),#6570,.T.);
#25818=ADVANCED_FACE('',(#6994),#814,.T.);
#25819=ADVANCED_FACE('',(#6995),#500,.T.);
#25820=ADVANCED_FACE('',(#6996),#501,.T.);
#25821=ADVANCED_FACE('',(#6997),#815,.T.);
#25822=ADVANCED_FACE('',(#6998),#816,.T.);
#25823=ADVANCED_FACE('',(#6999),#6571,.T.);
#25824=ADVANCED_FACE('',(#7000),#817,.T.);
#25825=ADVANCED_FACE('',(#7001),#502,.T.);
#25826=ADVANCED_FACE('',(#7002),#503,.T.);
#25827=ADVANCED_FACE('',(#7003),#818,.T.);
#25828=ADVANCED_FACE('',(#7004),#819,.T.);
#25829=ADVANCED_FACE('',(#7005),#6572,.T.);
#25830=ADVANCED_FACE('',(#7006),#820,.T.);
#25831=ADVANCED_FACE('',(#7007),#504,.T.);
#25832=ADVANCED_FACE('',(#7008),#505,.T.);
#25833=ADVANCED_FACE('',(#7009),#821,.T.);
#25834=ADVANCED_FACE('',(#7010),#6573,.T.);
#25835=ADVANCED_FACE('',(#7011),#822,.T.);
#25836=ADVANCED_FACE('',(#7012),#506,.T.);
#25837=ADVANCED_FACE('',(#7013),#507,.T.);
#25838=ADVANCED_FACE('',(#7014),#823,.T.);
#25839=ADVANCED_FACE('',(#7015),#824,.T.);
#25840=ADVANCED_FACE('',(#7016),#6574,.T.);
#25841=ADVANCED_FACE('',(#7017),#825,.T.);
#25842=ADVANCED_FACE('',(#7018),#508,.T.);
#25843=ADVANCED_FACE('',(#7019),#509,.T.);
#25844=ADVANCED_FACE('',(#7020),#826,.T.);
#25845=ADVANCED_FACE('',(#7021),#6575,.T.);
#25846=ADVANCED_FACE('',(#7022),#827,.T.);
#25847=ADVANCED_FACE('',(#7023),#25611,.T.);
#25848=ADVANCED_FACE('',(#7024),#339,.T.);
#25849=ADVANCED_FACE('',(#7025),#6576,.T.);
#25850=ADVANCED_FACE('',(#7026),#25612,.T.);
#25851=ADVANCED_FACE('',(#7027,#631,#632,#633,#634,#635,#636,#637,#638,
#639),#828,.T.);
#25852=ADVANCED_FACE('',(#7028),#6577,.T.);
#25853=ADVANCED_FACE('',(#7029),#829,.T.);
#25854=ADVANCED_FACE('',(#7030),#6578,.T.);
#25855=ADVANCED_FACE('',(#7031),#830,.T.);
#25856=ADVANCED_FACE('',(#7032),#25613,.T.);
#25857=ADVANCED_FACE('',(#7033,#640),#831,.T.);
#25858=ADVANCED_FACE('',(#7034),#25614,.T.);
#25859=ADVANCED_FACE('',(#7035),#340,.T.);
#25860=ADVANCED_FACE('',(#7036,#641,#642,#643,#644,#645),#832,.T.);
#25861=ADVANCED_FACE('',(#7037),#6579,.T.);
#25862=ADVANCED_FACE('',(#7038),#6580,.T.);
#25863=ADVANCED_FACE('',(#7039),#338,.T.);
#25864=ADVANCED_FACE('',(#7040),#6581,.T.);
#25865=ADVANCED_FACE('',(#7041),#833,.T.);
#25866=ADVANCED_FACE('',(#7042),#25615,.T.);
#25867=ADVANCED_FACE('',(#7043),#6582,.T.);
#25868=ADVANCED_FACE('',(#7044),#6583,.T.);
#25869=ADVANCED_FACE('',(#7045),#834,.T.);
#25870=ADVANCED_FACE('',(#7046),#25616,.T.);
#25871=ADVANCED_FACE('',(#7047),#6584,.T.);
#25872=ADVANCED_FACE('',(#7048),#6585,.T.);
#25873=ADVANCED_FACE('',(#7049),#835,.F.);
#25874=ADVANCED_FACE('',(#7050),#25617,.T.);
#25875=ADVANCED_FACE('',(#7051),#6586,.F.);
#25876=ADVANCED_FACE('',(#7052),#25618,.T.);
#25877=ADVANCED_FACE('',(#7053),#6587,.F.);
#25878=ADVANCED_FACE('',(#7054),#6588,.F.);
#25879=ADVANCED_FACE('',(#7055),#6589,.F.);
#25880=ADVANCED_FACE('',(#7056),#6590,.F.);
#25881=ADVANCED_FACE('',(#7057),#6591,.F.);
#25882=ADVANCED_FACE('',(#7058),#6592,.T.);
#25883=ADVANCED_FACE('',(#7059),#6593,.T.);
#25884=ADVANCED_FACE('',(#7060),#6594,.T.);
#25885=ADVANCED_FACE('',(#7061),#6595,.T.);
#25886=ADVANCED_FACE('',(#7062),#6596,.T.);
#25887=ADVANCED_FACE('',(#7063),#836,.F.);
#25888=ADVANCED_FACE('',(#7064),#837,.F.);
#25889=ADVANCED_FACE('',(#7065),#838,.F.);
#25890=ADVANCED_FACE('',(#7066),#839,.F.);
#25891=ADVANCED_FACE('',(#7067),#840,.F.);
#25892=ADVANCED_FACE('',(#7068),#841,.F.);
#25893=ADVANCED_FACE('',(#7069),#842,.F.);
#25894=ADVANCED_FACE('',(#7070),#843,.F.);
#25895=ADVANCED_FACE('',(#7071),#844,.F.);
#25896=ADVANCED_FACE('',(#7072),#845,.F.);
#25897=ADVANCED_FACE('',(#7073),#846,.F.);
#25898=ADVANCED_FACE('',(#7074),#847,.F.);
#25899=ADVANCED_FACE('',(#7075),#848,.F.);
#25900=ADVANCED_FACE('',(#7076),#849,.F.);
#25901=ADVANCED_FACE('',(#7077),#850,.F.);
#25902=ADVANCED_FACE('',(#7078),#851,.F.);
#25903=ADVANCED_FACE('',(#7079),#852,.F.);
#25904=ADVANCED_FACE('',(#7080),#853,.F.);
#25905=ADVANCED_FACE('',(#7081),#854,.F.);
#25906=ADVANCED_FACE('',(#7082),#510,.F.);
#25907=ADVANCED_FACE('',(#7083),#511,.F.);
#25908=ADVANCED_FACE('',(#7084),#512,.F.);
#25909=ADVANCED_FACE('',(#7085),#513,.F.);
#25910=ADVANCED_FACE('',(#7086),#514,.F.);
#25911=ADVANCED_FACE('',(#7087),#515,.F.);
#25912=ADVANCED_FACE('',(#7088),#516,.F.);
#25913=ADVANCED_FACE('',(#7089),#517,.F.);
#25914=ADVANCED_FACE('',(#7090),#518,.F.);
#25915=ADVANCED_FACE('',(#7091),#519,.F.);
#25916=ADVANCED_FACE('',(#7092),#855,.F.);
#25917=ADVANCED_FACE('',(#7093),#856,.F.);
#25918=ADVANCED_FACE('',(#7094),#520,.F.);
#25919=ADVANCED_FACE('',(#7095),#857,.T.);
#25920=ADVANCED_FACE('',(#7096),#521,.F.);
#25921=ADVANCED_FACE('',(#7097),#522,.F.);
#25922=ADVANCED_FACE('',(#7098),#523,.F.);
#25923=ADVANCED_FACE('',(#7099),#524,.F.);
#25924=ADVANCED_FACE('',(#7100),#525,.F.);
#25925=ADVANCED_FACE('',(#7101),#526,.F.);
#25926=ADVANCED_FACE('',(#7102),#527,.F.);
#25927=ADVANCED_FACE('',(#7103),#528,.F.);
#25928=ADVANCED_FACE('',(#7104),#529,.F.);
#25929=ADVANCED_FACE('',(#7105),#530,.F.);
#25930=ADVANCED_FACE('',(#7106),#531,.F.);
#25931=ADVANCED_FACE('',(#7107),#532,.F.);
#25932=ADVANCED_FACE('',(#7108),#533,.F.);
#25933=ADVANCED_FACE('',(#7109),#858,.F.);
#25934=ADVANCED_FACE('',(#7110),#534,.F.);
#25935=ADVANCED_FACE('',(#7111),#535,.F.);
#25936=ADVANCED_FACE('',(#7112),#536,.F.);
#25937=ADVANCED_FACE('',(#7113),#537,.F.);
#25938=ADVANCED_FACE('',(#7114),#538,.F.);
#25939=ADVANCED_FACE('',(#7115),#539,.F.);
#25940=ADVANCED_FACE('',(#7116),#540,.F.);
#25941=ADVANCED_FACE('',(#7117),#541,.F.);
#25942=ADVANCED_FACE('',(#7118),#542,.F.);
#25943=ADVANCED_FACE('',(#7119),#543,.F.);
#25944=ADVANCED_FACE('',(#7120),#544,.F.);
#25945=ADVANCED_FACE('',(#7121),#545,.F.);
#25946=ADVANCED_FACE('',(#7122),#546,.F.);
#25947=ADVANCED_FACE('',(#7123),#547,.F.);
#25948=ADVANCED_FACE('',(#7124),#548,.F.);
#25949=ADVANCED_FACE('',(#7125),#549,.F.);
#25950=ADVANCED_FACE('',(#7126),#550,.F.);
#25951=ADVANCED_FACE('',(#7127),#551,.F.);
#25952=ADVANCED_FACE('',(#7128),#859,.F.);
#25953=ADVANCED_FACE('',(#7129),#552,.F.);
#25954=ADVANCED_FACE('',(#7130),#553,.F.);
#25955=ADVANCED_FACE('',(#7131),#860,.T.);
#25956=ADVANCED_FACE('',(#7132),#861,.F.);
#25957=ADVANCED_FACE('',(#7133),#554,.F.);
#25958=ADVANCED_FACE('',(#7134),#555,.F.);
#25959=ADVANCED_FACE('',(#7135),#556,.F.);
#25960=ADVANCED_FACE('',(#7136),#557,.F.);
#25961=ADVANCED_FACE('',(#7137),#862,.F.);
#25962=ADVANCED_FACE('',(#7138),#863,.F.);
#25963=ADVANCED_FACE('',(#7139),#558,.F.);
#25964=ADVANCED_FACE('',(#7140),#559,.F.);
#25965=ADVANCED_FACE('',(#7141),#560,.F.);
#25966=ADVANCED_FACE('',(#7142),#561,.F.);
#25967=ADVANCED_FACE('',(#7143),#562,.F.);
#25968=ADVANCED_FACE('',(#7144),#563,.F.);
#25969=ADVANCED_FACE('',(#7145),#564,.F.);
#25970=ADVANCED_FACE('',(#7146),#864,.F.);
#25971=ADVANCED_FACE('',(#7147),#865,.F.);
#25972=ADVANCED_FACE('',(#7148),#866,.F.);
#25973=ADVANCED_FACE('',(#7149),#867,.T.);
#25974=ADVANCED_FACE('',(#7150),#868,.F.);
#25975=ADVANCED_FACE('',(#7151),#869,.F.);
#25976=ADVANCED_FACE('',(#7152),#870,.F.);
#25977=ADVANCED_FACE('',(#7153),#565,.F.);
#25978=ADVANCED_FACE('',(#7154),#566,.F.);
#25979=ADVANCED_FACE('',(#7155),#871,.F.);
#25980=ADVANCED_FACE('',(#7156),#872,.F.);
#25981=ADVANCED_FACE('',(#7157),#873,.F.);
#25982=ADVANCED_FACE('',(#7158),#874,.F.);
#25983=ADVANCED_FACE('',(#7159),#875,.F.);
#25984=ADVANCED_FACE('',(#7160),#876,.F.);
#25985=ADVANCED_FACE('',(#7161),#877,.T.);
#25986=ADVANCED_FACE('',(#7162),#6597,.F.);
#25987=ADVANCED_FACE('',(#7163),#6598,.F.);
#25988=ADVANCED_FACE('',(#7164),#6599,.F.);
#25989=ADVANCED_FACE('',(#7165),#6600,.F.);
#25990=ADVANCED_FACE('',(#7166,#646),#878,.F.);
#25991=ADVANCED_FACE('',(#7167),#6601,.T.);
#25992=ADVANCED_FACE('',(#7168),#879,.F.);
#25993=ADVANCED_FACE('',(#7169),#880,.F.);
#25994=ADVANCED_FACE('',(#7170),#881,.T.);
#25995=ADVANCED_FACE('',(#7171),#882,.T.);
#27222=CLOSED_SHELL('',(#25808,#25809,#25810,#25811,#25812,#25813,#25814,
#25815,#25816,#25817,#25818,#25819,#25820,#25821,#25822,#25823,#25824,#25825,
#25826,#25827,#25828,#25829,#25830,#25831,#25832,#25833,#25834,#25835,#25836,
#25837,#25838,#25839,#25840,#25841,#25842,#25843,#25844,#25845,#25846,#25847,
#25848,#25849,#25850,#25851,#25852,#25853,#25854,#25855,#25856,#25857,#25858,
#25859,#25860,#25861,#25862,#25863,#25864,#25865,#25866,#25867,#25868,#25869,
#25870,#25871,#25872,#25873,#25874,#25875,#25876,#25877,#25878,#25879,#25880,
#25881,#25882,#25883,#25884,#25885,#25886,#25887,#25888,#25889,#25890,#25891,
#25892,#25893,#25894,#25895,#25896,#25897,#25898,#25899,#25900,#25901,#25902,
#25903,#25904,#25905,#25906,#25907,#25908,#25909,#25910,#25911,#25912,#25913,
#25914,#25915,#25916,#25917,#25918,#25919,#25920,#25921,#25922,#25923,#25924,
#25925,#25926,#25927,#25928,#25929,#25930,#25931,#25932,#25933,#25934,#25935,
#25936,#25937,#25938,#25939,#25940,#25941,#25942,#25943,#25944,#25945,#25946,
#25947,#25948,#25949,#25950,#25951,#25952,#25953,#25954,#25955,#25956,#25957,
#25958,#25959,#25960,#25961,#25962,#25963,#25964,#25965,#25966,#25967,#25968,
#25969,#25970,#25971,#25972,#25973,#25974,#25975,#25976,#25977,#25978,#25979,
#25980,#25981,#25982,#25983,#25984,#25985,#25986,#25987,#25988,#25989,#25990,
#25991,#25992,#25993,#25994,#25995));
#27785=AXIS2_PLACEMENT_3D('',#38585,#30763,#30764);
#27786=AXIS2_PLACEMENT_3D('',#38768,#30767,#30768);
#27787=AXIS2_PLACEMENT_3D('',#38774,#30772,#30773);
#27788=AXIS2_PLACEMENT_3D('',#38782,#30777,#30778);
#27789=AXIS2_PLACEMENT_3D('',#38784,#30779,#30780);
#27790=AXIS2_PLACEMENT_3D('',#38786,#30782,#30783);
#27791=AXIS2_PLACEMENT_3D('',#38852,#30785,#30786);
#27792=AXIS2_PLACEMENT_3D('',#38977,#30790,#30791);
#27793=AXIS2_PLACEMENT_3D('',#38981,#30794,#30795);
#27794=AXIS2_PLACEMENT_3D('',#38994,#30797,#30798);
#27795=AXIS2_PLACEMENT_3D('',#39180,#30803,#30804);
#27796=AXIS2_PLACEMENT_3D('',#39186,#30808,#30809);
#27797=AXIS2_PLACEMENT_3D('',#39192,#30812,#30813);
#27798=AXIS2_PLACEMENT_3D('',#39194,#30815,#30816);
#27799=AXIS2_PLACEMENT_3D('',#39197,#30818,#30819);
#27800=AXIS2_PLACEMENT_3D('',#39198,#30820,#30821);
#27801=AXIS2_PLACEMENT_3D('',#39384,#30826,#30827);
#27802=AXIS2_PLACEMENT_3D('',#39390,#30831,#30832);
#27803=AXIS2_PLACEMENT_3D('',#39398,#30836,#30837);
#27804=AXIS2_PLACEMENT_3D('',#39400,#30839,#30840);
#27805=AXIS2_PLACEMENT_3D('',#39465,#30842,#30843);
#27806=AXIS2_PLACEMENT_3D('',#39585,#30847,#30848);
#27807=AXIS2_PLACEMENT_3D('',#39589,#30851,#30852);
#27808=AXIS2_PLACEMENT_3D('',#39602,#30854,#30855);
#27809=AXIS2_PLACEMENT_3D('',#39794,#30860,#30861);
#27810=AXIS2_PLACEMENT_3D('',#39800,#30865,#30866);
#27811=AXIS2_PLACEMENT_3D('',#39808,#30870,#30871);
#27812=AXIS2_PLACEMENT_3D('',#39810,#30873,#30874);
#27813=AXIS2_PLACEMENT_3D('',#39876,#30876,#30877);
#27814=AXIS2_PLACEMENT_3D('',#40001,#30881,#30882);
#27815=AXIS2_PLACEMENT_3D('',#40005,#30885,#30886);
#27816=AXIS2_PLACEMENT_3D('',#40018,#30888,#30889);
#27817=AXIS2_PLACEMENT_3D('',#40022,#30892,#30893);
#27818=AXIS2_PLACEMENT_3D('',#40024,#30894,#30895);
#27819=AXIS2_PLACEMENT_3D('',#40026,#30896,#30897);
#27820=AXIS2_PLACEMENT_3D('',#40027,#30898,#30899);
#27821=AXIS2_PLACEMENT_3D('',#40028,#30900,#30901);
#27822=AXIS2_PLACEMENT_3D('',#40031,#30903,#30904);
#27823=AXIS2_PLACEMENT_3D('',#40032,#30905,#30906);
#27824=AXIS2_PLACEMENT_3D('',#40034,#30907,#30908);
#27825=AXIS2_PLACEMENT_3D('',#40036,#30910,#30911);
#27826=AXIS2_PLACEMENT_3D('',#40038,#30912,#30913);
#27827=AXIS2_PLACEMENT_3D('',#40039,#30914,#30915);
#27828=AXIS2_PLACEMENT_3D('',#40040,#30916,#30917);
#27829=AXIS2_PLACEMENT_3D('',#40042,#30918,#30919);
#27830=AXIS2_PLACEMENT_3D('',#40044,#30920,#30921);
#27831=AXIS2_PLACEMENT_3D('',#40046,#30922,#30923);
#27832=AXIS2_PLACEMENT_3D('',#40048,#30924,#30925);
#27833=AXIS2_PLACEMENT_3D('',#40050,#30926,#30927);
#27834=AXIS2_PLACEMENT_3D('',#40052,#30928,#30929);
#27835=AXIS2_PLACEMENT_3D('',#40054,#30930,#30931);
#27836=AXIS2_PLACEMENT_3D('',#40056,#30932,#30933);
#27837=AXIS2_PLACEMENT_3D('',#40060,#30935,#30936);
#27838=AXIS2_PLACEMENT_3D('',#40063,#30938,#30939);
#27839=AXIS2_PLACEMENT_3D('',#40066,#30941,#30942);
#27840=AXIS2_PLACEMENT_3D('',#40069,#30944,#30945);
#27841=AXIS2_PLACEMENT_3D('',#40072,#30947,#30948);
#27842=AXIS2_PLACEMENT_3D('',#40073,#30949,#30950);
#27843=AXIS2_PLACEMENT_3D('',#40086,#30952,#30953);
#27844=AXIS2_PLACEMENT_3D('',#40088,#30955,#30956);
#27845=AXIS2_PLACEMENT_3D('',#40101,#30958,#30959);
#27846=AXIS2_PLACEMENT_3D('',#40103,#30961,#30962);
#27847=AXIS2_PLACEMENT_3D('',#40105,#30963,#30964);
#27848=AXIS2_PLACEMENT_3D('',#40106,#30965,#30966);
#27849=AXIS2_PLACEMENT_3D('',#40107,#30967,#30968);
#27850=AXIS2_PLACEMENT_3D('',#40110,#30969,#30970);
#27851=AXIS2_PLACEMENT_3D('',#40112,#30971,#30972);
#27852=AXIS2_PLACEMENT_3D('',#40114,#30973,#30974);
#27853=AXIS2_PLACEMENT_3D('',#40116,#30975,#30976);
#27854=AXIS2_PLACEMENT_3D('',#40118,#30977,#30978);
#27855=AXIS2_PLACEMENT_3D('',#40120,#30979,#30980);
#27856=AXIS2_PLACEMENT_3D('',#40122,#30981,#30982);
#27857=AXIS2_PLACEMENT_3D('',#40124,#30983,#30984);
#27858=AXIS2_PLACEMENT_3D('',#40126,#30985,#30986);
#27859=AXIS2_PLACEMENT_3D('',#40128,#30987,#30988);
#27860=AXIS2_PLACEMENT_3D('',#40130,#30989,#30990);
#27861=AXIS2_PLACEMENT_3D('',#40132,#30991,#30992);
#27862=AXIS2_PLACEMENT_3D('',#40134,#30993,#30994);
#27863=AXIS2_PLACEMENT_3D('',#40136,#30995,#30996);
#27864=AXIS2_PLACEMENT_3D('',#40138,#30997,#30998);
#27865=AXIS2_PLACEMENT_3D('',#40140,#30999,#31000);
#27866=AXIS2_PLACEMENT_3D('',#40142,#31001,#31002);
#27867=AXIS2_PLACEMENT_3D('',#40144,#31003,#31004);
#27868=AXIS2_PLACEMENT_3D('',#40146,#31005,#31006);
#27869=AXIS2_PLACEMENT_3D('',#40148,#31007,#31008);
#27870=AXIS2_PLACEMENT_3D('',#40150,#31009,#31010);
#27871=AXIS2_PLACEMENT_3D('',#40152,#31011,#31012);
#27872=AXIS2_PLACEMENT_3D('',#40154,#31013,#31014);
#27873=AXIS2_PLACEMENT_3D('',#40156,#31015,#31016);
#27874=AXIS2_PLACEMENT_3D('',#40157,#31017,#31018);
#27875=AXIS2_PLACEMENT_3D('',#40158,#31019,#31020);
#27876=AXIS2_PLACEMENT_3D('',#40160,#31021,#31022);
#27877=AXIS2_PLACEMENT_3D('',#40162,#31023,#31024);
#27878=AXIS2_PLACEMENT_3D('',#40163,#31025,#31026);
#27879=AXIS2_PLACEMENT_3D('',#40164,#31027,#31028);
#27880=AXIS2_PLACEMENT_3D('',#40166,#31029,#31030);
#27881=AXIS2_PLACEMENT_3D('',#40168,#31032,#31033);
#27882=AXIS2_PLACEMENT_3D('',#40479,#31075,#31076);
#27883=AXIS2_PLACEMENT_3D('',#40492,#31078,#31079);
#27884=AXIS2_PLACEMENT_3D('',#40494,#31080,#31081);
#27885=AXIS2_PLACEMENT_3D('',#40496,#31083,#31084);
#27886=AXIS2_PLACEMENT_3D('',#40497,#31085,#31086);
#27887=AXIS2_PLACEMENT_3D('',#40498,#31087,#31088);
#27888=AXIS2_PLACEMENT_3D('',#40511,#31090,#31091);
#27889=AXIS2_PLACEMENT_3D('',#40513,#31093,#31094);
#27890=AXIS2_PLACEMENT_3D('',#40515,#31095,#31096);
#27891=AXIS2_PLACEMENT_3D('',#40516,#31097,#31098);
#27892=AXIS2_PLACEMENT_3D('',#40517,#31099,#31100);
#27893=AXIS2_PLACEMENT_3D('',#40532,#31104,#31105);
#27894=AXIS2_PLACEMENT_3D('',#40534,#31107,#31108);
#27895=AXIS2_PLACEMENT_3D('',#40535,#31109,#31110);
#27896=AXIS2_PLACEMENT_3D('',#40538,#31111,#31112);
#27897=AXIS2_PLACEMENT_3D('',#40555,#31113,#31114);
#27898=AXIS2_PLACEMENT_3D('',#40570,#31115,#31116);
#27899=AXIS2_PLACEMENT_3D('',#40585,#31119,#31120);
#27900=AXIS2_PLACEMENT_3D('',#40600,#31123,#31124);
#27901=AXIS2_PLACEMENT_3D('',#40601,#31125,#31126);
#27902=AXIS2_PLACEMENT_3D('',#40602,#31127,#31128);
#27903=AXIS2_PLACEMENT_3D('',#40605,#31129,#31130);
#27904=AXIS2_PLACEMENT_3D('',#40606,#31131,#31132);
#27905=AXIS2_PLACEMENT_3D('',#40608,#31133,#31134);
#27906=AXIS2_PLACEMENT_3D('',#40609,#31135,#31136);
#27907=AXIS2_PLACEMENT_3D('',#40610,#31137,#31138);
#27908=AXIS2_PLACEMENT_3D('',#40614,#31140,#31141);
#27909=AXIS2_PLACEMENT_3D('',#40617,#31143,#31144);
#27910=AXIS2_PLACEMENT_3D('',#40619,#31146,#31147);
#27911=AXIS2_PLACEMENT_3D('',#40641,#31148,#31149);
#27912=AXIS2_PLACEMENT_3D('',#40643,#31150,#31151);
#27913=AXIS2_PLACEMENT_3D('',#40644,#31152,#31153);
#27914=AXIS2_PLACEMENT_3D('',#40657,#31154,#31155);
#27915=AXIS2_PLACEMENT_3D('',#40659,#31157,#31158);
#27916=AXIS2_PLACEMENT_3D('',#40661,#31160,#31161);
#27917=AXIS2_PLACEMENT_3D('',#40663,#31163,#31164);
#27918=AXIS2_PLACEMENT_3D('',#40665,#31166,#31167);
#27919=AXIS2_PLACEMENT_3D('',#40667,#31168,#31169);
#27920=AXIS2_PLACEMENT_3D('',#40669,#31171,#31172);
#27921=AXIS2_PLACEMENT_3D('',#40671,#31173,#31174);
#27922=AXIS2_PLACEMENT_3D('',#40673,#31175,#31176);
#27923=AXIS2_PLACEMENT_3D('',#40675,#31178,#31179);
#27924=AXIS2_PLACEMENT_3D('',#40677,#31180,#31181);
#27925=AXIS2_PLACEMENT_3D('',#40679,#31182,#31183);
#27926=AXIS2_PLACEMENT_3D('',#40681,#31185,#31186);
#27927=AXIS2_PLACEMENT_3D('',#40683,#31187,#31188);
#27928=AXIS2_PLACEMENT_3D('',#40685,#31189,#31190);
#27929=AXIS2_PLACEMENT_3D('',#40687,#31192,#31193);
#27930=AXIS2_PLACEMENT_3D('',#40689,#31194,#31195);
#27931=AXIS2_PLACEMENT_3D('',#40691,#31196,#31197);
#27932=AXIS2_PLACEMENT_3D('',#40693,#31198,#31199);
#27933=AXIS2_PLACEMENT_3D('',#40695,#31201,#31202);
#27934=AXIS2_PLACEMENT_3D('',#40697,#31203,#31204);
#27935=AXIS2_PLACEMENT_3D('',#40699,#31205,#31206);
#27936=AXIS2_PLACEMENT_3D('',#40701,#31208,#31209);
#27937=AXIS2_PLACEMENT_3D('',#40707,#31213,#31214);
#27938=AXIS2_PLACEMENT_3D('',#40711,#31217,#31218);
#27939=AXIS2_PLACEMENT_3D('',#40713,#31220,#31221);
#27940=AXIS2_PLACEMENT_3D('',#40715,#31223,#31224);
#27941=AXIS2_PLACEMENT_3D('',#40724,#31230,#31231);
#27942=AXIS2_PLACEMENT_3D('',#40726,#31233,#31234);
#27943=AXIS2_PLACEMENT_3D('',#40727,#31235,#31236);
#27944=AXIS2_PLACEMENT_3D('',#40733,#31240,#31241);
#27945=AXIS2_PLACEMENT_3D('',#40737,#31244,#31245);
#27946=AXIS2_PLACEMENT_3D('',#40741,#31248,#31249);
#27947=AXIS2_PLACEMENT_3D('',#40745,#31252,#31253);
#27948=AXIS2_PLACEMENT_3D('',#40749,#31256,#31257);
#27949=AXIS2_PLACEMENT_3D('',#40753,#31260,#31261);
#27950=AXIS2_PLACEMENT_3D('',#40757,#31264,#31265);
#27951=AXIS2_PLACEMENT_3D('',#40761,#31268,#31269);
#27952=AXIS2_PLACEMENT_3D('',#40763,#31271,#31272);
#27953=AXIS2_PLACEMENT_3D('',#40767,#31275,#31276);
#27954=AXIS2_PLACEMENT_3D('',#40769,#31278,#31279);
#27955=AXIS2_PLACEMENT_3D('',#40882,#31291,#31292);
#27956=AXIS2_PLACEMENT_3D('',#40884,#31294,#31295);
#27957=AXIS2_PLACEMENT_3D('',#40897,#31298,#31299);
#27958=AXIS2_PLACEMENT_3D('',#41043,#31314,#31315);
#27959=AXIS2_PLACEMENT_3D('',#41245,#31336,#31337);
#27960=AXIS2_PLACEMENT_3D('',#41269,#31341,#31342);
#27961=AXIS2_PLACEMENT_3D('',#41270,#31343,#31344);
#27962=AXIS2_PLACEMENT_3D('',#41320,#31352,#31353);
#27963=AXIS2_PLACEMENT_3D('',#41322,#31355,#31356);
#27964=AXIS2_PLACEMENT_3D('',#41403,#31366,#31367);
#27965=AXIS2_PLACEMENT_3D('',#41405,#31369,#31370);
#27966=AXIS2_PLACEMENT_3D('',#41409,#31373,#31374);
#27967=AXIS2_PLACEMENT_3D('',#41411,#31376,#31377);
#27968=AXIS2_PLACEMENT_3D('',#41412,#31378,#31379);
#27969=AXIS2_PLACEMENT_3D('',#41418,#31383,#31384);
#27970=AXIS2_PLACEMENT_3D('',#41422,#31387,#31388);
#27971=AXIS2_PLACEMENT_3D('',#41448,#31393,#31394);
#27972=AXIS2_PLACEMENT_3D('',#41452,#31397,#31398);
#27973=AXIS2_PLACEMENT_3D('',#41456,#31401,#31402);
#27974=AXIS2_PLACEMENT_3D('',#41460,#31405,#31406);
#27975=AXIS2_PLACEMENT_3D('',#41464,#31409,#31410);
#27976=AXIS2_PLACEMENT_3D('',#41468,#31413,#31414);
#27977=AXIS2_PLACEMENT_3D('',#41470,#31416,#31417);
#27978=AXIS2_PLACEMENT_3D('',#41471,#31418,#31419);
#27979=AXIS2_PLACEMENT_3D('',#41473,#31421,#31422);
#27980=AXIS2_PLACEMENT_3D('',#41475,#31424,#31425);
#27981=AXIS2_PLACEMENT_3D('',#41477,#31427,#31428);
#27982=AXIS2_PLACEMENT_3D('',#41479,#31430,#31431);
#27983=AXIS2_PLACEMENT_3D('',#41480,#31432,#31433);
#27984=AXIS2_PLACEMENT_3D('',#41484,#31435,#31436);
#27985=AXIS2_PLACEMENT_3D('',#41486,#31438,#31439);
#27986=AXIS2_PLACEMENT_3D('',#41488,#31441,#31442);
#27987=AXIS2_PLACEMENT_3D('',#41490,#31444,#31445);
#27988=AXIS2_PLACEMENT_3D('',#41491,#31446,#31447);
#30763=DIRECTION('axis',(0.,0.,1.));
#30764=DIRECTION('refdir',(1.,0.,0.));
#30765=DIRECTION('',(-0.707106781186548,0.,0.707106781186547));
#30766=DIRECTION('',(0.70710678118655,-3.14018491736755E-15,-0.707106781186545));
#30767=DIRECTION('center_axis',(-0.707106781186546,0.,-0.707106781186549));
#30768=DIRECTION('ref_axis',(-0.707106781186549,0.,0.707106781186546));
#30769=DIRECTION('',(-0.707106781186549,0.,0.707106781186546));
#30770=DIRECTION('',(0.,-1.,0.));
#30771=DIRECTION('',(0.,1.,0.));
#30772=DIRECTION('center_axis',(0.,-1.,0.));
#30773=DIRECTION('ref_axis',(0.,0.,-1.));
#30774=DIRECTION('',(-1.,0.,0.));
#30775=DIRECTION('',(-0.707106781186548,0.,-0.707106781186547));
#30776=DIRECTION('',(-1.85037170770859E-16,0.,-1.));
#30777=DIRECTION('center_axis',(0.,-1.,0.));
#30778=DIRECTION('ref_axis',(0.,0.,1.));
#30779=DIRECTION('center_axis',(0.,-1.,0.));
#30780=DIRECTION('ref_axis',(0.,0.,1.));
#30781=DIRECTION('',(1.85037170770859E-16,0.,1.));
#30782=DIRECTION('center_axis',(1.,0.,0.));
#30783=DIRECTION('ref_axis',(0.,-0.707106781186548,-0.707106781186548));
#30784=DIRECTION('',(1.,0.,0.));
#30785=DIRECTION('center_axis',(0.,0.,-1.));
#30786=DIRECTION('ref_axis',(1.,0.,0.));
#30787=DIRECTION('',(-1.,0.,0.));
#30788=DIRECTION('',(0.,1.,0.));
#30789=DIRECTION('',(0.707106781186548,0.,0.707106781186547));
#30790=DIRECTION('center_axis',(0.707106781186552,0.,-0.707106781186543));
#30791=DIRECTION('ref_axis',(-0.707106781186543,0.,-0.707106781186552));
#30792=DIRECTION('',(-0.707106781186543,0.,-0.707106781186552));
#30793=DIRECTION('',(0.,-1.,0.));
#30794=DIRECTION('center_axis',(1.85037170770859E-16,0.,1.));
#30795=DIRECTION('ref_axis',(0.707106781186547,-0.707106781186548,0.));
#30796=DIRECTION('',(1.85037170770859E-16,0.,1.));
#30797=DIRECTION('center_axis',(1.,0.,-1.85037170770859E-16));
#30798=DIRECTION('ref_axis',(1.85037170770859E-16,0.,1.));
#30799=DIRECTION('',(-1.85037170770859E-16,0.,-1.));
#30800=DIRECTION('',(0.,1.,0.));
#30801=DIRECTION('',(0.707106781186547,0.,0.707106781186548));
#30802=DIRECTION('',(-0.707106781186546,0.,-0.707106781186549));
#30803=DIRECTION('center_axis',(-0.707106781186549,0.,0.707106781186546));
#30804=DIRECTION('ref_axis',(0.707106781186546,0.,0.707106781186549));
#30805=DIRECTION('',(0.707106781186546,0.,0.707106781186549));
#30806=DIRECTION('',(0.,-1.,0.));
#30807=DIRECTION('',(0.,1.,0.));
#30808=DIRECTION('center_axis',(0.,-1.,0.));
#30809=DIRECTION('ref_axis',(0.,0.,-1.));
#30810=DIRECTION('',(0.,0.,1.));
#30811=DIRECTION('',(-1.,0.,1.15648231731787E-16));
#30812=DIRECTION('center_axis',(0.,-1.,0.));
#30813=DIRECTION('ref_axis',(0.,0.,1.));
#30814=DIRECTION('',(1.,0.,-9.25185853854297E-17));
#30815=DIRECTION('center_axis',(0.,0.,-1.));
#30816=DIRECTION('ref_axis',(-0.707106781186548,-0.707106781186548,0.));
#30817=DIRECTION('',(0.,0.,-1.));
#30818=DIRECTION('center_axis',(0.,-3.70074341541719E-16,1.));
#30819=DIRECTION('ref_axis',(-1.,0.,0.));
#30820=DIRECTION('center_axis',(-1.,0.,0.));
#30821=DIRECTION('ref_axis',(0.,0.,-1.));
#30822=DIRECTION('',(0.,0.,1.));
#30823=DIRECTION('',(0.,1.,0.));
#30824=DIRECTION('',(0.707106781186548,0.,-0.707106781186547));
#30825=DIRECTION('',(-0.707106781186549,0.,0.707106781186546));
#30826=DIRECTION('center_axis',(0.707106781186546,0.,0.707106781186549));
#30827=DIRECTION('ref_axis',(0.707106781186549,0.,-0.707106781186546));
#30828=DIRECTION('',(0.707106781186549,0.,-0.707106781186546));
#30829=DIRECTION('',(0.,-1.,0.));
#30830=DIRECTION('',(0.,1.,0.));
#30831=DIRECTION('center_axis',(0.,-1.,0.));
#30832=DIRECTION('ref_axis',(0.,0.,-1.));
#30833=DIRECTION('',(1.,0.,0.));
#30834=DIRECTION('',(0.707106781186549,0.,0.707106781186546));
#30835=DIRECTION('',(6.93889390390723E-17,0.,1.));
#30836=DIRECTION('center_axis',(0.,-1.,0.));
#30837=DIRECTION('ref_axis',(0.,0.,1.));
#30838=DIRECTION('',(-9.25185853854297E-17,0.,-1.));
#30839=DIRECTION('center_axis',(-1.,0.,0.));
#30840=DIRECTION('ref_axis',(0.,-0.707106781186548,0.707106781186548));
#30841=DIRECTION('',(-1.,0.,0.));
#30842=DIRECTION('center_axis',(0.,0.,1.));
#30843=DIRECTION('ref_axis',(-1.,0.,0.));
#30844=DIRECTION('',(1.,0.,0.));
#30845=DIRECTION('',(0.,1.,0.));
#30846=DIRECTION('',(-0.707106781186548,0.,-0.707106781186547));
#30847=DIRECTION('center_axis',(-0.707106781186552,0.,0.707106781186543));
#30848=DIRECTION('ref_axis',(0.707106781186543,0.,0.707106781186552));
#30849=DIRECTION('',(0.707106781186543,0.,0.707106781186552));
#30850=DIRECTION('',(0.,-1.,0.));
#30851=DIRECTION('center_axis',(-6.93889390390723E-17,0.,-1.));
#30852=DIRECTION('ref_axis',(-0.707106781186547,-0.707106781186548,0.));
#30853=DIRECTION('',(-6.93889390390723E-17,0.,-1.));
#30854=DIRECTION('center_axis',(-1.,0.,6.93889390390723E-17));
#30855=DIRECTION('ref_axis',(-6.93889390390723E-17,0.,-1.));
#30856=DIRECTION('',(6.93889390390723E-17,0.,1.));
#30857=DIRECTION('',(0.,1.,0.));
#30858=DIRECTION('',(-0.707106781186547,0.,-0.707106781186548));
#30859=DIRECTION('',(0.707106781186544,0.,0.707106781186551));
#30860=DIRECTION('center_axis',(0.707106781186549,0.,-0.707106781186546));
#30861=DIRECTION('ref_axis',(-0.707106781186546,0.,-0.707106781186549));
#30862=DIRECTION('',(-0.707106781186546,0.,-0.707106781186549));
#30863=DIRECTION('',(0.,-1.,0.));
#30864=DIRECTION('',(0.,1.,0.));
#30865=DIRECTION('center_axis',(0.,-1.,0.));
#30866=DIRECTION('ref_axis',(0.,0.,-1.));
#30867=DIRECTION('',(0.,0.,-1.));
#30868=DIRECTION('',(0.707106781186546,0.,-0.707106781186549));
#30869=DIRECTION('',(1.,0.,0.));
#30870=DIRECTION('center_axis',(0.,-1.,0.));
#30871=DIRECTION('ref_axis',(0.,0.,1.));
#30872=DIRECTION('',(-1.,0.,0.));
#30873=DIRECTION('center_axis',(0.,0.,1.));
#30874=DIRECTION('ref_axis',(0.707106781186548,-0.707106781186548,0.));
#30875=DIRECTION('',(0.,0.,1.));
#30876=DIRECTION('center_axis',(1.,0.,0.));
#30877=DIRECTION('ref_axis',(0.,0.,1.));
#30878=DIRECTION('',(0.,0.,-1.));
#30879=DIRECTION('',(0.,1.,0.));
#30880=DIRECTION('',(-0.707106781186546,0.,0.707106781186549));
#30881=DIRECTION('center_axis',(0.707106781186543,0.,0.707106781186552));
#30882=DIRECTION('ref_axis',(0.707106781186552,0.,-0.707106781186543));
#30883=DIRECTION('',(0.707106781186552,0.,-0.707106781186543));
#30884=DIRECTION('',(0.,-1.,0.));
#30885=DIRECTION('center_axis',(-1.,0.,0.));
#30886=DIRECTION('ref_axis',(0.,-0.707106781186548,0.707106781186547));
#30887=DIRECTION('',(-1.,0.,0.));
#30888=DIRECTION('center_axis',(0.,0.,1.));
#30889=DIRECTION('ref_axis',(-1.,0.,0.));
#30890=DIRECTION('',(1.,0.,0.));
#30891=DIRECTION('',(0.,1.,0.));
#30892=DIRECTION('center_axis',(0.,1.,0.));
#30893=DIRECTION('ref_axis',(0.,0.,1.));
#30894=DIRECTION('center_axis',(0.,-1.,0.));
#30895=DIRECTION('ref_axis',(6.12323399573676E-17,0.,-1.));
#30896=DIRECTION('center_axis',(-1.,0.,1.22464679914735E-16));
#30897=DIRECTION('ref_axis',(-1.22464679914735E-16,0.,-1.));
#30898=DIRECTION('center_axis',(0.,1.,0.));
#30899=DIRECTION('ref_axis',(-3.06161699786838E-17,0.,-1.));
#30900=DIRECTION('center_axis',(0.,1.,0.));
#30901=DIRECTION('ref_axis',(0.,0.,1.));
#30902=DIRECTION('',(8.65956056235492E-17,-0.707106781186548,0.707106781186547));
#30903=DIRECTION('center_axis',(0.,-1.,0.));
#30904=DIRECTION('ref_axis',(-3.06161699786838E-17,0.,-1.));
#30905=DIRECTION('center_axis',(0.,1.,0.));
#30906=DIRECTION('ref_axis',(0.,0.,1.));
#30907=DIRECTION('center_axis',(0.,1.,0.));
#30908=DIRECTION('ref_axis',(6.12323399573676E-17,0.,-1.));
#30909=DIRECTION('',(0.,-1.,0.));
#30910=DIRECTION('center_axis',(0.,1.,0.));
#30911=DIRECTION('ref_axis',(0.,0.,1.));
#30912=DIRECTION('center_axis',(-1.,0.,1.22464679914735E-16));
#30913=DIRECTION('ref_axis',(-1.22464679914735E-16,0.,-1.));
#30914=DIRECTION('center_axis',(0.,1.,0.));
#30915=DIRECTION('ref_axis',(6.12323399573677E-17,0.,-1.));
#30916=DIRECTION('center_axis',(0.,-1.,0.));
#30917=DIRECTION('ref_axis',(0.,0.,-1.));
#30918=DIRECTION('center_axis',(0.,1.,0.));
#30919=DIRECTION('ref_axis',(1.,0.,0.));
#30920=DIRECTION('center_axis',(0.,1.,0.));
#30921=DIRECTION('ref_axis',(1.,0.,0.));
#30922=DIRECTION('center_axis',(0.,1.,0.));
#30923=DIRECTION('ref_axis',(1.,0.,0.));
#30924=DIRECTION('center_axis',(0.,1.,0.));
#30925=DIRECTION('ref_axis',(1.,0.,0.));
#30926=DIRECTION('center_axis',(0.,1.,0.));
#30927=DIRECTION('ref_axis',(1.,0.,0.));
#30928=DIRECTION('center_axis',(0.,1.,0.));
#30929=DIRECTION('ref_axis',(1.,0.,0.));
#30930=DIRECTION('center_axis',(0.,1.,0.));
#30931=DIRECTION('ref_axis',(1.,0.,0.));
#30932=DIRECTION('center_axis',(0.,1.,0.));
#30933=DIRECTION('ref_axis',(1.,0.,0.));
#30934=DIRECTION('',(1.85037170770859E-16,0.,1.));
#30935=DIRECTION('center_axis',(0.,1.,0.));
#30936=DIRECTION('ref_axis',(0.,0.,1.));
#30937=DIRECTION('',(-1.,0.,1.15648231731787E-16));
#30938=DIRECTION('center_axis',(0.,1.,0.));
#30939=DIRECTION('ref_axis',(-0.707106781186548,0.,-0.707106781186547));
#30940=DIRECTION('',(1.,0.,-9.25185853854297E-17));
#30941=DIRECTION('center_axis',(0.,1.,0.));
#30942=DIRECTION('ref_axis',(0.,0.,1.));
#30943=DIRECTION('',(-9.25185853854297E-17,0.,-1.));
#30944=DIRECTION('center_axis',(0.,1.,0.));
#30945=DIRECTION('ref_axis',(0.,0.,1.));
#30946=DIRECTION('',(-1.,0.,0.));
#30947=DIRECTION('center_axis',(0.,1.,0.));
#30948=DIRECTION('ref_axis',(0.,0.,1.));
#30949=DIRECTION('center_axis',(1.,0.,0.));
#30950=DIRECTION('ref_axis',(0.,-0.707106781186548,-0.707106781186547));
#30951=DIRECTION('',(1.,0.,0.));
#30952=DIRECTION('center_axis',(0.,0.,-1.));
#30953=DIRECTION('ref_axis',(1.,0.,0.));
#30954=DIRECTION('',(0.,-1.,0.));
#30955=DIRECTION('center_axis',(9.25185853854297E-17,0.,1.));
#30956=DIRECTION('ref_axis',(0.707106781186547,-0.707106781186548,0.));
#30957=DIRECTION('',(9.25185853854297E-17,0.,1.));
#30958=DIRECTION('center_axis',(1.,0.,-9.25185853854297E-17));
#30959=DIRECTION('ref_axis',(9.25185853854297E-17,0.,1.));
#30960=DIRECTION('',(0.,-1.,0.));
#30961=DIRECTION('center_axis',(0.,1.,0.));
#30962=DIRECTION('ref_axis',(0.,0.,1.));
#30963=DIRECTION('center_axis',(0.,-1.,0.));
#30964=DIRECTION('ref_axis',(6.12323399573677E-17,0.,-1.));
#30965=DIRECTION('center_axis',(-1.,0.,1.22464679914735E-16));
#30966=DIRECTION('ref_axis',(-1.22464679914735E-16,0.,-1.));
#30967=DIRECTION('center_axis',(0.,1.,0.));
#30968=DIRECTION('ref_axis',(0.,0.,1.));
#30969=DIRECTION('center_axis',(0.,1.,0.));
#30970=DIRECTION('ref_axis',(0.,0.,1.));
#30971=DIRECTION('center_axis',(0.,-1.,0.));
#30972=DIRECTION('ref_axis',(1.,0.,0.));
#30973=DIRECTION('center_axis',(0.,-1.,0.));
#30974=DIRECTION('ref_axis',(1.,0.,0.));
#30975=DIRECTION('center_axis',(0.,1.,0.));
#30976=DIRECTION('ref_axis',(0.,0.,1.));
#30977=DIRECTION('center_axis',(0.,-1.,0.));
#30978=DIRECTION('ref_axis',(1.,0.,0.));
#30979=DIRECTION('center_axis',(0.,-1.,0.));
#30980=DIRECTION('ref_axis',(1.,0.,0.));
#30981=DIRECTION('center_axis',(0.,1.,0.));
#30982=DIRECTION('ref_axis',(0.,0.,1.));
#30983=DIRECTION('center_axis',(0.,-1.,0.));
#30984=DIRECTION('ref_axis',(1.,0.,0.));
#30985=DIRECTION('center_axis',(0.,-1.,0.));
#30986=DIRECTION('ref_axis',(1.,0.,0.));
#30987=DIRECTION('center_axis',(0.,1.,0.));
#30988=DIRECTION('ref_axis',(0.,0.,1.));
#30989=DIRECTION('center_axis',(0.,-1.,0.));
#30990=DIRECTION('ref_axis',(1.,0.,0.));
#30991=DIRECTION('center_axis',(0.,-1.,0.));
#30992=DIRECTION('ref_axis',(1.,0.,0.));
#30993=DIRECTION('center_axis',(0.,1.,0.));
#30994=DIRECTION('ref_axis',(0.,0.,1.));
#30995=DIRECTION('center_axis',(0.,-1.,0.));
#30996=DIRECTION('ref_axis',(1.,0.,0.));
#30997=DIRECTION('center_axis',(0.,-1.,0.));
#30998=DIRECTION('ref_axis',(1.,0.,0.));
#30999=DIRECTION('center_axis',(0.,1.,0.));
#31000=DIRECTION('ref_axis',(0.,0.,1.));
#31001=DIRECTION('center_axis',(0.,-1.,0.));
#31002=DIRECTION('ref_axis',(1.,0.,0.));
#31003=DIRECTION('center_axis',(0.,-1.,0.));
#31004=DIRECTION('ref_axis',(1.,0.,0.));
#31005=DIRECTION('center_axis',(0.,1.,0.));
#31006=DIRECTION('ref_axis',(0.,0.,1.));
#31007=DIRECTION('center_axis',(0.,1.,0.));
#31008=DIRECTION('ref_axis',(0.,0.,1.));
#31009=DIRECTION('center_axis',(0.,-1.,0.));
#31010=DIRECTION('ref_axis',(1.,0.,0.));
#31011=DIRECTION('center_axis',(0.,-1.,0.));
#31012=DIRECTION('ref_axis',(1.,0.,0.));
#31013=DIRECTION('center_axis',(0.,1.,0.));
#31014=DIRECTION('ref_axis',(0.,0.,1.));
#31015=DIRECTION('center_axis',(0.,-1.,0.));
#31016=DIRECTION('ref_axis',(1.,0.,0.));
#31017=DIRECTION('center_axis',(0.,-1.,0.));
#31018=DIRECTION('ref_axis',(1.,0.,0.));
#31019=DIRECTION('center_axis',(0.,1.,0.));
#31020=DIRECTION('ref_axis',(0.,0.,1.));
#31021=DIRECTION('center_axis',(0.,-1.,0.));
#31022=DIRECTION('ref_axis',(-3.06161699786838E-17,0.,-1.));
#31023=DIRECTION('center_axis',(-1.,0.,1.22464679914735E-16));
#31024=DIRECTION('ref_axis',(-1.22464679914735E-16,0.,-1.));
#31025=DIRECTION('center_axis',(0.,1.,0.));
#31026=DIRECTION('ref_axis',(6.12323399573677E-17,0.,-1.));
#31027=DIRECTION('center_axis',(0.,1.,0.));
#31028=DIRECTION('ref_axis',(0.,0.,1.));
#31029=DIRECTION('center_axis',(0.,1.,0.));
#31030=DIRECTION('ref_axis',(-3.06161699786838E-17,0.,-1.));
#31031=DIRECTION('',(8.65956056235495E-17,-0.707106781186546,0.707106781186549));
#31032=DIRECTION('center_axis',(0.,-1.,0.));
#31033=DIRECTION('ref_axis',(0.,0.,-1.));
#31034=DIRECTION('',(0.996199654101518,0.,0.0870990767345742));
#31035=DIRECTION('',(-0.997179284808876,0.,-0.0750564717266851));
#31036=DIRECTION('',(-0.569209969005557,0.,-0.822192198445529));
#31037=DIRECTION('',(0.,0.,-1.));
#31038=DIRECTION('',(-1.,0.,0.));
#31039=DIRECTION('',(0.,0.,1.));
#31040=DIRECTION('',(-0.555834771638921,0.,0.831292792364464));
#31041=DIRECTION('',(1.,0.,0.));
#31042=DIRECTION('',(0.547249318401935,0.,-0.836969643122507));
#31043=DIRECTION('',(0.550221176517859,0.,0.835018956019145));
#31044=DIRECTION('',(1.,0.,0.));
#31045=DIRECTION('',(1.,0.,0.));
#31046=DIRECTION('',(0.,0.,-1.));
#31047=DIRECTION('',(-1.,0.,0.));
#31048=DIRECTION('',(0.,0.,-1.));
#31049=DIRECTION('',(1.,0.,0.));
#31050=DIRECTION('',(0.,0.,-1.));
#31051=DIRECTION('',(-1.,0.,0.));
#31052=DIRECTION('',(0.,0.,-1.));
#31053=DIRECTION('',(1.,0.,0.));
#31054=DIRECTION('',(0.,0.,-1.));
#31055=DIRECTION('',(1.,0.,0.));
#31056=DIRECTION('',(0.,0.,-1.));
#31057=DIRECTION('',(1.,0.,0.));
#31058=DIRECTION('',(1.,0.,0.));
#31059=DIRECTION('',(0.,0.,-1.));
#31060=DIRECTION('',(1.,0.,0.));
#31061=DIRECTION('',(0.53851434427711,0.,-0.842616342713452));
#31062=DIRECTION('',(-0.358509645558692,0.,-0.933526022155452));
#31063=DIRECTION('',(-1.,0.,0.));
#31064=DIRECTION('',(-0.378780343133087,0.,0.925486602634517));
#31065=DIRECTION('',(-1.,0.,0.));
#31066=DIRECTION('',(-0.359401529578064,0.,0.933183015563907));
#31067=DIRECTION('',(-1.,0.,0.));
#31068=DIRECTION('',(-0.340892911214198,0.,-0.940102134389614));
#31069=DIRECTION('',(-1.,0.,0.));
#31070=DIRECTION('',(-0.536696416993486,0.,0.843775417979425));
#31071=DIRECTION('',(-1.,0.,0.));
#31072=DIRECTION('',(0.,0.,-1.));
#31073=DIRECTION('',(1.,0.,0.));
#31074=DIRECTION('',(0.,0.,-1.));
#31075=DIRECTION('center_axis',(-1.,0.,9.25185853854297E-17));
#31076=DIRECTION('ref_axis',(0.,-0.707106781186548,0.707106781186547));
#31077=DIRECTION('',(-1.,0.,9.25185853854297E-17));
#31078=DIRECTION('center_axis',(0.,-1.,0.));
#31079=DIRECTION('ref_axis',(-0.707106781186548,0.,-0.707106781186547));
#31080=DIRECTION('center_axis',(0.,1.,0.));
#31081=DIRECTION('ref_axis',(0.,0.,-1.));
#31082=DIRECTION('',(0.,-1.,0.));
#31083=DIRECTION('center_axis',(0.40824829046386,0.408248290463862,-0.816496580927728));
#31084=DIRECTION('ref_axis',(-0.577350269189624,-0.577350269189627,-0.577350269189626));
#31085=DIRECTION('center_axis',(-1.,0.,1.15648231731787E-16));
#31086=DIRECTION('ref_axis',(0.,-0.707106781186549,-0.707106781186546));
#31087=DIRECTION('center_axis',(1.,0.,-1.15648231731787E-16));
#31088=DIRECTION('ref_axis',(0.,-0.707106781186548,-0.707106781186547));
#31089=DIRECTION('',(1.,0.,-1.15648231731787E-16));
#31090=DIRECTION('center_axis',(-1.15648231731787E-16,0.,-1.));
#31091=DIRECTION('ref_axis',(1.,0.,-1.15648231731787E-16));
#31092=DIRECTION('',(0.,1.,0.));
#31093=DIRECTION('center_axis',(0.,1.,0.));
#31094=DIRECTION('ref_axis',(0.,0.,1.));
#31095=DIRECTION('center_axis',(0.,-1.,0.));
#31096=DIRECTION('ref_axis',(6.12323399573677E-17,0.,-1.));
#31097=DIRECTION('center_axis',(-1.,0.,1.22464679914735E-16));
#31098=DIRECTION('ref_axis',(-1.22464679914735E-16,0.,-1.));
#31099=DIRECTION('center_axis',(0.,1.,0.));
#31100=DIRECTION('ref_axis',(0.,0.,1.));
#31101=DIRECTION('',(0.,-1.,0.));
#31102=DIRECTION('',(0.,-1.,0.));
#31103=DIRECTION('',(0.,-1.,0.));
#31104=DIRECTION('center_axis',(-1.85037170770859E-16,0.,-1.));
#31105=DIRECTION('ref_axis',(-0.707106781186547,-0.707106781186548,0.));
#31106=DIRECTION('',(-1.85037170770859E-16,0.,-1.));
#31107=DIRECTION('center_axis',(-1.,0.,1.85037170770859E-16));
#31108=DIRECTION('ref_axis',(-1.85037170770859E-16,0.,-1.));
#31109=DIRECTION('center_axis',(0.,1.,0.));
#31110=DIRECTION('ref_axis',(-1.22464679914735E-16,0.,-1.));
#31111=DIRECTION('center_axis',(0.,-1.,0.));
#31112=DIRECTION('ref_axis',(1.94775969232484E-16,0.,-1.));
#31113=DIRECTION('center_axis',(0.,1.,0.));
#31114=DIRECTION('ref_axis',(1.94775969232484E-16,0.,-1.));
#31115=DIRECTION('center_axis',(-0.499999999999999,0.,-0.866025403784439));
#31116=DIRECTION('ref_axis',(0.612372435695794,0.707106781186546,-0.353553390593278));
#31117=DIRECTION('',(0.499999999999999,0.,0.866025403784439));
#31118=DIRECTION('',(-0.499999999999999,0.,-0.866025403784439));
#31119=DIRECTION('center_axis',(-0.5,0.,0.866025403784439));
#31120=DIRECTION('ref_axis',(-0.612372435695794,0.707106781186546,-0.353553390593278));
#31121=DIRECTION('',(-0.5,0.,0.866025403784439));
#31122=DIRECTION('',(0.5,0.,-0.866025403784439));
#31123=DIRECTION('center_axis',(0.,-1.,0.));
#31124=DIRECTION('ref_axis',(0.,0.,-1.));
#31125=DIRECTION('center_axis',(0.,1.,0.));
#31126=DIRECTION('ref_axis',(1.,0.,0.));
#31127=DIRECTION('center_axis',(0.,1.,0.));
#31128=DIRECTION('ref_axis',(2.13501882696539E-19,0.,-1.));
#31129=DIRECTION('center_axis',(0.,-1.,0.));
#31130=DIRECTION('ref_axis',(2.13501882696539E-19,0.,-1.));
#31131=DIRECTION('center_axis',(0.,-1.,0.));
#31132=DIRECTION('ref_axis',(2.13501882696539E-19,0.,-1.));
#31133=DIRECTION('center_axis',(1.,0.,1.22678181797432E-16));
#31134=DIRECTION('ref_axis',(-1.22678181797432E-16,0.,1.));
#31135=DIRECTION('center_axis',(0.,1.,0.));
#31136=DIRECTION('ref_axis',(1.,0.,0.));
#31137=DIRECTION('center_axis',(0.,1.,0.));
#31138=DIRECTION('ref_axis',(0.,0.,1.));
#31139=DIRECTION('',(0.,-1.,0.));
#31140=DIRECTION('center_axis',(0.,-1.,0.));
#31141=DIRECTION('ref_axis',(0.5,0.,0.866025403784439));
#31142=DIRECTION('',(0.,1.,0.));
#31143=DIRECTION('center_axis',(0.,-1.,0.));
#31144=DIRECTION('ref_axis',(0.5,0.,0.866025403784439));
#31145=DIRECTION('',(0.,-1.,0.));
#31146=DIRECTION('center_axis',(0.,-1.,0.));
#31147=DIRECTION('ref_axis',(0.,0.,-1.));
#31148=DIRECTION('center_axis',(-1.,0.,-1.22464679914735E-16));
#31149=DIRECTION('ref_axis',(-1.22464679914735E-16,0.,1.));
#31150=DIRECTION('center_axis',(0.,-1.,0.));
#31151=DIRECTION('ref_axis',(0.,0.,1.));
#31152=DIRECTION('center_axis',(0.,-1.,0.));
#31153=DIRECTION('ref_axis',(0.,0.,1.));
#31154=DIRECTION('center_axis',(0.,1.,0.));
#31155=DIRECTION('ref_axis',(1.,0.,0.));
#31156=DIRECTION('',(0.,1.,0.));
#31157=DIRECTION('center_axis',(0.,1.,0.));
#31158=DIRECTION('ref_axis',(1.,0.,0.));
#31159=DIRECTION('',(0.,1.,0.));
#31160=DIRECTION('center_axis',(0.,1.,0.));
#31161=DIRECTION('ref_axis',(1.,0.,0.));
#31162=DIRECTION('',(0.,1.,0.));
#31163=DIRECTION('center_axis',(0.,1.,0.));
#31164=DIRECTION('ref_axis',(1.,0.,0.));
#31165=DIRECTION('',(0.,1.,0.));
#31166=DIRECTION('center_axis',(0.,1.,0.));
#31167=DIRECTION('ref_axis',(0.,0.,1.));
#31168=DIRECTION('center_axis',(0.,1.,0.));
#31169=DIRECTION('ref_axis',(1.,0.,0.));
#31170=DIRECTION('',(0.,1.,0.));
#31171=DIRECTION('center_axis',(0.,0.,-1.));
#31172=DIRECTION('ref_axis',(0.745355992499931,-0.666666666666666,0.));
#31173=DIRECTION('center_axis',(0.,0.,1.));
#31174=DIRECTION('ref_axis',(0.745355992499931,-0.666666666666666,0.));
#31175=DIRECTION('center_axis',(0.,0.,-1.));
#31176=DIRECTION('ref_axis',(0.745355992499931,-0.666666666666666,0.));
#31177=DIRECTION('',(0.,0.,1.));
#31178=DIRECTION('center_axis',(0.,0.,-1.));
#31179=DIRECTION('ref_axis',(0.745355992499931,-0.666666666666666,0.));
#31180=DIRECTION('center_axis',(0.,0.,1.));
#31181=DIRECTION('ref_axis',(0.745355992499931,-0.666666666666666,0.));
#31182=DIRECTION('center_axis',(0.,0.,-1.));
#31183=DIRECTION('ref_axis',(0.745355992499931,-0.666666666666666,0.));
#31184=DIRECTION('',(0.,0.,1.));
#31185=DIRECTION('center_axis',(0.,0.,-1.));
#31186=DIRECTION('ref_axis',(0.745355992499931,-0.666666666666666,0.));
#31187=DIRECTION('center_axis',(0.,0.,1.));
#31188=DIRECTION('ref_axis',(0.745355992499931,-0.666666666666666,0.));
#31189=DIRECTION('center_axis',(0.,0.,-1.));
#31190=DIRECTION('ref_axis',(0.745355992499931,-0.666666666666666,0.));
#31191=DIRECTION('',(0.,0.,1.));
#31192=DIRECTION('center_axis',(-0.358509645558692,0.,-0.933526022155452));
#31193=DIRECTION('ref_axis',(0.695809214768189,-0.666666666666666,-0.267217312686197));
#31194=DIRECTION('center_axis',(0.,0.,1.));
#31195=DIRECTION('ref_axis',(1.,6.90948055922478E-16,0.));
#31196=DIRECTION('center_axis',(0.842616342713453,0.,0.53851434427711));
#31197=DIRECTION('ref_axis',(0.53851434427711,7.44592572834826E-17,-0.842616342713453));
#31198=DIRECTION('center_axis',(0.,0.,-1.));
#31199=DIRECTION('ref_axis',(1.,6.90948055922478E-16,0.));
#31200=DIRECTION('',(0.358509645558692,0.,0.933526022155452));
#31201=DIRECTION('center_axis',(-0.378780343133087,0.,0.925486602634517));
#31202=DIRECTION('ref_axis',(-0.68981698525204,-0.666666666666666,-0.282326198595426));
#31203=DIRECTION('center_axis',(0.,0.,-1.));
#31204=DIRECTION('ref_axis',(-1.,-1.71249422537826E-16,0.));
#31205=DIRECTION('center_axis',(0.,0.,1.));
#31206=DIRECTION('ref_axis',(-1.,-1.71249422537826E-16,0.));
#31207=DIRECTION('',(0.378780343133087,0.,-0.925486602634517));
#31208=DIRECTION('center_axis',(0.,0.,-1.));
#31209=DIRECTION('ref_axis',(-1.,0.,0.));
#31210=DIRECTION('',(0.,1.,0.));
#31211=DIRECTION('',(-1.,0.,0.));
#31212=DIRECTION('',(0.,1.,0.));
#31213=DIRECTION('center_axis',(-0.933183015563908,0.,-0.359401529578064));
#31214=DIRECTION('ref_axis',(-0.359401529578064,0.,0.933183015563907));
#31215=DIRECTION('',(0.,1.,0.));
#31216=DIRECTION('',(-0.359401529578064,0.,0.933183015563907));
#31217=DIRECTION('center_axis',(0.,0.,-1.));
#31218=DIRECTION('ref_axis',(-1.,0.,0.));
#31219=DIRECTION('',(-1.,0.,0.));
#31220=DIRECTION('center_axis',(0.,0.,1.));
#31221=DIRECTION('ref_axis',(1.,0.,0.));
#31222=DIRECTION('',(1.,0.,0.));
#31223=DIRECTION('center_axis',(0.,0.,-1.));
#31224=DIRECTION('ref_axis',(-1.,0.,0.));
#31225=DIRECTION('',(0.,1.,0.));
#31226=DIRECTION('',(-1.,0.,0.));
#31227=DIRECTION('',(0.,1.,0.));
#31228=DIRECTION('',(-1.,0.,0.));
#31229=DIRECTION('',(0.,1.,0.));
#31230=DIRECTION('center_axis',(0.940102134389614,0.,-0.340892911214198));
#31231=DIRECTION('ref_axis',(-0.340892911214198,0.,-0.940102134389614));
#31232=DIRECTION('',(-0.340892911214198,0.,-0.940102134389614));
#31233=DIRECTION('center_axis',(0.,1.,0.));
#31234=DIRECTION('ref_axis',(0.,0.,1.));
#31235=DIRECTION('center_axis',(0.,0.,1.));
#31236=DIRECTION('ref_axis',(1.,0.,0.));
#31237=DIRECTION('',(0.,1.,0.));
#31238=DIRECTION('',(1.,0.,0.));
#31239=DIRECTION('',(0.,1.,0.));
#31240=DIRECTION('center_axis',(1.,0.,0.));
#31241=DIRECTION('ref_axis',(0.,0.,-1.));
#31242=DIRECTION('',(0.,1.,0.));
#31243=DIRECTION('',(0.,0.,-1.));
#31244=DIRECTION('center_axis',(0.,0.,-1.));
#31245=DIRECTION('ref_axis',(-1.,0.,0.));
#31246=DIRECTION('',(0.,1.,0.));
#31247=DIRECTION('',(-1.,0.,0.));
#31248=DIRECTION('center_axis',(1.,0.,0.));
#31249=DIRECTION('ref_axis',(0.,0.,-1.));
#31250=DIRECTION('',(0.,1.,0.));
#31251=DIRECTION('',(0.,0.,-1.));
#31252=DIRECTION('center_axis',(0.,0.,1.));
#31253=DIRECTION('ref_axis',(1.,0.,0.));
#31254=DIRECTION('',(0.,1.,0.));
#31255=DIRECTION('',(1.,0.,0.));
#31256=DIRECTION('center_axis',(1.,0.,0.));
#31257=DIRECTION('ref_axis',(0.,0.,-1.));
#31258=DIRECTION('',(0.,1.,0.));
#31259=DIRECTION('',(0.,0.,-1.));
#31260=DIRECTION('center_axis',(0.,0.,-1.));
#31261=DIRECTION('ref_axis',(-1.,0.,0.));
#31262=DIRECTION('',(0.,1.,0.));
#31263=DIRECTION('',(-1.,0.,0.));
#31264=DIRECTION('center_axis',(1.,0.,0.));
#31265=DIRECTION('ref_axis',(0.,0.,-1.));
#31266=DIRECTION('',(0.,1.,0.));
#31267=DIRECTION('',(0.,0.,-1.));
#31268=DIRECTION('center_axis',(0.,0.,1.));
#31269=DIRECTION('ref_axis',(1.,0.,0.));
#31270=DIRECTION('',(1.,0.,0.));
#31271=DIRECTION('center_axis',(0.,0.,-1.));
#31272=DIRECTION('ref_axis',(-1.,0.,0.));
#31273=DIRECTION('',(0.,1.,0.));
#31274=DIRECTION('',(-1.,0.,0.));
#31275=DIRECTION('center_axis',(1.,0.,0.));
#31276=DIRECTION('ref_axis',(0.,0.,-1.));
#31277=DIRECTION('',(0.,0.,-1.));
#31278=DIRECTION('center_axis',(0.,1.,0.));
#31279=DIRECTION('ref_axis',(0.,0.,1.));
#31280=DIRECTION('',(0.,1.,0.));
#31281=DIRECTION('',(0.,1.,0.));
#31282=DIRECTION('',(0.,1.,0.));
#31283=DIRECTION('',(0.,1.,0.));
#31284=DIRECTION('',(0.,1.,0.));
#31285=DIRECTION('',(0.,1.,0.));
#31286=DIRECTION('',(0.,1.,0.));
#31287=DIRECTION('',(0.,1.,0.));
#31288=DIRECTION('',(0.,1.,0.));
#31289=DIRECTION('',(0.,1.,0.));
#31290=DIRECTION('',(0.,1.,0.));
#31291=DIRECTION('center_axis',(0.,0.,1.));
#31292=DIRECTION('ref_axis',(1.,0.,0.));
#31293=DIRECTION('',(1.,0.,0.));
#31294=DIRECTION('center_axis',(0.,0.,-1.));
#31295=DIRECTION('ref_axis',(-1.,0.,0.));
#31296=DIRECTION('',(0.,1.,0.));
#31297=DIRECTION('',(-1.,0.,0.));
#31298=DIRECTION('center_axis',(0.,-1.,0.));
#31299=DIRECTION('ref_axis',(0.,0.,-1.));
#31300=DIRECTION('',(0.,1.,0.));
#31301=DIRECTION('',(0.,1.,0.));
#31302=DIRECTION('',(0.,1.,0.));
#31303=DIRECTION('',(0.,1.,0.));
#31304=DIRECTION('',(0.,1.,0.));
#31305=DIRECTION('',(0.,1.,0.));
#31306=DIRECTION('',(0.,1.,0.));
#31307=DIRECTION('',(0.,1.,0.));
#31308=DIRECTION('',(0.,1.,0.));
#31309=DIRECTION('',(0.,1.,0.));
#31310=DIRECTION('',(0.,1.,0.));
#31311=DIRECTION('',(0.,1.,0.));
#31312=DIRECTION('',(0.,1.,0.));
#31313=DIRECTION('',(0.,1.,0.));
#31314=DIRECTION('center_axis',(0.0750564717266851,0.,-0.997179284808876));
#31315=DIRECTION('ref_axis',(-0.997179284808876,0.,-0.0750564717266851));
#31316=DIRECTION('',(0.,1.,0.));
#31317=DIRECTION('',(-0.997179284808876,0.,-0.0750564717266851));
#31318=DIRECTION('',(0.,1.,0.));
#31319=DIRECTION('',(0.,1.,0.));
#31320=DIRECTION('',(0.,1.,0.));
#31321=DIRECTION('',(0.,1.,0.));
#31322=DIRECTION('',(0.,1.,0.));
#31323=DIRECTION('',(0.,1.,0.));
#31324=DIRECTION('',(0.,1.,0.));
#31325=DIRECTION('',(0.,1.,0.));
#31326=DIRECTION('',(0.,1.,0.));
#31327=DIRECTION('',(0.,1.,0.));
#31328=DIRECTION('',(0.,1.,0.));
#31329=DIRECTION('',(0.,1.,0.));
#31330=DIRECTION('',(0.,1.,0.));
#31331=DIRECTION('',(0.,1.,0.));
#31332=DIRECTION('',(0.,1.,0.));
#31333=DIRECTION('',(0.,1.,0.));
#31334=DIRECTION('',(0.,1.,0.));
#31335=DIRECTION('',(0.,1.,0.));
#31336=DIRECTION('center_axis',(-0.0870990767345742,0.,0.996199654101518));
#31337=DIRECTION('ref_axis',(0.996199654101518,0.,0.0870990767345742));
#31338=DIRECTION('',(0.,1.,0.));
#31339=DIRECTION('',(0.996199654101518,0.,0.0870990767345742));
#31340=DIRECTION('',(0.,1.,0.));
#31341=DIRECTION('center_axis',(0.,-1.,0.));
#31342=DIRECTION('ref_axis',(0.,0.,-1.));
#31343=DIRECTION('center_axis',(0.,0.,-1.));
#31344=DIRECTION('ref_axis',(-1.,0.,0.));
#31345=DIRECTION('',(0.,1.,0.));
#31346=DIRECTION('',(-1.,0.,0.));
#31347=DIRECTION('',(0.,1.,0.));
#31348=DIRECTION('',(0.,1.,0.));
#31349=DIRECTION('',(0.,1.,0.));
#31350=DIRECTION('',(0.,1.,0.));
#31351=DIRECTION('',(0.,1.,0.));
#31352=DIRECTION('center_axis',(-0.843775417979425,0.,-0.536696416993487));
#31353=DIRECTION('ref_axis',(-0.536696416993486,0.,0.843775417979425));
#31354=DIRECTION('',(-0.536696416993487,0.,0.843775417979425));
#31355=DIRECTION('center_axis',(0.842616342713453,0.,0.53851434427711));
#31356=DIRECTION('ref_axis',(0.53851434427711,0.,-0.842616342713452));
#31357=DIRECTION('',(0.,1.,0.));
#31358=DIRECTION('',(0.53851434427711,0.,-0.842616342713452));
#31359=DIRECTION('',(0.,1.,0.));
#31360=DIRECTION('',(0.,1.,0.));
#31361=DIRECTION('',(0.,1.,0.));
#31362=DIRECTION('',(0.,1.,0.));
#31363=DIRECTION('',(0.,1.,0.));
#31364=DIRECTION('',(0.,1.,0.));
#31365=DIRECTION('',(0.,1.,0.));
#31366=DIRECTION('center_axis',(0.,0.,1.));
#31367=DIRECTION('ref_axis',(1.,0.,0.));
#31368=DIRECTION('',(1.,0.,0.));
#31369=DIRECTION('center_axis',(0.,0.,-1.));
#31370=DIRECTION('ref_axis',(-1.,0.,0.));
#31371=DIRECTION('',(0.,1.,0.));
#31372=DIRECTION('',(-1.,0.,0.));
#31373=DIRECTION('center_axis',(1.,0.,0.));
#31374=DIRECTION('ref_axis',(0.,0.,-1.));
#31375=DIRECTION('',(0.,0.,-1.));
#31376=DIRECTION('center_axis',(0.,-1.,0.));
#31377=DIRECTION('ref_axis',(0.,0.,-1.));
#31378=DIRECTION('center_axis',(0.822192198445529,0.,-0.569209969005558));
#31379=DIRECTION('ref_axis',(-0.569209969005557,0.,-0.822192198445529));
#31380=DIRECTION('',(0.,1.,0.));
#31381=DIRECTION('',(-0.569209969005557,0.,-0.822192198445529));
#31382=DIRECTION('',(0.,1.,0.));
#31383=DIRECTION('center_axis',(0.,0.,1.));
#31384=DIRECTION('ref_axis',(1.,0.,0.));
#31385=DIRECTION('',(0.,1.,0.));
#31386=DIRECTION('',(1.,0.,0.));
#31387=DIRECTION('center_axis',(-0.835018956019145,0.,0.550221176517859));
#31388=DIRECTION('ref_axis',(0.550221176517859,0.,0.835018956019145));
#31389=DIRECTION('',(0.,1.,0.));
#31390=DIRECTION('',(0.550221176517859,0.,0.835018956019145));
#31391=DIRECTION('',(0.,1.,0.));
#31392=DIRECTION('',(0.,1.,0.));
#31393=DIRECTION('center_axis',(0.836969643122507,0.,0.547249318401935));
#31394=DIRECTION('ref_axis',(0.547249318401935,0.,-0.836969643122507));
#31395=DIRECTION('',(0.,1.,0.));
#31396=DIRECTION('',(0.547249318401935,0.,-0.836969643122507));
#31397=DIRECTION('center_axis',(0.,0.,1.));
#31398=DIRECTION('ref_axis',(1.,0.,0.));
#31399=DIRECTION('',(0.,1.,0.));
#31400=DIRECTION('',(1.,0.,0.));
#31401=DIRECTION('center_axis',(-0.831292792364464,0.,-0.555834771638921));
#31402=DIRECTION('ref_axis',(-0.555834771638921,0.,0.831292792364464));
#31403=DIRECTION('',(0.,1.,0.));
#31404=DIRECTION('',(-0.555834771638921,0.,0.831292792364464));
#31405=DIRECTION('center_axis',(-1.,0.,0.));
#31406=DIRECTION('ref_axis',(0.,0.,1.));
#31407=DIRECTION('',(0.,1.,0.));
#31408=DIRECTION('',(0.,0.,1.));
#31409=DIRECTION('center_axis',(0.,0.,-1.));
#31410=DIRECTION('ref_axis',(-1.,0.,0.));
#31411=DIRECTION('',(0.,1.,0.));
#31412=DIRECTION('',(-1.,0.,0.));
#31413=DIRECTION('center_axis',(1.,0.,0.));
#31414=DIRECTION('ref_axis',(0.,0.,-1.));
#31415=DIRECTION('',(0.,0.,-1.));
#31416=DIRECTION('center_axis',(0.,-1.,0.));
#31417=DIRECTION('ref_axis',(0.,0.,-1.));
#31418=DIRECTION('center_axis',(0.,1.,0.));
#31419=DIRECTION('ref_axis',(1.,0.,0.));
#31420=DIRECTION('',(0.,1.,0.));
#31421=DIRECTION('center_axis',(0.,1.,0.));
#31422=DIRECTION('ref_axis',(1.,0.,0.));
#31423=DIRECTION('',(0.,1.,0.));
#31424=DIRECTION('center_axis',(0.,1.,0.));
#31425=DIRECTION('ref_axis',(1.,0.,0.));
#31426=DIRECTION('',(0.,1.,0.));
#31427=DIRECTION('center_axis',(0.,1.,0.));
#31428=DIRECTION('ref_axis',(1.,0.,0.));
#31429=DIRECTION('',(0.,1.,0.));
#31430=DIRECTION('center_axis',(0.,-1.,0.));
#31431=DIRECTION('ref_axis',(0.,0.,-1.));
#31432=DIRECTION('center_axis',(0.,-1.,0.));
#31433=DIRECTION('ref_axis',(-7.79103876929934E-17,0.,-1.));
#31434=DIRECTION('',(0.,-1.,0.));
#31435=DIRECTION('center_axis',(0.,1.,0.));
#31436=DIRECTION('ref_axis',(0.5,0.,0.866025403784439));
#31437=DIRECTION('',(0.,-1.,0.));
#31438=DIRECTION('center_axis',(-0.866025403784439,0.,0.499999999999999));
#31439=DIRECTION('ref_axis',(-0.499999999999999,0.,-0.866025403784439));
#31440=DIRECTION('',(-0.499999999999999,0.,-0.866025403784439));
#31441=DIRECTION('center_axis',(0.866025403784439,0.,0.5));
#31442=DIRECTION('ref_axis',(-0.5,0.,0.866025403784439));
#31443=DIRECTION('',(-0.5,0.,0.866025403784439));
#31444=DIRECTION('center_axis',(0.,1.,0.));
#31445=DIRECTION('ref_axis',(1.,0.,0.));
#31446=DIRECTION('center_axis',(9.25185853854297E-17,0.,1.));
#31447=DIRECTION('ref_axis',(-1.,0.,9.25185853854297E-17));
#38585=CARTESIAN_POINT('',(0.,0.,0.));
#38586=CARTESIAN_POINT('Ctrl Pts',(-3.57453458878627,-16.9981470538884,
-71.8682453580158));
#38587=CARTESIAN_POINT('Ctrl Pts',(-3.57038661518134,-16.9983534204838,
-71.8641633585059));
#38588=CARTESIAN_POINT('Ctrl Pts',(-3.53990786586211,-16.9997799301677,
-71.834280745957));
#38589=CARTESIAN_POINT('Ctrl Pts',(-3.50642976897921,-16.9999870327594,
-71.8016132291015));
#38590=CARTESIAN_POINT('Ctrl Pts',(-3.50104102377553,-17.,-71.7963365978802));
#38591=CARTESIAN_POINT('Ctrl Pts',(-3.50000000000001,-17.,-71.7953186364093));
#38592=CARTESIAN_POINT('Ctrl Pts',(-3.33910484519611,-16.9981470538884,
-72.1036751016059));
#38593=CARTESIAN_POINT('Ctrl Pts',(-3.33497886295621,-16.9983534204838,
-72.0995711107311));
#38594=CARTESIAN_POINT('Ctrl Pts',(-3.30473155320942,-16.9997799301677,
-72.0694570586097));
#38595=CARTESIAN_POINT('Ctrl Pts',(-3.27148136320786,-16.9999870327594,
-72.0365616348729));
#38596=CARTESIAN_POINT('Ctrl Pts',(-3.26613954847709,-17.,-72.0312380731786));
#38597=CARTESIAN_POINT('Ctrl Pts',(-3.26510621213643,-17.,-72.0302124242728));
#38598=CARTESIAN_POINT('Ctrl Pts',(-3.10367510160595,-16.9981470538884,
-72.3391048451961));
#38599=CARTESIAN_POINT('Ctrl Pts',(-3.09957111073108,-16.9983534204838,
-72.3349788629562));
#38600=CARTESIAN_POINT('Ctrl Pts',(-3.06945705860968,-17.0000242835561,
-72.3045547255514));
#38601=CARTESIAN_POINT('Ctrl Pts',(-3.03656163487292,-16.9998354184739,
-72.2714568031683));
#38602=CARTESIAN_POINT('Ctrl Pts',(-3.03123807317866,-17.,-72.2661395484771));
#38603=CARTESIAN_POINT('Ctrl Pts',(-3.03021242427286,-17.,-72.2651062121364));
#38604=CARTESIAN_POINT('Ctrl Pts',(-2.8682453580158,-16.9981470538884,-72.5745345887863));
#38605=CARTESIAN_POINT('Ctrl Pts',(-2.86416335850596,-16.9983534204838,
-72.5703866151813));
#38606=CARTESIAN_POINT('Ctrl Pts',(-2.834280745957,-16.9997799301677,-72.5399078658621));
#38607=CARTESIAN_POINT('Ctrl Pts',(-2.80161322910157,-16.9999870327594,
-72.5064297689792));
#38608=CARTESIAN_POINT('Ctrl Pts',(-2.79633659788023,-17.,-72.5010410237755));
#38609=CARTESIAN_POINT('Ctrl Pts',(-2.79531863640928,-17.,-72.5));
#38610=CARTESIAN_POINT('',(-3.50000000000001,-17.,-71.7953186364093));
#38611=CARTESIAN_POINT('',(-3.57453458878627,-16.9981470538884,-71.8682453580158));
#38612=CARTESIAN_POINT('Ctrl Pts',(-3.50000000000001,-17.,-71.7953186364093));
#38613=CARTESIAN_POINT('Ctrl Pts',(-3.50033136103369,-17.,-71.7956426566413));
#38614=CARTESIAN_POINT('Ctrl Pts',(-3.5006659910395,-16.9999999087783,-71.7959698710105));
#38615=CARTESIAN_POINT('Ctrl Pts',(-3.50107815475911,-16.9999996125274,
-71.7963728195339));
#38616=CARTESIAN_POINT('Ctrl Pts',(-3.50151072778698,-16.9999993016069,
-71.7967957210522));
#38617=CARTESIAN_POINT('Ctrl Pts',(-3.50202849537424,-16.999998768055,-71.7973018394014));
#38618=CARTESIAN_POINT('Ctrl Pts',(-3.50267576544797,-16.9999976134245,
-71.7979344421874));
#38619=CARTESIAN_POINT('Ctrl Pts',(-3.50336536547692,-16.9999963832839,
-71.7986084157221));
#38620=CARTESIAN_POINT('Ctrl Pts',(-3.50420167541479,-16.9999944448324,
-71.7994256794686));
#38621=CARTESIAN_POINT('Ctrl Pts',(-3.50519595537292,-16.9999910006556,
-71.8003972134395));
#38622=CARTESIAN_POINT('Ctrl Pts',(-3.50629355744884,-16.9999871985718,
-71.8014697058443));
#38623=CARTESIAN_POINT('Ctrl Pts',(-3.50758325228922,-16.9999815341953,
-71.8027297908791));
#38624=CARTESIAN_POINT('Ctrl Pts',(-3.50903534240292,-16.9999727872824,
-71.8041484437089));
#38625=CARTESIAN_POINT('Ctrl Pts',(-3.51085714423962,-16.9999618133477,
-71.8059282949086));
#38626=CARTESIAN_POINT('Ctrl Pts',(-3.51293366154212,-16.9999458718544,
-71.8079568545964));
#38627=CARTESIAN_POINT('Ctrl Pts',(-3.51514671247924,-16.9999235237508,
-71.8101187023244));
#38628=CARTESIAN_POINT('Ctrl Pts',(-3.51749449195537,-16.9998998151149,
-71.8124121613864));
#38629=CARTESIAN_POINT('Ctrl Pts',(-3.51999108761033,-16.9998688531822,
-71.8148508937686));
#38630=CARTESIAN_POINT('Ctrl Pts',(-3.52248486630919,-16.9998314674613,
-71.8172869062406));
#38631=CARTESIAN_POINT('Ctrl Pts',(-3.52437422457713,-16.9998031429668,
-71.8191324991581));
#38632=CARTESIAN_POINT('Ctrl Pts',(-3.52626114404881,-16.9997712320714,
-71.820975729331));
#38633=CARTESIAN_POINT('Ctrl Pts',(-3.52810370841093,-16.9997367040829,
-71.8227757579311));
#38634=CARTESIAN_POINT('Ctrl Pts',(-3.52976637007423,-16.9997055473083,
-71.8244000369021));
#38635=CARTESIAN_POINT('Ctrl Pts',(-3.53139250445814,-16.9996723091153,
-71.8259887368555));
#38636=CARTESIAN_POINT('Ctrl Pts',(-3.53298085050798,-16.9996373773349,
-71.8275407505539));
#38637=CARTESIAN_POINT('Ctrl Pts',(-3.53454774391493,-16.9996029173527,
-71.8290718023242));
#38638=CARTESIAN_POINT('Ctrl Pts',(-3.53607719242338,-16.9995668629652,
-71.8305664957214));
#38639=CARTESIAN_POINT('Ctrl Pts',(-3.53760652085725,-16.9995285090951,
-71.8320614739058));
#38640=CARTESIAN_POINT('Ctrl Pts',(-3.53909804395504,-16.9994911033411,
-71.8335194958999));
#38641=CARTESIAN_POINT('Ctrl Pts',(-3.54059613558281,-16.9994513364011,
-71.8349843334469));
#38642=CARTESIAN_POINT('Ctrl Pts',(-3.54213060631552,-16.9994082206029,
-71.8364852326097));
#38643=CARTESIAN_POINT('Ctrl Pts',(-3.54377985735808,-16.9993618796896,
-71.8380984008873));
#38644=CARTESIAN_POINT('Ctrl Pts',(-3.54547077478773,-16.9993116397098,
-71.8397528770164));
#38645=CARTESIAN_POINT('Ctrl Pts',(-3.54719744053076,-16.9992572833264,
-71.8414428847978));
#38646=CARTESIAN_POINT('Ctrl Pts',(-3.54917002631363,-16.9991951852455,
-71.8433735916159));
#38647=CARTESIAN_POINT('Ctrl Pts',(-3.5511887316105,-16.9991276636875,-71.8453501484939));
#38648=CARTESIAN_POINT('Ctrl Pts',(-3.55319701397691,-16.9990563957717,
-71.8473171286809));
#38649=CARTESIAN_POINT('Ctrl Pts',(-3.55597939118123,-16.9989576575524,
-71.8500422837315));
#38650=CARTESIAN_POINT('Ctrl Pts',(-3.55873880452009,-16.9988515979041,
-71.852746171332));
#38651=CARTESIAN_POINT('Ctrl Pts',(-3.56125854441703,-16.9987486082515,
-71.8552161386878));
#38652=CARTESIAN_POINT('Ctrl Pts',(-3.56314834933973,-16.9986713660121,
-71.8570686142047));
#38653=CARTESIAN_POINT('Ctrl Pts',(-3.56490064570704,-16.998596102758,-71.8587868623067));
#38654=CARTESIAN_POINT('Ctrl Pts',(-3.56643959313734,-16.9985278711001,
-71.8602963585416));
#38655=CARTESIAN_POINT('Ctrl Pts',(-3.5677289530966,-16.9984707052957,-71.861561043719));
#38656=CARTESIAN_POINT('Ctrl Pts',(-3.56886818435408,-16.9984185388897,
-71.8626788313976));
#38657=CARTESIAN_POINT('Ctrl Pts',(-3.569838986615,-16.998373289921,-71.8636316653217));
#38658=CARTESIAN_POINT('Ctrl Pts',(-3.5707517147712,-16.9983307477788,-71.8645275000202));
#38659=CARTESIAN_POINT('Ctrl Pts',(-3.57151514502306,-16.9982943574932,
-71.8652771155595));
#38660=CARTESIAN_POINT('Ctrl Pts',(-3.57214502087146,-16.9982640274543,
-71.8658958651527));
#38661=CARTESIAN_POINT('Ctrl Pts',(-3.57273209133855,-16.9982357585976,
-71.8664725654875));
#38662=CARTESIAN_POINT('Ctrl Pts',(-3.57320299278079,-16.9982127623775,
-71.8669354348749));
#38663=CARTESIAN_POINT('Ctrl Pts',(-3.57360188999631,-16.9981931657129,
-71.867327729259));
#38664=CARTESIAN_POINT('Ctrl Pts',(-3.57394979081279,-16.9981760743537,
-71.8676698713729));
#38665=CARTESIAN_POINT('Ctrl Pts',(-3.57424318974085,-16.9981615513357,
-71.8679585937126));
#38666=CARTESIAN_POINT('Ctrl Pts',(-3.57453458878627,-16.9981470538884,
-71.8682453580158));
#38667=CARTESIAN_POINT('',(-2.8682453580158,-16.9981470538884,-72.5745345887863));
#38668=CARTESIAN_POINT('Ctrl Pts',(-2.8682453580158,-16.9981470538884,-72.5745345887863));
#38669=CARTESIAN_POINT('Ctrl Pts',(-3.10367510160595,-16.9981470538884,
-72.3391048451961));
#38670=CARTESIAN_POINT('Ctrl Pts',(-3.33910484519611,-16.9981470538884,
-72.1036751016059));
#38671=CARTESIAN_POINT('Ctrl Pts',(-3.57453458878627,-16.9981470538884,
-71.8682453580158));
#38672=CARTESIAN_POINT('',(-2.79531863640928,-17.,-72.5));
#38673=CARTESIAN_POINT('Ctrl Pts',(-2.8682453580158,-16.9981470538884,-72.5745345887863));
#38674=CARTESIAN_POINT('Ctrl Pts',(-2.86792051198432,-16.9981634765679,
-72.5742044925281));
#38675=CARTESIAN_POINT('Ctrl Pts',(-2.86759246756108,-16.9981799708645,
-72.5738711310018));
#38676=CARTESIAN_POINT('Ctrl Pts',(-2.86718860352499,-16.9982001093812,
-72.57346041281));
#38677=CARTESIAN_POINT('Ctrl Pts',(-2.8667647393911,-16.9982212451946,-72.57302935509));
#38678=CARTESIAN_POINT('Ctrl Pts',(-2.86625756382415,-16.9982463879926,
-72.5725132968389));
#38679=CARTESIAN_POINT('Ctrl Pts',(-2.86562376912052,-16.9982773404549,
-72.5718680115171));
#38680=CARTESIAN_POINT('Ctrl Pts',(-2.86494852089772,-16.9983103173716,
-72.5711805211291));
#38681=CARTESIAN_POINT('Ctrl Pts',(-2.86412982782488,-16.9983498713227,
-72.5703466306137));
#38682=CARTESIAN_POINT('Ctrl Pts',(-2.86315671761944,-16.9983957676602,
-72.5693550535868));
#38683=CARTESIAN_POINT('Ctrl Pts',(-2.86208246075231,-16.9984464345378,
-72.5682604104266));
#38684=CARTESIAN_POINT('Ctrl Pts',(-2.86082042406595,-16.9985047829815,
-72.5669740091159));
#38685=CARTESIAN_POINT('Ctrl Pts',(-2.85939970674286,-16.9985681244217,
-72.565525387959));
#38686=CARTESIAN_POINT('Ctrl Pts',(-2.85761705827721,-16.9986476022457,
-72.5637077270911));
#38687=CARTESIAN_POINT('Ctrl Pts',(-2.85558546640714,-16.9987347812318,
-72.5616355608823));
#38688=CARTESIAN_POINT('Ctrl Pts',(-2.85342062894715,-16.9988223610841,
-72.5594266767905));
#38689=CARTESIAN_POINT('Ctrl Pts',(-2.85112488425853,-16.9989152368701,
-72.5570842219803));
#38690=CARTESIAN_POINT('Ctrl Pts',(-2.84868403352369,-16.9990082804756,
-72.5545928471897));
#38691=CARTESIAN_POINT('Ctrl Pts',(-2.84624625175194,-16.9990947989236,
-72.552103587594));
#38692=CARTESIAN_POINT('Ctrl Pts',(-2.84439897927723,-16.9991603598156,
-72.5502173068831));
#38693=CARTESIAN_POINT('Ctrl Pts',(-2.84255427195847,-16.9992222334679,
-72.5483330647398));
#38694=CARTESIAN_POINT('Ctrl Pts',(-2.84075306394265,-16.9992793054386,
-72.5464926261216));
#38695=CARTESIAN_POINT('Ctrl Pts',(-2.83912769582927,-16.9993308058541,
-72.5448318572274));
#38696=CARTESIAN_POINT('Ctrl Pts',(-2.83753815081148,-16.9993784253393,
-72.543207168852));
#38697=CARTESIAN_POINT('Ctrl Pts',(-2.83598557864455,-16.9994224873957,
-72.5416197584348));
#38698=CARTESIAN_POINT('Ctrl Pts',(-2.83445351746977,-16.9994659673493,
-72.540053319257));
#38699=CARTESIAN_POINT('Ctrl Pts',(-2.83295811821705,-16.9995060035546,
-72.5385238533706));
#38700=CARTESIAN_POINT('Ctrl Pts',(-2.83146270058428,-16.9995437460623,
-72.5369939676884));
#38701=CARTESIAN_POINT('Ctrl Pts',(-2.83000471420189,-16.9995805438512,
-72.5355023760136));
#38702=CARTESIAN_POINT('Ctrl Pts',(-2.82854016663104,-16.9996153196962,
-72.5340037037557));
#38703=CARTESIAN_POINT('Ctrl Pts',(-2.82703981578638,-16.9996485645807,
-72.5324681805947));
#38704=CARTESIAN_POINT('Ctrl Pts',(-2.82542721104073,-16.9996842967954,
-72.5308177719951));
#38705=CARTESIAN_POINT('Ctrl Pts',(-2.82377359513262,-16.9997182120423,
-72.529125149268));
#38706=CARTESIAN_POINT('Ctrl Pts',(-2.82208470500296,-16.9997497930326,
-72.5273963190708));
#38707=CARTESIAN_POINT('Ctrl Pts',(-2.82015515581749,-16.9997858741684,
-72.5254211385423));
#38708=CARTESIAN_POINT('Ctrl Pts',(-2.81818008615893,-16.9998188305302,
-72.5233992312896));
#38709=CARTESIAN_POINT('Ctrl Pts',(-2.81621482751817,-16.9998475191546,
-72.52138736276));
#38710=CARTESIAN_POINT('Ctrl Pts',(-2.81349256857323,-16.9998872583841,
-72.5186005402078));
#38711=CARTESIAN_POINT('Ctrl Pts',(-2.81079201806523,-16.9999185308537,
-72.5158359360068));
#38712=CARTESIAN_POINT('Ctrl Pts',(-2.80832539114039,-16.9999409383933,
-72.5133109478137));
#38713=CARTESIAN_POINT('Ctrl Pts',(-2.80647542094676,-16.9999577440481,
-72.5114172066689));
#38714=CARTESIAN_POINT('Ctrl Pts',(-2.80475967567115,-16.9999696816405,
-72.5096609508553));
#38715=CARTESIAN_POINT('Ctrl Pts',(-2.803252515256,-16.9999780308564,-72.508118309431));
#38716=CARTESIAN_POINT('Ctrl Pts',(-2.80198975715483,-16.999985026157,-72.5068258239488));
#38717=CARTESIAN_POINT('Ctrl Pts',(-2.80087378577512,-16.9999895478102,
-72.5056836631397));
#38718=CARTESIAN_POINT('Ctrl Pts',(-2.79992260032024,-16.9999926045357,
-72.5047102375997));
#38719=CARTESIAN_POINT('Ctrl Pts',(-2.7990283037671,-16.9999954784432,-72.5037950311059));
#38720=CARTESIAN_POINT('Ctrl Pts',(-2.79828008131995,-16.9999970739683,
-72.5030293988184));
#38721=CARTESIAN_POINT('Ctrl Pts',(-2.797662574869,-16.9999980838367,-72.5023976001144));
#38722=CARTESIAN_POINT('Ctrl Pts',(-2.79708702610117,-16.9999990250876,
-72.5018087302087));
#38723=CARTESIAN_POINT('Ctrl Pts',(-2.79662518068282,-16.9999994582021,
-72.5013362750362));
#38724=CARTESIAN_POINT('Ctrl Pts',(-2.79623381941523,-16.9999997079814,
-72.500935978419));
#38725=CARTESIAN_POINT('Ctrl Pts',(-2.79589255313754,-16.9999999257886,
-72.5005869205336));
#38726=CARTESIAN_POINT('Ctrl Pts',(-2.79560461778333,-17.,-72.5002924603909));
#38727=CARTESIAN_POINT('Ctrl Pts',(-2.79531863640928,-17.,-72.5));
#38728=CARTESIAN_POINT('',(-3.14765931820465,-17.,-72.1476593182046));
#38729=CARTESIAN_POINT('Ctrl Pts',(-2.8682453580158,-16.9981470538884,-72.5745345887863));
#38730=CARTESIAN_POINT('Ctrl Pts',(-3.24643975969904,-16.9790273330526,
-72.9588414442702));
#38731=CARTESIAN_POINT('Ctrl Pts',(-3.89283858086127,-16.6911512202391,
-73.5507380181503));
#38732=CARTESIAN_POINT('Ctrl Pts',(-4.4212646197358,-16.0144112572066,-73.9509340499422));
#38733=CARTESIAN_POINT('Ctrl Pts',(-4.50000000000001,-15.6672482052684,
-74.));
#38734=CARTESIAN_POINT('Ctrl Pts',(-4.50000000000001,-15.5,-74.));
#38735=CARTESIAN_POINT('Ctrl Pts',(-3.10367510160595,-16.9981470538884,
-72.3391048451961));
#38736=CARTESIAN_POINT('Ctrl Pts',(-3.48390698788944,-16.9790273330526,
-72.7213742160798));
#38737=CARTESIAN_POINT('Ctrl Pts',(-4.11213839329096,-16.6911512202391,
-73.3314382057206));
#38738=CARTESIAN_POINT('Ctrl Pts',(-4.59782109647127,-16.0144112572066,
-73.7743775732067));
#38739=CARTESIAN_POINT('Ctrl Pts',(-4.66666666666668,-15.6672482052684,
-73.8333333333333));
#38740=CARTESIAN_POINT('Ctrl Pts',(-4.66666666666668,-15.5,-73.8333333333333));
#38741=CARTESIAN_POINT('Ctrl Pts',(-3.33910484519611,-16.9981470538884,
-72.1036751016059));
#38742=CARTESIAN_POINT('Ctrl Pts',(-3.72137421607984,-16.9790273330526,
-72.4839069878894));
#38743=CARTESIAN_POINT('Ctrl Pts',(-4.33143820572064,-16.6911512202391,
-73.112138393291));
#38744=CARTESIAN_POINT('Ctrl Pts',(-4.77437757320675,-16.0144112572066,
-73.5978210964713));
#38745=CARTESIAN_POINT('Ctrl Pts',(-4.83333333333335,-15.6672482052684,
-73.6666666666667));
#38746=CARTESIAN_POINT('Ctrl Pts',(-4.83333333333335,-15.5,-73.6666666666667));
#38747=CARTESIAN_POINT('Ctrl Pts',(-3.57453458878627,-16.9981470538884,
-71.8682453580158));
#38748=CARTESIAN_POINT('Ctrl Pts',(-3.95884144427025,-16.9790273330526,
-72.246439759699));
#38749=CARTESIAN_POINT('Ctrl Pts',(-4.55073801815033,-16.6911512202391,
-72.8928385808613));
#38750=CARTESIAN_POINT('Ctrl Pts',(-4.95093404994221,-16.0144112572066,
-73.4212646197358));
#38751=CARTESIAN_POINT('Ctrl Pts',(-5.00000000000001,-15.6672482052684,
-73.5));
#38752=CARTESIAN_POINT('Ctrl Pts',(-5.00000000000001,-15.5,-73.5));
#38753=CARTESIAN_POINT('',(-5.00000000000001,-15.5,-73.5));
#38754=CARTESIAN_POINT('Ctrl Pts',(-3.57453458878627,-16.9981470538884,
-71.8682453580158));
#38755=CARTESIAN_POINT('Ctrl Pts',(-3.95884144427025,-16.9790273330526,
-72.246439759699));
#38756=CARTESIAN_POINT('Ctrl Pts',(-4.55073801815033,-16.6911512202391,
-72.8928385808613));
#38757=CARTESIAN_POINT('Ctrl Pts',(-4.95093404994221,-16.0144112572066,
-73.4212646197358));
#38758=CARTESIAN_POINT('Ctrl Pts',(-5.00000000000001,-15.6672482052684,
-73.5));
#38759=CARTESIAN_POINT('Ctrl Pts',(-5.00000000000001,-15.5,-73.5));
#38760=CARTESIAN_POINT('',(-4.50000000000001,-15.5,-74.));
#38761=CARTESIAN_POINT('',(-5.00000000000001,-15.5,-73.5));
#38762=CARTESIAN_POINT('Ctrl Pts',(-4.50000000000001,-15.5,-74.));
#38763=CARTESIAN_POINT('Ctrl Pts',(-4.50000000000001,-15.6672482052684,
-74.));
#38764=CARTESIAN_POINT('Ctrl Pts',(-4.4212646197358,-16.0144112572066,-73.9509340499422));
#38765=CARTESIAN_POINT('Ctrl Pts',(-3.89283858086127,-16.6911512202391,
-73.5507380181503));
#38766=CARTESIAN_POINT('Ctrl Pts',(-3.24643975969904,-16.9790273330526,
-72.9588414442702));
#38767=CARTESIAN_POINT('Ctrl Pts',(-2.8682453580158,-16.9981470538884,-72.5745345887863));
#38768=CARTESIAN_POINT('Origin',(-4.75000000000001,-14.,-73.75));
#38769=CARTESIAN_POINT('',(-5.00000000000001,-14.,-73.5));
#38770=CARTESIAN_POINT('',(-4.50000000000001,-14.,-74.));
#38771=CARTESIAN_POINT('',(-44.75,-14.,-33.7500000000002));
#38772=CARTESIAN_POINT('',(-4.50000000000001,-14.,-74.));
#38773=CARTESIAN_POINT('',(-5.00000000000001,-14.,-73.5));
#38774=CARTESIAN_POINT('Origin',(-1.11022302462516E-14,-17.,-62.));
#38775=CARTESIAN_POINT('',(2.79531863640925,-17.,-72.5));
#38776=CARTESIAN_POINT('',(-2.50000000000001,-17.,-72.5));
#38777=CARTESIAN_POINT('',(3.49999999999999,-17.,-71.7953186364093));
#38778=CARTESIAN_POINT('',(3.14765931820462,-17.,-72.1476593182046));
#38779=CARTESIAN_POINT('',(3.49999999999999,-17.,-56.3914887194867));
#38780=CARTESIAN_POINT('',(3.49999999999999,-17.,-68.));
#38781=CARTESIAN_POINT('',(-6.91925441518255E-15,-17.,-56.5));
#38782=CARTESIAN_POINT('Origin',(0.,-17.,0.));
#38783=CARTESIAN_POINT('',(-3.50000000000001,-17.,-56.3914887194867));
#38784=CARTESIAN_POINT('Origin',(0.,-17.,0.));
#38785=CARTESIAN_POINT('',(-3.50000000000001,-17.,-56.));
#38786=CARTESIAN_POINT('Origin',(-2.50000000000001,-15.5,-72.5));
#38787=CARTESIAN_POINT('',(4.49999999999999,-15.5,-74.));
#38788=CARTESIAN_POINT('',(-2.50000000000001,-15.5,-74.));
#38789=CARTESIAN_POINT('',(2.86824535801577,-16.9981470538884,-72.5745345887863));
#38790=CARTESIAN_POINT('Ctrl Pts',(2.86824535801577,-16.9981470538884,-72.5745345887863));
#38791=CARTESIAN_POINT('Ctrl Pts',(3.12037495913793,-16.9854005733312,-72.8307391591089));
#38792=CARTESIAN_POINT('Ctrl Pts',(3.63377877163942,-16.8268077199093,-73.3201733549766));
#38793=CARTESIAN_POINT('Ctrl Pts',(4.13541628736353,-16.3991227020429,-73.7358067305414));
#38794=CARTESIAN_POINT('Ctrl Pts',(4.43902863521563,-15.9274342791999,-73.9615602058987));
#38795=CARTESIAN_POINT('Ctrl Pts',(4.49999999999999,-15.6672482052684,-74.));
#38796=CARTESIAN_POINT('Ctrl Pts',(4.49999999999999,-15.5,-74.));
#38797=CARTESIAN_POINT('Ctrl Pts',(2.79531863640925,-17.,-72.5));
#38798=CARTESIAN_POINT('Ctrl Pts',(2.79564265664125,-17.,-72.5003313610337));
#38799=CARTESIAN_POINT('Ctrl Pts',(2.79596987101048,-16.9999999087783,-72.5006659910395));
#38800=CARTESIAN_POINT('Ctrl Pts',(2.79637281953385,-16.9999996125274,-72.5010781547591));
#38801=CARTESIAN_POINT('Ctrl Pts',(2.79679572105219,-16.9999993016069,-72.501510727787));
#38802=CARTESIAN_POINT('Ctrl Pts',(2.79730183940143,-16.999998768055,-72.5020284953742));
#38803=CARTESIAN_POINT('Ctrl Pts',(2.79793444218738,-16.9999976134245,-72.502675765448));
#38804=CARTESIAN_POINT('Ctrl Pts',(2.79860841572207,-16.9999963832839,-72.5033653654769));
#38805=CARTESIAN_POINT('Ctrl Pts',(2.79942567946863,-16.9999944448324,-72.5042016754148));
#38806=CARTESIAN_POINT('Ctrl Pts',(2.80039721343958,-16.9999910006556,-72.505195955373));
#38807=CARTESIAN_POINT('Ctrl Pts',(2.80146970584441,-16.9999871985718,-72.5062935574489));
#38808=CARTESIAN_POINT('Ctrl Pts',(2.80272979087922,-16.9999815341953,-72.5075832522893));
#38809=CARTESIAN_POINT('Ctrl Pts',(2.80414844370906,-16.9999727872824,-72.5090353424031));
#38810=CARTESIAN_POINT('Ctrl Pts',(2.80592829490883,-16.9999618133477,-72.5108571442398));
#38811=CARTESIAN_POINT('Ctrl Pts',(2.80795685459665,-16.9999458718544,-72.5129336615423));
#38812=CARTESIAN_POINT('Ctrl Pts',(2.81011870232471,-16.9999235237508,-72.5151467124795));
#38813=CARTESIAN_POINT('Ctrl Pts',(2.81241216138656,-16.9998998151149,-72.5174944919555));
#38814=CARTESIAN_POINT('Ctrl Pts',(2.81485089376864,-16.9998688531822,-72.5199910876103));
#38815=CARTESIAN_POINT('Ctrl Pts',(2.81728690624043,-16.9998314674613,-72.522484866309));
#38816=CARTESIAN_POINT('Ctrl Pts',(2.81913249915803,-16.9998031429668,-72.524374224577));
#38817=CARTESIAN_POINT('Ctrl Pts',(2.82097572933092,-16.9997712320714,-72.5262611440487));
#38818=CARTESIAN_POINT('Ctrl Pts',(2.82277575793103,-16.9997367040829,-72.5281037084108));
#38819=CARTESIAN_POINT('Ctrl Pts',(2.82440003690208,-16.9997055473083,-72.5297663700741));
#38820=CARTESIAN_POINT('Ctrl Pts',(2.82598873685543,-16.9996723091153,-72.531392504458));
#38821=CARTESIAN_POINT('Ctrl Pts',(2.82754075055383,-16.9996373773349,-72.5329808505079));
#38822=CARTESIAN_POINT('Ctrl Pts',(2.82907180232415,-16.9996029173527,-72.5345477439148));
#38823=CARTESIAN_POINT('Ctrl Pts',(2.83056649572128,-16.9995668629652,-72.5360771924232));
#38824=CARTESIAN_POINT('Ctrl Pts',(2.83206147390567,-16.9995285090951,-72.5376065208571));
#38825=CARTESIAN_POINT('Ctrl Pts',(2.83351949589972,-16.9994911033411,-72.5390980439549));
#38826=CARTESIAN_POINT('Ctrl Pts',(2.83498433344674,-16.9994513364011,-72.5405961355826));
#38827=CARTESIAN_POINT('Ctrl Pts',(2.83648523260946,-16.9994082206029,-72.5421306063153));
#38828=CARTESIAN_POINT('Ctrl Pts',(2.83809840088706,-16.9993618796896,-72.5437798573578));
#38829=CARTESIAN_POINT('Ctrl Pts',(2.83975287701612,-16.9993116397098,-72.5454707747875));
#38830=CARTESIAN_POINT('Ctrl Pts',(2.84144288479756,-16.9992572833264,-72.5471974405305));
#38831=CARTESIAN_POINT('Ctrl Pts',(2.84337359161558,-16.9991951852455,-72.5491700263133));
#38832=CARTESIAN_POINT('Ctrl Pts',(2.84535014849349,-16.9991276636876,-72.5511887316101));
#38833=CARTESIAN_POINT('Ctrl Pts',(2.84731712868045,-16.9990563957717,-72.5531970139764));
#38834=CARTESIAN_POINT('Ctrl Pts',(2.85004228373103,-16.9989576575525,-72.5559793911808));
#38835=CARTESIAN_POINT('Ctrl Pts',(2.85274617133159,-16.9988515979041,-72.5587388045197));
#38836=CARTESIAN_POINT('Ctrl Pts',(2.8552161386875,-16.9987486082515,-72.5612585444167));
#38837=CARTESIAN_POINT('Ctrl Pts',(2.85706861420443,-16.9986713660121,-72.5631483493394));
#38838=CARTESIAN_POINT('Ctrl Pts',(2.85878686230641,-16.998596102758,-72.5649006457068));
#38839=CARTESIAN_POINT('Ctrl Pts',(2.86029635854136,-16.9985278711001,-72.5664395931371));
#38840=CARTESIAN_POINT('Ctrl Pts',(2.86156104371881,-16.9984707052957,-72.5677289530964));
#38841=CARTESIAN_POINT('Ctrl Pts',(2.8626788313974,-16.9984185388897,-72.5688681843539));
#38842=CARTESIAN_POINT('Ctrl Pts',(2.86363166532155,-16.998373289921,-72.5698389866148));
#38843=CARTESIAN_POINT('Ctrl Pts',(2.8645275000201,-16.9983307477788,-72.5707517147711));
#38844=CARTESIAN_POINT('Ctrl Pts',(2.86527711555933,-16.9982943574932,-72.5715151450229));
#38845=CARTESIAN_POINT('Ctrl Pts',(2.86589586515254,-16.9982640274543,-72.5721450208714));
#38846=CARTESIAN_POINT('Ctrl Pts',(2.8664725654874,-16.9982357585976,-72.5727320913385));
#38847=CARTESIAN_POINT('Ctrl Pts',(2.86693543487485,-16.9982127623775,-72.5732029927807));
#38848=CARTESIAN_POINT('Ctrl Pts',(2.86732772925896,-16.9981931657129,-72.5736018899962));
#38849=CARTESIAN_POINT('Ctrl Pts',(2.86766987137285,-16.9981760743537,-72.5739497908127));
#38850=CARTESIAN_POINT('Ctrl Pts',(2.86795859371254,-16.9981615513357,-72.5742431897408));
#38851=CARTESIAN_POINT('Ctrl Pts',(2.86824535801577,-16.9981470538884,-72.5745345887863));
#38852=CARTESIAN_POINT('Origin',(-5.00000000000001,-14.,-74.));
#38853=CARTESIAN_POINT('',(4.49999999999999,-14.,-74.));
#38854=CARTESIAN_POINT('',(-2.50000000000001,-14.,-74.));
#38855=CARTESIAN_POINT('',(4.49999999999999,-14.,-74.));
#38856=CARTESIAN_POINT('Ctrl Pts',(2.86824535801577,-16.9981470538884,-72.5745345887863));
#38857=CARTESIAN_POINT('Ctrl Pts',(2.86416335850593,-16.9983534204838,-72.5703866151813));
#38858=CARTESIAN_POINT('Ctrl Pts',(2.83428074595699,-16.9997799301677,-72.5399078658621));
#38859=CARTESIAN_POINT('Ctrl Pts',(2.80161322910155,-16.9999870327594,-72.5064297689792));
#38860=CARTESIAN_POINT('Ctrl Pts',(2.79633659788021,-17.,-72.5010410237755));
#38861=CARTESIAN_POINT('Ctrl Pts',(2.79531863640925,-17.,-72.5));
#38862=CARTESIAN_POINT('Ctrl Pts',(3.10367510160593,-16.9981470538884,-72.3391048451961));
#38863=CARTESIAN_POINT('Ctrl Pts',(3.09957111073106,-16.9983534204838,-72.3349788629562));
#38864=CARTESIAN_POINT('Ctrl Pts',(3.06945705860967,-16.9997799301677,-72.3047315532094));
#38865=CARTESIAN_POINT('Ctrl Pts',(3.0365616348729,-16.9999870327594,-72.2714813632078));
#38866=CARTESIAN_POINT('Ctrl Pts',(3.03123807317864,-17.,-72.2661395484771));
#38867=CARTESIAN_POINT('Ctrl Pts',(3.03021242427283,-17.,-72.2651062121364));
#38868=CARTESIAN_POINT('Ctrl Pts',(3.33910484519608,-16.9981470538884,-72.1036751016059));
#38869=CARTESIAN_POINT('Ctrl Pts',(3.33497886295619,-16.9983534204838,-72.0995711107311));
#38870=CARTESIAN_POINT('Ctrl Pts',(3.30455472555143,-17.0000242835561,-72.0694570586097));
#38871=CARTESIAN_POINT('Ctrl Pts',(3.27145680316826,-16.9998354184739,-72.0365616348729));
#38872=CARTESIAN_POINT('Ctrl Pts',(3.26613954847707,-17.,-72.0312380731786));
#38873=CARTESIAN_POINT('Ctrl Pts',(3.26510621213641,-17.,-72.0302124242728));
#38874=CARTESIAN_POINT('Ctrl Pts',(3.57453458878624,-16.9981470538884,-71.8682453580158));
#38875=CARTESIAN_POINT('Ctrl Pts',(3.57038661518131,-16.9983534204838,-71.8641633585059));
#38876=CARTESIAN_POINT('Ctrl Pts',(3.53990786586207,-16.9997799301677,-71.834280745957));
#38877=CARTESIAN_POINT('Ctrl Pts',(3.50642976897918,-16.9999870327594,-71.8016132291015));
#38878=CARTESIAN_POINT('Ctrl Pts',(3.5010410237755,-17.,-71.7963365978802));
#38879=CARTESIAN_POINT('Ctrl Pts',(3.49999999999999,-17.,-71.7953186364093));
#38880=CARTESIAN_POINT('',(3.57453458878624,-16.9981470538884,-71.8682453580158));
#38881=CARTESIAN_POINT('Ctrl Pts',(3.57453458878624,-16.9981470538884,-71.8682453580158));
#38882=CARTESIAN_POINT('Ctrl Pts',(3.33910484519608,-16.9981470538884,-72.1036751016059));
#38883=CARTESIAN_POINT('Ctrl Pts',(3.10367510160593,-16.9981470538884,-72.3391048451961));
#38884=CARTESIAN_POINT('Ctrl Pts',(2.86824535801577,-16.9981470538884,-72.5745345887863));
#38885=CARTESIAN_POINT('Ctrl Pts',(3.57453458878624,-16.9981470538884,-71.8682453580158));
#38886=CARTESIAN_POINT('Ctrl Pts',(3.57420449252802,-16.9981634765679,-71.8679205119843));
#38887=CARTESIAN_POINT('Ctrl Pts',(3.57387113100173,-16.9981799708645,-71.8675924675611));
#38888=CARTESIAN_POINT('Ctrl Pts',(3.57346041281003,-16.9982001093812,-71.867188603525));
#38889=CARTESIAN_POINT('Ctrl Pts',(3.57302935508999,-16.9982212451946,-71.8667647393911));
#38890=CARTESIAN_POINT('Ctrl Pts',(3.57251329683893,-16.9982463879926,-71.8662575638241));
#38891=CARTESIAN_POINT('Ctrl Pts',(3.57186801151713,-16.9982773404549,-71.8656237691205));
#38892=CARTESIAN_POINT('Ctrl Pts',(3.57118052112906,-16.9983103173716,-71.8649485208977));
#38893=CARTESIAN_POINT('Ctrl Pts',(3.57034663061369,-16.9983498713227,-71.8641298278249));
#38894=CARTESIAN_POINT('Ctrl Pts',(3.56935505358675,-16.9983957676602,-71.8631567176194));
#38895=CARTESIAN_POINT('Ctrl Pts',(3.56826041042658,-16.9984464345378,-71.8620824607523));
#38896=CARTESIAN_POINT('Ctrl Pts',(3.56697400911584,-16.9985047829815,-71.8608204240659));
#38897=CARTESIAN_POINT('Ctrl Pts',(3.56552538795898,-16.9985681244217,-71.8593997067428));
#38898=CARTESIAN_POINT('Ctrl Pts',(3.56370772709103,-16.9986476022457,-71.8576170582772));
#38899=CARTESIAN_POINT('Ctrl Pts',(3.56163556088222,-16.9987347812318,-71.8555854664071));
#38900=CARTESIAN_POINT('Ctrl Pts',(3.55942667679046,-16.9988223610841,-71.8534206289471));
#38901=CARTESIAN_POINT('Ctrl Pts',(3.55708422198031,-16.9989152368701,-71.8511248842585));
#38902=CARTESIAN_POINT('Ctrl Pts',(3.5545928471897,-16.9990082804756,-71.8486840335237));
#38903=CARTESIAN_POINT('Ctrl Pts',(3.55210358759401,-16.9990947989236,-71.8462462517519));
#38904=CARTESIAN_POINT('Ctrl Pts',(3.55021730688307,-16.9991603598156,-71.8443989792772));
#38905=CARTESIAN_POINT('Ctrl Pts',(3.5483330647398,-16.9992222334679,-71.8425542719585));
#38906=CARTESIAN_POINT('Ctrl Pts',(3.54649262612161,-16.9992793054386,-71.8407530639426));
#38907=CARTESIAN_POINT('Ctrl Pts',(3.54483185722742,-16.9993308058541,-71.8391276958293));
#38908=CARTESIAN_POINT('Ctrl Pts',(3.54320716885198,-16.9993784253393,-71.8375381508115));
#38909=CARTESIAN_POINT('Ctrl Pts',(3.54161975843479,-16.9994224873957,-71.8359855786445));
#38910=CARTESIAN_POINT('Ctrl Pts',(3.54005331925701,-16.9994659673493,-71.8344535174698));
#38911=CARTESIAN_POINT('Ctrl Pts',(3.53852385337056,-16.9995060035546,-71.832958118217));
#38912=CARTESIAN_POINT('Ctrl Pts',(3.53699396768836,-16.9995437460623,-71.8314627005843));
#38913=CARTESIAN_POINT('Ctrl Pts',(3.53550237601364,-16.9995805438512,-71.8300047142019));
#38914=CARTESIAN_POINT('Ctrl Pts',(3.53400370375569,-16.9996153196962,-71.828540166631));
#38915=CARTESIAN_POINT('Ctrl Pts',(3.53246818059468,-16.9996485645807,-71.8270398157864));
#38916=CARTESIAN_POINT('Ctrl Pts',(3.53081777199505,-16.9996842967954,-71.8254272110407));
#38917=CARTESIAN_POINT('Ctrl Pts',(3.52912514926799,-16.9997182120423,-71.8237735951326));
#38918=CARTESIAN_POINT('Ctrl Pts',(3.5273963190708,-16.9997497930326,-71.822084705003));
#38919=CARTESIAN_POINT('Ctrl Pts',(3.52542113854233,-16.9997858741684,-71.8201551558175));
#38920=CARTESIAN_POINT('Ctrl Pts',(3.52339923128957,-16.9998188305302,-71.8181800861589));
#38921=CARTESIAN_POINT('Ctrl Pts',(3.52138736275993,-16.9998475191546,-71.8162148275182));
#38922=CARTESIAN_POINT('Ctrl Pts',(3.51860054020781,-16.9998872583841,-71.8134925685732));
#38923=CARTESIAN_POINT('Ctrl Pts',(3.51583593600675,-16.9999185308537,-71.8107920180652));
#38924=CARTESIAN_POINT('Ctrl Pts',(3.51331094781367,-16.9999409383933,-71.8083253911404));
#38925=CARTESIAN_POINT('Ctrl Pts',(3.51141720666886,-16.9999577440481,-71.8064754209467));
#38926=CARTESIAN_POINT('Ctrl Pts',(3.50966095085529,-16.9999696816405,-71.8047596756711));
#38927=CARTESIAN_POINT('Ctrl Pts',(3.50811830943094,-16.9999780308564,-71.803252515256));
#38928=CARTESIAN_POINT('Ctrl Pts',(3.50682582394882,-16.999985026157,-71.8019897571548));
#38929=CARTESIAN_POINT('Ctrl Pts',(3.50568366313965,-16.9999895478102,-71.8008737857751));
#38930=CARTESIAN_POINT('Ctrl Pts',(3.5047102375997,-16.9999926045357,-71.7999226003202));
#38931=CARTESIAN_POINT('Ctrl Pts',(3.50379503110591,-16.9999954784432,-71.7990283037671));
#38932=CARTESIAN_POINT('Ctrl Pts',(3.50302939881839,-16.9999970739683,-71.7982800813199));
#38933=CARTESIAN_POINT('Ctrl Pts',(3.50239760011444,-16.9999980838367,-71.797662574869));
#38934=CARTESIAN_POINT('Ctrl Pts',(3.50180873020868,-16.9999990250876,-71.7970870261012));
#38935=CARTESIAN_POINT('Ctrl Pts',(3.50133627503613,-16.9999994582021,-71.7966251806828));
#38936=CARTESIAN_POINT('Ctrl Pts',(3.50093597841901,-16.9999997079814,-71.7962338194152));
#38937=CARTESIAN_POINT('Ctrl Pts',(3.50058692053359,-16.9999999257886,-71.7958925531375));
#38938=CARTESIAN_POINT('Ctrl Pts',(3.50029246039091,-17.,-71.7956046177833));
#38939=CARTESIAN_POINT('Ctrl Pts',(3.49999999999999,-17.,-71.7953186364093));
#38940=CARTESIAN_POINT('Ctrl Pts',(3.57453458878624,-16.9981470538884,-71.8682453580158));
#38941=CARTESIAN_POINT('Ctrl Pts',(3.83073915910889,-16.9854005733312,-72.1203749591379));
#38942=CARTESIAN_POINT('Ctrl Pts',(4.32017335497657,-16.8268077199093,-72.6337787716394));
#38943=CARTESIAN_POINT('Ctrl Pts',(4.7358067305414,-16.3991227020429,-73.1354162873635));
#38944=CARTESIAN_POINT('Ctrl Pts',(4.96156020589869,-15.9274342791999,-73.4390286352156));
#38945=CARTESIAN_POINT('Ctrl Pts',(4.99999999999999,-15.6672482052684,-73.5));
#38946=CARTESIAN_POINT('Ctrl Pts',(4.99999999999999,-15.5,-73.5));
#38947=CARTESIAN_POINT('Ctrl Pts',(3.33910484519608,-16.9981470538884,-72.1036751016059));
#38948=CARTESIAN_POINT('Ctrl Pts',(3.59395109245191,-16.9854005733312,-72.3571630257949));
#38949=CARTESIAN_POINT('Ctrl Pts',(4.09137516053085,-16.8268077199093,-72.8625769660851));
#38950=CARTESIAN_POINT('Ctrl Pts',(4.53567658281545,-16.3991227020429,-73.3355464350895));
#38951=CARTESIAN_POINT('Ctrl Pts',(4.787383015671,-15.9274342791999,-73.6132058254433));
#38952=CARTESIAN_POINT('Ctrl Pts',(4.83333333333332,-15.6672482052684,-73.6666666666667));
#38953=CARTESIAN_POINT('Ctrl Pts',(4.83333333333332,-15.5,-73.6666666666667));
#38954=CARTESIAN_POINT('Ctrl Pts',(3.10367510160593,-16.9981470538884,-72.3391048451961));
#38955=CARTESIAN_POINT('Ctrl Pts',(3.35716302579492,-16.9854005733312,-72.5939510924519));
#38956=CARTESIAN_POINT('Ctrl Pts',(3.86257696608514,-16.8268077199093,-73.0913751605309));
#38957=CARTESIAN_POINT('Ctrl Pts',(4.33554643508949,-16.3991227020429,-73.5356765828154));
#38958=CARTESIAN_POINT('Ctrl Pts',(4.61320582544332,-15.9274342791999,-73.787383015671));
#38959=CARTESIAN_POINT('Ctrl Pts',(4.66666666666665,-15.6672482052684,-73.8333333333333));
#38960=CARTESIAN_POINT('Ctrl Pts',(4.66666666666665,-15.5,-73.8333333333333));
#38961=CARTESIAN_POINT('Ctrl Pts',(2.86824535801577,-16.9981470538884,-72.5745345887863));
#38962=CARTESIAN_POINT('Ctrl Pts',(3.12037495913793,-16.9854005733312,-72.8307391591089));
#38963=CARTESIAN_POINT('Ctrl Pts',(3.63377877163942,-16.8268077199093,-73.3201733549766));
#38964=CARTESIAN_POINT('Ctrl Pts',(4.13541628736353,-16.3991227020429,-73.7358067305414));
#38965=CARTESIAN_POINT('Ctrl Pts',(4.43902863521563,-15.9274342791999,-73.9615602058987));
#38966=CARTESIAN_POINT('Ctrl Pts',(4.49999999999999,-15.6672482052684,-74.));
#38967=CARTESIAN_POINT('Ctrl Pts',(4.49999999999999,-15.5,-74.));
#38968=CARTESIAN_POINT('',(4.99999999999999,-15.5,-73.5));
#38969=CARTESIAN_POINT('',(4.49999999999999,-15.5,-74.));
#38970=CARTESIAN_POINT('Ctrl Pts',(4.99999999999999,-15.5,-73.5));
#38971=CARTESIAN_POINT('Ctrl Pts',(4.99999999999999,-15.6672482052684,-73.5));
#38972=CARTESIAN_POINT('Ctrl Pts',(4.96156020589869,-15.9274342791999,-73.4390286352156));
#38973=CARTESIAN_POINT('Ctrl Pts',(4.7358067305414,-16.3991227020429,-73.1354162873635));
#38974=CARTESIAN_POINT('Ctrl Pts',(4.32017335497657,-16.8268077199093,-72.6337787716394));
#38975=CARTESIAN_POINT('Ctrl Pts',(3.83073915910889,-16.9854005733312,-72.1203749591379));
#38976=CARTESIAN_POINT('Ctrl Pts',(3.57453458878624,-16.9981470538884,-71.8682453580158));
#38977=CARTESIAN_POINT('Origin',(4.74999999999999,-14.,-73.75));
#38978=CARTESIAN_POINT('',(4.99999999999999,-14.,-73.5));
#38979=CARTESIAN_POINT('',(44.75,-14.,-33.7499999999994));
#38980=CARTESIAN_POINT('',(4.99999999999999,-14.,-73.5));
#38981=CARTESIAN_POINT('Origin',(3.49999999999999,-15.5,-68.));
#38982=CARTESIAN_POINT('',(4.99999999999999,-15.5,-56.2783262011229));
#38983=CARTESIAN_POINT('',(4.99999999999999,-15.5,-68.));
#38984=CARTESIAN_POINT('Ctrl Pts',(3.49999999999999,-17.,-56.3914887194867));
#38985=CARTESIAN_POINT('Ctrl Pts',(3.68849285843232,-17.,-56.379789702144));
#38986=CARTESIAN_POINT('Ctrl Pts',(3.88949595769793,-16.9623071985392,-56.366268079425));
#38987=CARTESIAN_POINT('Ctrl Pts',(4.25923828551907,-16.8090480003591,-56.3395353657988));
#38988=CARTESIAN_POINT('Ctrl Pts',(4.42798167302477,-16.6934822832211,-56.3263779287031));
#38989=CARTESIAN_POINT('Ctrl Pts',(4.69412389350912,-16.4270526075957,-56.3048219679644));
#38990=CARTESIAN_POINT('Ctrl Pts',(4.80941523738749,-16.2585410496607,-56.2949857165266));
#38991=CARTESIAN_POINT('Ctrl Pts',(4.96235566707567,-15.889189778178,-56.2817103328366));
#38992=CARTESIAN_POINT('Ctrl Pts',(4.99999999999999,-15.6883461217826,-56.2783262011229));
#38993=CARTESIAN_POINT('Ctrl Pts',(4.99999999999999,-15.5,-56.2783262011229));
#38994=CARTESIAN_POINT('Origin',(4.99999999999999,-14.,-74.));
#38995=CARTESIAN_POINT('',(4.99999999999999,-14.,-56.2783262011229));
#38996=CARTESIAN_POINT('',(5.,-14.,8.5));
#38997=CARTESIAN_POINT('',(4.99999999999999,-16.45,-56.2783262011229));
#38998=CARTESIAN_POINT('Ctrl Pts',(-71.8682453580158,-16.9981470538884,
3.57453458878626));
#38999=CARTESIAN_POINT('Ctrl Pts',(-71.8641633585059,-16.9983534204838,
3.57038661518134));
#39000=CARTESIAN_POINT('Ctrl Pts',(-71.834280745957,-16.9997799301677,3.5399078658621));
#39001=CARTESIAN_POINT('Ctrl Pts',(-71.8016132291015,-16.9999870327594,
3.50642976897921));
#39002=CARTESIAN_POINT('Ctrl Pts',(-71.7963365978802,-17.,3.50104102377552));
#39003=CARTESIAN_POINT('Ctrl Pts',(-71.7953186364093,-17.,3.50000000000001));
#39004=CARTESIAN_POINT('Ctrl Pts',(-72.1036751016059,-16.9981470538884,
3.33910484519611));
#39005=CARTESIAN_POINT('Ctrl Pts',(-72.0995711107311,-16.9983534204838,
3.33497886295621));
#39006=CARTESIAN_POINT('Ctrl Pts',(-72.0694570586097,-16.9997799301677,
3.30473155320942));
#39007=CARTESIAN_POINT('Ctrl Pts',(-72.0365616348729,-16.9999870327594,
3.27148136320786));
#39008=CARTESIAN_POINT('Ctrl Pts',(-72.0312380731786,-17.,3.26613954847709));
#39009=CARTESIAN_POINT('Ctrl Pts',(-72.0302124242728,-17.,3.26510621213643));
#39010=CARTESIAN_POINT('Ctrl Pts',(-72.3391048451961,-16.9981470538884,
3.10367510160595));
#39011=CARTESIAN_POINT('Ctrl Pts',(-72.3349788629562,-16.9983534204838,
3.09957111073108));
#39012=CARTESIAN_POINT('Ctrl Pts',(-72.3045547255514,-17.0000242835561,
3.06945705860968));
#39013=CARTESIAN_POINT('Ctrl Pts',(-72.2714568031683,-16.9998354184739,
3.03656163487291));
#39014=CARTESIAN_POINT('Ctrl Pts',(-72.2661395484771,-17.,3.03123807317866));
#39015=CARTESIAN_POINT('Ctrl Pts',(-72.2651062121364,-17.,3.03021242427285));
#39016=CARTESIAN_POINT('Ctrl Pts',(-72.5745345887863,-16.9981470538884,
2.86824535801579));
#39017=CARTESIAN_POINT('Ctrl Pts',(-72.5703866151813,-16.9983534204838,
2.86416335850595));
#39018=CARTESIAN_POINT('Ctrl Pts',(-72.5399078658621,-16.9997799301677,
2.834280745957));
#39019=CARTESIAN_POINT('Ctrl Pts',(-72.5064297689792,-16.9999870327594,
2.80161322910156));
#39020=CARTESIAN_POINT('Ctrl Pts',(-72.5010410237755,-17.,2.79633659788023));
#39021=CARTESIAN_POINT('Ctrl Pts',(-72.5,-17.,2.79531863640927));
#39022=CARTESIAN_POINT('',(-71.7953186364093,-17.,3.50000000000001));
#39023=CARTESIAN_POINT('',(-71.8682453580158,-16.9981470538884,3.57453458878626));
#39024=CARTESIAN_POINT('Ctrl Pts',(-71.7953186364093,-17.,3.50000000000001));
#39025=CARTESIAN_POINT('Ctrl Pts',(-71.7956426566413,-17.,3.50033136103369));
#39026=CARTESIAN_POINT('Ctrl Pts',(-71.7959698710105,-16.9999999087783,
3.5006659910395));
#39027=CARTESIAN_POINT('Ctrl Pts',(-71.7963728195339,-16.9999996125274,
3.50107815475912));
#39028=CARTESIAN_POINT('Ctrl Pts',(-71.7967957210522,-16.9999993016069,
3.501510727787));
#39029=CARTESIAN_POINT('Ctrl Pts',(-71.7973018394015,-16.999998768055,3.50202849537427));
#39030=CARTESIAN_POINT('Ctrl Pts',(-71.7979344421874,-16.9999976134245,
3.50267576544801));
#39031=CARTESIAN_POINT('Ctrl Pts',(-71.7986084157221,-16.9999963832839,
3.50336536547696));
#39032=CARTESIAN_POINT('Ctrl Pts',(-71.7994256794686,-16.9999944448324,
3.50420167541483));
#39033=CARTESIAN_POINT('Ctrl Pts',(-71.8003972134396,-16.9999910006556,
3.50519595537295));
#39034=CARTESIAN_POINT('Ctrl Pts',(-71.8014697058444,-16.9999871985718,
3.50629355744889));
#39035=CARTESIAN_POINT('Ctrl Pts',(-71.8027297908792,-16.9999815341953,
3.50758325228928));
#39036=CARTESIAN_POINT('Ctrl Pts',(-71.804148443709,-16.9999727872824,3.50903534240298));
#39037=CARTESIAN_POINT('Ctrl Pts',(-71.8059282949087,-16.9999618133477,
3.51085714423967));
#39038=CARTESIAN_POINT('Ctrl Pts',(-71.8079568545964,-16.9999458718544,
3.51293366154214));
#39039=CARTESIAN_POINT('Ctrl Pts',(-71.8101187023244,-16.9999235237508,
3.51514671247923));
#39040=CARTESIAN_POINT('Ctrl Pts',(-71.8124121613863,-16.9998998151149,
3.51749449195529));
#39041=CARTESIAN_POINT('Ctrl Pts',(-71.8148508937685,-16.9998688531822,
3.51999108761016));
#39042=CARTESIAN_POINT('Ctrl Pts',(-71.8172869062403,-16.9998314674613,
3.52248486630895));
#39043=CARTESIAN_POINT('Ctrl Pts',(-71.8191324991579,-16.9998031429668,
3.52437422457693));
#39044=CARTESIAN_POINT('Ctrl Pts',(-71.8209757293309,-16.9997712320714,
3.52626114404865));
#39045=CARTESIAN_POINT('Ctrl Pts',(-71.822775757931,-16.9997367040829,3.52810370841081));
#39046=CARTESIAN_POINT('Ctrl Pts',(-71.824400036902,-16.9997055473083,3.5297663700741));
#39047=CARTESIAN_POINT('Ctrl Pts',(-71.8259887368554,-16.9996723091153,
3.531392504458));
#39048=CARTESIAN_POINT('Ctrl Pts',(-71.8275407505538,-16.9996373773349,
3.53298085050784));
#39049=CARTESIAN_POINT('Ctrl Pts',(-71.8290718023241,-16.9996029173527,
3.53454774391476));
#39050=CARTESIAN_POINT('Ctrl Pts',(-71.8305664957212,-16.9995668629652,
3.53607719242319));
#39051=CARTESIAN_POINT('Ctrl Pts',(-71.8320614739056,-16.9995285090951,
3.53760652085704));
#39052=CARTESIAN_POINT('Ctrl Pts',(-71.8335194958997,-16.9994911033411,
3.53909804395481));
#39053=CARTESIAN_POINT('Ctrl Pts',(-71.8349843334467,-16.9994513364011,
3.54059613558254));
#39054=CARTESIAN_POINT('Ctrl Pts',(-71.8364852326094,-16.9994082206029,
3.54213060631522));
#39055=CARTESIAN_POINT('Ctrl Pts',(-71.838098400887,-16.9993618796896,3.54377985735778));
#39056=CARTESIAN_POINT('Ctrl Pts',(-71.8397528770161,-16.9993116397098,
3.54547077478745));
#39057=CARTESIAN_POINT('Ctrl Pts',(-71.8414428847976,-16.9992572833264,
3.54719744053049));
#39058=CARTESIAN_POINT('Ctrl Pts',(-71.8433735916156,-16.9991951852455,
3.54917002631327));
#39059=CARTESIAN_POINT('Ctrl Pts',(-71.8453501484935,-16.9991276636876,
3.55118873161006));
#39060=CARTESIAN_POINT('Ctrl Pts',(-71.8473171286804,-16.9990563957717,
3.5531970139764));
#39061=CARTESIAN_POINT('Ctrl Pts',(-71.850042283731,-16.9989576575525,3.55597939118077));
#39062=CARTESIAN_POINT('Ctrl Pts',(-71.8527461713316,-16.9988515979041,
3.55873880451969));
#39063=CARTESIAN_POINT('Ctrl Pts',(-71.8552161386875,-16.9987486082515,
3.56125854441668));
#39064=CARTESIAN_POINT('Ctrl Pts',(-71.8570686142045,-16.9986713660121,
3.56314834933943));
#39065=CARTESIAN_POINT('Ctrl Pts',(-71.8587868623064,-16.998596102758,3.56490064570679));
#39066=CARTESIAN_POINT('Ctrl Pts',(-71.8602963585414,-16.9985278711001,
3.56643959313713));
#39067=CARTESIAN_POINT('Ctrl Pts',(-71.8615610437188,-16.9984707052957,
3.56772895309641));
#39068=CARTESIAN_POINT('Ctrl Pts',(-71.8626788313974,-16.9984185388897,
3.56886818435391));
#39069=CARTESIAN_POINT('Ctrl Pts',(-71.8636316653216,-16.998373289921,3.56983898661485));
#39070=CARTESIAN_POINT('Ctrl Pts',(-71.8645275000201,-16.9983307477788,
3.57075171477107));
#39071=CARTESIAN_POINT('Ctrl Pts',(-71.8652771155594,-16.9982943574932,
3.57151514502294));
#39072=CARTESIAN_POINT('Ctrl Pts',(-71.8658958651526,-16.9982640274543,
3.57214502087136));
#39073=CARTESIAN_POINT('Ctrl Pts',(-71.8664725654874,-16.9982357585976,
3.57273209133846));
#39074=CARTESIAN_POINT('Ctrl Pts',(-71.8669354348749,-16.9982127623775,
3.57320299278071));
#39075=CARTESIAN_POINT('Ctrl Pts',(-71.867327729259,-16.9981931657129,3.57360188999624));
#39076=CARTESIAN_POINT('Ctrl Pts',(-71.8676698713729,-16.9981760743537,
3.57394979081275));
#39077=CARTESIAN_POINT('Ctrl Pts',(-71.8679585937125,-16.9981615513357,
3.57424318974083));
#39078=CARTESIAN_POINT('Ctrl Pts',(-71.8682453580158,-16.9981470538884,
3.57453458878627));
#39079=CARTESIAN_POINT('',(-72.5745345887863,-16.9981470538884,2.86824535801579));
#39080=CARTESIAN_POINT('Ctrl Pts',(-72.5745345887863,-16.9981470538884,
2.86824535801579));
#39081=CARTESIAN_POINT('Ctrl Pts',(-72.3391048451961,-16.9981470538884,
3.10367510160595));
#39082=CARTESIAN_POINT('Ctrl Pts',(-72.1036751016059,-16.9981470538884,
3.33910484519611));
#39083=CARTESIAN_POINT('Ctrl Pts',(-71.8682453580158,-16.9981470538884,
3.57453458878626));
#39084=CARTESIAN_POINT('',(-72.5,-17.,2.79531863640927));
#39085=CARTESIAN_POINT('Ctrl Pts',(-72.5745345887863,-16.9981470538884,
2.86824535801579));
#39086=CARTESIAN_POINT('Ctrl Pts',(-72.5742044925281,-16.9981634765679,
2.86792051198432));
#39087=CARTESIAN_POINT('Ctrl Pts',(-72.5738711310018,-16.9981799708645,
2.86759246756108));
#39088=CARTESIAN_POINT('Ctrl Pts',(-72.57346041281,-16.9982001093812,2.86718860352498));
#39089=CARTESIAN_POINT('Ctrl Pts',(-72.57302935509,-16.9982212451946,2.8667647393911));
#39090=CARTESIAN_POINT('Ctrl Pts',(-72.5725132968389,-16.9982463879926,
2.86625756382415));
#39091=CARTESIAN_POINT('Ctrl Pts',(-72.5718680115171,-16.9982773404549,
2.86562376912052));
#39092=CARTESIAN_POINT('Ctrl Pts',(-72.5711805211291,-16.9983103173716,
2.86494852089772));
#39093=CARTESIAN_POINT('Ctrl Pts',(-72.5703466306137,-16.9983498713227,
2.86412982782488));
#39094=CARTESIAN_POINT('Ctrl Pts',(-72.5693550535868,-16.9983957676602,
2.86315671761944));
#39095=CARTESIAN_POINT('Ctrl Pts',(-72.5682604104266,-16.9984464345378,
2.86208246075231));
#39096=CARTESIAN_POINT('Ctrl Pts',(-72.5669740091159,-16.9985047829815,
2.86082042406595));
#39097=CARTESIAN_POINT('Ctrl Pts',(-72.565525387959,-16.9985681244217,2.85939970674287));
#39098=CARTESIAN_POINT('Ctrl Pts',(-72.5637077270911,-16.9986476022457,
2.85761705827722));
#39099=CARTESIAN_POINT('Ctrl Pts',(-72.5616355608823,-16.9987347812318,
2.85558546640715));
#39100=CARTESIAN_POINT('Ctrl Pts',(-72.5594266767905,-16.9988223610841,
2.85342062894716));
#39101=CARTESIAN_POINT('Ctrl Pts',(-72.5570842219804,-16.9989152368701,
2.85112488425854));
#39102=CARTESIAN_POINT('Ctrl Pts',(-72.5545928471897,-16.9990082804756,
2.84868403352371));
#39103=CARTESIAN_POINT('Ctrl Pts',(-72.552103587594,-16.9990947989236,2.84624625175195));
#39104=CARTESIAN_POINT('Ctrl Pts',(-72.5502173068831,-16.9991603598156,
2.84439897927725));
#39105=CARTESIAN_POINT('Ctrl Pts',(-72.5483330647398,-16.9992222334679,
2.84255427195848));
#39106=CARTESIAN_POINT('Ctrl Pts',(-72.5464926261216,-16.9992793054386,
2.84075306394266));
#39107=CARTESIAN_POINT('Ctrl Pts',(-72.5448318572274,-16.9993308058541,
2.83912769582928));
#39108=CARTESIAN_POINT('Ctrl Pts',(-72.543207168852,-16.9993784253393,2.83753815081149));
#39109=CARTESIAN_POINT('Ctrl Pts',(-72.5416197584348,-16.9994224873957,
2.83598557864455));
#39110=CARTESIAN_POINT('Ctrl Pts',(-72.540053319257,-16.9994659673493,2.83445351746978));
#39111=CARTESIAN_POINT('Ctrl Pts',(-72.5385238533706,-16.9995060035546,
2.83295811821706));
#39112=CARTESIAN_POINT('Ctrl Pts',(-72.5369939676884,-16.9995437460623,
2.83146270058429));
#39113=CARTESIAN_POINT('Ctrl Pts',(-72.5355023760137,-16.9995805438512,
2.8300047142019));
#39114=CARTESIAN_POINT('Ctrl Pts',(-72.5340037037557,-16.9996153196962,
2.82854016663104));
#39115=CARTESIAN_POINT('Ctrl Pts',(-72.5324681805947,-16.9996485645807,
2.82703981578639));
#39116=CARTESIAN_POINT('Ctrl Pts',(-72.5308177719951,-16.9996842967954,
2.82542721104074));
#39117=CARTESIAN_POINT('Ctrl Pts',(-72.529125149268,-16.9997182120423,2.82377359513262));
#39118=CARTESIAN_POINT('Ctrl Pts',(-72.5273963190708,-16.9997497930326,
2.82208470500297));
#39119=CARTESIAN_POINT('Ctrl Pts',(-72.5254211385424,-16.9997858741684,
2.82015515581749));
#39120=CARTESIAN_POINT('Ctrl Pts',(-72.5233992312896,-16.9998188305302,
2.81818008615893));
#39121=CARTESIAN_POINT('Ctrl Pts',(-72.52138736276,-16.9998475191546,2.81621482751818));
#39122=CARTESIAN_POINT('Ctrl Pts',(-72.5186005402078,-16.9998872583841,
2.81349256857324));
#39123=CARTESIAN_POINT('Ctrl Pts',(-72.5158359360068,-16.9999185308537,
2.81079201806524));
#39124=CARTESIAN_POINT('Ctrl Pts',(-72.5133109478137,-16.9999409383933,
2.8083253911404));
#39125=CARTESIAN_POINT('Ctrl Pts',(-72.5114172066689,-16.9999577440481,
2.80647542094676));
#39126=CARTESIAN_POINT('Ctrl Pts',(-72.5096609508553,-16.9999696816405,
2.80475967567115));
#39127=CARTESIAN_POINT('Ctrl Pts',(-72.508118309431,-16.9999780308564,2.803252515256));
#39128=CARTESIAN_POINT('Ctrl Pts',(-72.5068258239488,-16.999985026157,2.80198975715482));
#39129=CARTESIAN_POINT('Ctrl Pts',(-72.5056836631397,-16.9999895478102,
2.80087378577512));
#39130=CARTESIAN_POINT('Ctrl Pts',(-72.5047102375997,-16.9999926045357,
2.79992260032024));
#39131=CARTESIAN_POINT('Ctrl Pts',(-72.5037950311059,-16.9999954784432,
2.7990283037671));
#39132=CARTESIAN_POINT('Ctrl Pts',(-72.5030293988184,-16.9999970739683,
2.79828008131995));
#39133=CARTESIAN_POINT('Ctrl Pts',(-72.5023976001144,-16.9999980838367,
2.797662574869));
#39134=CARTESIAN_POINT('Ctrl Pts',(-72.5018087302087,-16.9999990250876,
2.79708702610117));
#39135=CARTESIAN_POINT('Ctrl Pts',(-72.5013362750362,-16.9999994582021,
2.79662518068281));
#39136=CARTESIAN_POINT('Ctrl Pts',(-72.500935978419,-16.9999997079814,2.79623381941523));
#39137=CARTESIAN_POINT('Ctrl Pts',(-72.5005869205336,-16.9999999257886,
2.79589255313754));
#39138=CARTESIAN_POINT('Ctrl Pts',(-72.5002924603909,-17.,2.79560461778333));
#39139=CARTESIAN_POINT('Ctrl Pts',(-72.5,-17.,2.79531863640927));
#39140=CARTESIAN_POINT('',(-72.1476593182046,-17.,3.14765931820464));
#39141=CARTESIAN_POINT('Ctrl Pts',(-72.5745345887863,-16.9981470538884,
2.86824535801579));
#39142=CARTESIAN_POINT('Ctrl Pts',(-72.9588414442702,-16.9790273330526,
3.24643975969903));
#39143=CARTESIAN_POINT('Ctrl Pts',(-73.5507380181504,-16.6911512202391,
3.89283858086127));
#39144=CARTESIAN_POINT('Ctrl Pts',(-73.9509340499422,-16.0144112572066,
4.4212646197358));
#39145=CARTESIAN_POINT('Ctrl Pts',(-74.,-15.6672482052684,4.50000000000001));
#39146=CARTESIAN_POINT('Ctrl Pts',(-74.,-15.5,4.50000000000001));
#39147=CARTESIAN_POINT('Ctrl Pts',(-72.3391048451961,-16.9981470538884,
3.10367510160595));
#39148=CARTESIAN_POINT('Ctrl Pts',(-72.7213742160798,-16.9790273330526,
3.48390698788944));
#39149=CARTESIAN_POINT('Ctrl Pts',(-73.3314382057207,-16.6911512202391,
4.11213839329095));
#39150=CARTESIAN_POINT('Ctrl Pts',(-73.7743775732067,-16.0144112572066,
4.59782109647127));
#39151=CARTESIAN_POINT('Ctrl Pts',(-73.8333333333333,-15.6672482052684,
4.66666666666667));
#39152=CARTESIAN_POINT('Ctrl Pts',(-73.8333333333333,-15.5,4.66666666666667));
#39153=CARTESIAN_POINT('Ctrl Pts',(-72.1036751016059,-16.9981470538884,
3.33910484519611));
#39154=CARTESIAN_POINT('Ctrl Pts',(-72.4839069878894,-16.9790273330526,
3.72137421607984));
#39155=CARTESIAN_POINT('Ctrl Pts',(-73.112138393291,-16.6911512202391,4.33143820572064));
#39156=CARTESIAN_POINT('Ctrl Pts',(-73.5978210964713,-16.0144112572066,
4.77437757320674));
#39157=CARTESIAN_POINT('Ctrl Pts',(-73.6666666666667,-15.6672482052684,
4.83333333333334));
#39158=CARTESIAN_POINT('Ctrl Pts',(-73.6666666666667,-15.5,4.83333333333334));
#39159=CARTESIAN_POINT('Ctrl Pts',(-71.8682453580158,-16.9981470538884,
3.57453458878626));
#39160=CARTESIAN_POINT('Ctrl Pts',(-72.246439759699,-16.9790273330526,3.95884144427024));
#39161=CARTESIAN_POINT('Ctrl Pts',(-72.8928385808613,-16.6911512202391,
4.55073801815033));
#39162=CARTESIAN_POINT('Ctrl Pts',(-73.4212646197358,-16.0144112572066,
4.95093404994221));
#39163=CARTESIAN_POINT('Ctrl Pts',(-73.5,-15.6672482052684,5.00000000000001));
#39164=CARTESIAN_POINT('Ctrl Pts',(-73.5,-15.5,5.00000000000001));
#39165=CARTESIAN_POINT('',(-73.5,-15.5,5.00000000000001));
#39166=CARTESIAN_POINT('Ctrl Pts',(-71.8682453580158,-16.9981470538884,
3.57453458878626));
#39167=CARTESIAN_POINT('Ctrl Pts',(-72.246439759699,-16.9790273330526,3.95884144427024));
#39168=CARTESIAN_POINT('Ctrl Pts',(-72.8928385808613,-16.6911512202391,
4.55073801815033));
#39169=CARTESIAN_POINT('Ctrl Pts',(-73.4212646197358,-16.0144112572066,
4.95093404994221));
#39170=CARTESIAN_POINT('Ctrl Pts',(-73.5,-15.6672482052684,5.00000000000001));
#39171=CARTESIAN_POINT('Ctrl Pts',(-73.5,-15.5,5.00000000000001));
#39172=CARTESIAN_POINT('',(-74.,-15.5,4.50000000000001));
#39173=CARTESIAN_POINT('',(-73.5,-15.5,5.00000000000001));
#39174=CARTESIAN_POINT('Ctrl Pts',(-74.,-15.5,4.50000000000001));
#39175=CARTESIAN_POINT('Ctrl Pts',(-74.,-15.6672482052684,4.50000000000001));
#39176=CARTESIAN_POINT('Ctrl Pts',(-73.9509340499422,-16.0144112572066,
4.4212646197358));
#39177=CARTESIAN_POINT('Ctrl Pts',(-73.5507380181504,-16.6911512202391,
3.89283858086127));
#39178=CARTESIAN_POINT('Ctrl Pts',(-72.9588414442702,-16.9790273330526,
3.24643975969903));
#39179=CARTESIAN_POINT('Ctrl Pts',(-72.5745345887863,-16.9981470538884,
2.86824535801579));
#39180=CARTESIAN_POINT('Origin',(-73.75,-14.,4.75000000000001));
#39181=CARTESIAN_POINT('',(-73.5,-14.,5.));
#39182=CARTESIAN_POINT('',(-74.,-14.,4.50000000000001));
#39183=CARTESIAN_POINT('',(-33.7500000000001,-14.,44.7500000000001));
#39184=CARTESIAN_POINT('',(-74.,-14.,4.50000000000001));
#39185=CARTESIAN_POINT('',(-73.5,-14.,5.00000000000001));
#39186=CARTESIAN_POINT('Origin',(-62.,-17.,7.7715611723761E-15));
#39187=CARTESIAN_POINT('',(-72.5,-17.,-3.49999999999999));
#39188=CARTESIAN_POINT('',(-72.5,-17.,2.50000000000001));
#39189=CARTESIAN_POINT('',(-56.3914887194867,-17.,-3.49999999999999));
#39190=CARTESIAN_POINT('',(-68.,-17.,-3.49999999999999));
#39191=CARTESIAN_POINT('',(-56.3914887194867,-17.,3.50000000000001));
#39192=CARTESIAN_POINT('Origin',(0.,-17.,0.));
#39193=CARTESIAN_POINT('',(-56.,-17.,3.50000000000001));
#39194=CARTESIAN_POINT('Origin',(-72.5,-15.5,2.50000000000001));
#39195=CARTESIAN_POINT('',(-74.,-15.5,-3.49999999999999));
#39196=CARTESIAN_POINT('',(-74.,-15.5,2.50000000000001));
#39197=CARTESIAN_POINT('Origin',(-72.5,-15.5,-3.49999999999999));
#39198=CARTESIAN_POINT('Origin',(-74.,-14.,5.00000000000001));
#39199=CARTESIAN_POINT('',(-74.,-14.,-3.49999999999999));
#39200=CARTESIAN_POINT('',(-74.,-14.,48.));
#39201=CARTESIAN_POINT('',(-74.,-14.,-3.49999999999999));
#39202=CARTESIAN_POINT('Ctrl Pts',(3.57453458878626,-16.9981470538884,71.8682453580158));
#39203=CARTESIAN_POINT('Ctrl Pts',(3.57038661518133,-16.9983534204838,71.8641633585059));
#39204=CARTESIAN_POINT('Ctrl Pts',(3.5399078658621,-16.9997799301677,71.834280745957));
#39205=CARTESIAN_POINT('Ctrl Pts',(3.5064297689792,-16.9999870327594,71.8016132291015));
#39206=CARTESIAN_POINT('Ctrl Pts',(3.50104102377552,-17.,71.7963365978802));
#39207=CARTESIAN_POINT('Ctrl Pts',(3.5,-17.,71.7953186364093));
#39208=CARTESIAN_POINT('Ctrl Pts',(3.3391048451961,-16.9981470538884,72.1036751016059));
#39209=CARTESIAN_POINT('Ctrl Pts',(3.3349788629562,-16.9983534204838,72.0995711107311));
#39210=CARTESIAN_POINT('Ctrl Pts',(3.30473155320942,-16.9997799301677,72.0694570586097));
#39211=CARTESIAN_POINT('Ctrl Pts',(3.27148136320786,-16.9999870327594,72.0365616348729));
#39212=CARTESIAN_POINT('Ctrl Pts',(3.26613954847709,-17.,72.0312380731786));
#39213=CARTESIAN_POINT('Ctrl Pts',(3.26510621213643,-17.,72.0302124242728));
#39214=CARTESIAN_POINT('Ctrl Pts',(3.10367510160595,-16.9981470538884,72.3391048451961));
#39215=CARTESIAN_POINT('Ctrl Pts',(3.09957111073108,-16.9983534204838,72.3349788629562));
#39216=CARTESIAN_POINT('Ctrl Pts',(3.06945705860968,-17.0000242835561,72.3045547255514));
#39217=CARTESIAN_POINT('Ctrl Pts',(3.03656163487291,-16.9998354184739,72.2714568031683));
#39218=CARTESIAN_POINT('Ctrl Pts',(3.03123807317865,-17.,72.2661395484771));
#39219=CARTESIAN_POINT('Ctrl Pts',(3.03021242427285,-17.,72.2651062121364));
#39220=CARTESIAN_POINT('Ctrl Pts',(2.86824535801579,-16.9981470538884,72.5745345887863));
#39221=CARTESIAN_POINT('Ctrl Pts',(2.86416335850595,-16.9983534204838,72.5703866151813));
#39222=CARTESIAN_POINT('Ctrl Pts',(2.83428074595699,-16.9997799301677,72.5399078658621));
#39223=CARTESIAN_POINT('Ctrl Pts',(2.80161322910156,-16.9999870327594,72.5064297689792));
#39224=CARTESIAN_POINT('Ctrl Pts',(2.79633659788022,-17.,72.5010410237755));
#39225=CARTESIAN_POINT('Ctrl Pts',(2.79531863640927,-17.,72.5));
#39226=CARTESIAN_POINT('',(3.5,-17.,71.7953186364093));
#39227=CARTESIAN_POINT('',(3.57453458878626,-16.9981470538884,71.8682453580158));
#39228=CARTESIAN_POINT('Ctrl Pts',(3.50000000000001,-17.,71.7953186364093));
#39229=CARTESIAN_POINT('Ctrl Pts',(3.50033136103368,-17.,71.7956426566413));
#39230=CARTESIAN_POINT('Ctrl Pts',(3.5006659910395,-16.9999999087783,71.7959698710105));
#39231=CARTESIAN_POINT('Ctrl Pts',(3.50107815475912,-16.9999996125274,71.7963728195339));
#39232=CARTESIAN_POINT('Ctrl Pts',(3.50151072778699,-16.9999993016069,71.7967957210522));
#39233=CARTESIAN_POINT('Ctrl Pts',(3.50202849537426,-16.999998768055,71.7973018394015));
#39234=CARTESIAN_POINT('Ctrl Pts',(3.50267576544801,-16.9999976134245,71.7979344421874));
#39235=CARTESIAN_POINT('Ctrl Pts',(3.50336536547695,-16.9999963832839,71.7986084157221));
#39236=CARTESIAN_POINT('Ctrl Pts',(3.50420167541483,-16.9999944448324,71.7994256794686));
#39237=CARTESIAN_POINT('Ctrl Pts',(3.50519595537295,-16.9999910006556,71.8003972134396));
#39238=CARTESIAN_POINT('Ctrl Pts',(3.50629355744888,-16.9999871985718,71.8014697058444));
#39239=CARTESIAN_POINT('Ctrl Pts',(3.50758325228927,-16.9999815341953,71.8027297908792));
#39240=CARTESIAN_POINT('Ctrl Pts',(3.50903534240298,-16.9999727872824,71.804148443709));
#39241=CARTESIAN_POINT('Ctrl Pts',(3.51085714423966,-16.9999618133477,71.8059282949087));
#39242=CARTESIAN_POINT('Ctrl Pts',(3.51293366154214,-16.9999458718544,71.8079568545964));
#39243=CARTESIAN_POINT('Ctrl Pts',(3.51514671247922,-16.9999235237508,71.8101187023244));
#39244=CARTESIAN_POINT('Ctrl Pts',(3.51749449195528,-16.9998998151149,71.8124121613863));
#39245=CARTESIAN_POINT('Ctrl Pts',(3.51999108761016,-16.9998688531822,71.8148508937685));
#39246=CARTESIAN_POINT('Ctrl Pts',(3.52248486630895,-16.9998314674613,71.8172869062403));
#39247=CARTESIAN_POINT('Ctrl Pts',(3.52437422457692,-16.9998031429668,71.8191324991579));
#39248=CARTESIAN_POINT('Ctrl Pts',(3.52626114404864,-16.9997712320714,71.8209757293309));
#39249=CARTESIAN_POINT('Ctrl Pts',(3.5281037084108,-16.9997367040829,71.822775757931));
#39250=CARTESIAN_POINT('Ctrl Pts',(3.52976637007409,-16.9997055473083,71.824400036902));
#39251=CARTESIAN_POINT('Ctrl Pts',(3.531392504458,-16.9996723091153,71.8259887368554));
#39252=CARTESIAN_POINT('Ctrl Pts',(3.53298085050783,-16.9996373773349,71.8275407505538));
#39253=CARTESIAN_POINT('Ctrl Pts',(3.53454774391476,-16.9996029173527,71.8290718023241));
#39254=CARTESIAN_POINT('Ctrl Pts',(3.53607719242319,-16.9995668629652,71.8305664957212));
#39255=CARTESIAN_POINT('Ctrl Pts',(3.53760652085704,-16.9995285090951,71.8320614739056));
#39256=CARTESIAN_POINT('Ctrl Pts',(3.5390980439548,-16.9994911033411,71.8335194958997));
#39257=CARTESIAN_POINT('Ctrl Pts',(3.54059613558254,-16.9994513364011,71.8349843334467));
#39258=CARTESIAN_POINT('Ctrl Pts',(3.54213060631522,-16.9994082206029,71.8364852326094));
#39259=CARTESIAN_POINT('Ctrl Pts',(3.54377985735778,-16.9993618796896,71.838098400887));
#39260=CARTESIAN_POINT('Ctrl Pts',(3.54547077478744,-16.9993116397098,71.8397528770161));
#39261=CARTESIAN_POINT('Ctrl Pts',(3.54719744053048,-16.9992572833264,71.8414428847976));
#39262=CARTESIAN_POINT('Ctrl Pts',(3.54917002631327,-16.9991951852455,71.8433735916156));
#39263=CARTESIAN_POINT('Ctrl Pts',(3.55118873161006,-16.9991276636876,71.8453501484935));
#39264=CARTESIAN_POINT('Ctrl Pts',(3.5531970139764,-16.9990563957717,71.8473171286804));
#39265=CARTESIAN_POINT('Ctrl Pts',(3.55597939118076,-16.9989576575525,71.850042283731));
#39266=CARTESIAN_POINT('Ctrl Pts',(3.55873880451969,-16.9988515979041,71.8527461713316));
#39267=CARTESIAN_POINT('Ctrl Pts',(3.56125854441668,-16.9987486082515,71.8552161386875));
#39268=CARTESIAN_POINT('Ctrl Pts',(3.56314834933942,-16.9986713660121,71.8570686142045));
#39269=CARTESIAN_POINT('Ctrl Pts',(3.56490064570679,-16.998596102758,71.8587868623064));
#39270=CARTESIAN_POINT('Ctrl Pts',(3.56643959313712,-16.9985278711001,71.8602963585414));
#39271=CARTESIAN_POINT('Ctrl Pts',(3.5677289530964,-16.9984707052957,71.8615610437188));
#39272=CARTESIAN_POINT('Ctrl Pts',(3.5688681843539,-16.9984185388897,71.8626788313974));
#39273=CARTESIAN_POINT('Ctrl Pts',(3.56983898661485,-16.998373289921,71.8636316653216));
#39274=CARTESIAN_POINT('Ctrl Pts',(3.57075171477106,-16.9983307477788,71.8645275000201));
#39275=CARTESIAN_POINT('Ctrl Pts',(3.57151514502293,-16.9982943574932,71.8652771155594));
#39276=CARTESIAN_POINT('Ctrl Pts',(3.57214502087136,-16.9982640274543,71.8658958651526));
#39277=CARTESIAN_POINT('Ctrl Pts',(3.57273209133846,-16.9982357585976,71.8664725654874));
#39278=CARTESIAN_POINT('Ctrl Pts',(3.57320299278071,-16.9982127623775,71.8669354348749));
#39279=CARTESIAN_POINT('Ctrl Pts',(3.57360188999624,-16.9981931657129,71.867327729259));
#39280=CARTESIAN_POINT('Ctrl Pts',(3.57394979081275,-16.9981760743537,71.8676698713729));
#39281=CARTESIAN_POINT('Ctrl Pts',(3.57424318974082,-16.9981615513357,71.8679585937125));
#39282=CARTESIAN_POINT('Ctrl Pts',(3.57453458878626,-16.9981470538884,71.8682453580158));
#39283=CARTESIAN_POINT('',(2.86824535801579,-16.9981470538884,72.5745345887863));
#39284=CARTESIAN_POINT('Ctrl Pts',(2.86824535801579,-16.9981470538884,72.5745345887863));
#39285=CARTESIAN_POINT('Ctrl Pts',(3.10367510160595,-16.9981470538884,72.3391048451961));
#39286=CARTESIAN_POINT('Ctrl Pts',(3.3391048451961,-16.9981470538884,72.1036751016059));
#39287=CARTESIAN_POINT('Ctrl Pts',(3.57453458878626,-16.9981470538884,71.8682453580158));
#39288=CARTESIAN_POINT('',(2.79531863640927,-17.,72.5));
#39289=CARTESIAN_POINT('Ctrl Pts',(2.86824535801579,-16.9981470538884,72.5745345887863));
#39290=CARTESIAN_POINT('Ctrl Pts',(2.86792051198431,-16.9981634765679,72.5742044925281));
#39291=CARTESIAN_POINT('Ctrl Pts',(2.86759246756107,-16.9981799708645,72.5738711310018));
#39292=CARTESIAN_POINT('Ctrl Pts',(2.86718860352498,-16.9982001093812,72.57346041281));
#39293=CARTESIAN_POINT('Ctrl Pts',(2.86676473939109,-16.9982212451946,72.57302935509));
#39294=CARTESIAN_POINT('Ctrl Pts',(2.86625756382415,-16.9982463879926,72.5725132968389));
#39295=CARTESIAN_POINT('Ctrl Pts',(2.86562376912052,-16.9982773404549,72.5718680115171));
#39296=CARTESIAN_POINT('Ctrl Pts',(2.86494852089771,-16.9983103173716,72.5711805211291));
#39297=CARTESIAN_POINT('Ctrl Pts',(2.86412982782487,-16.9983498713227,72.5703466306137));
#39298=CARTESIAN_POINT('Ctrl Pts',(2.86315671761944,-16.9983957676602,72.5693550535868));
#39299=CARTESIAN_POINT('Ctrl Pts',(2.86208246075231,-16.9984464345378,72.5682604104266));
#39300=CARTESIAN_POINT('Ctrl Pts',(2.86082042406595,-16.9985047829815,72.5669740091159));
#39301=CARTESIAN_POINT('Ctrl Pts',(2.85939970674287,-16.9985681244217,72.565525387959));
#39302=CARTESIAN_POINT('Ctrl Pts',(2.85761705827722,-16.9986476022457,72.5637077270911));
#39303=CARTESIAN_POINT('Ctrl Pts',(2.85558546640715,-16.9987347812318,72.5616355608823));
#39304=CARTESIAN_POINT('Ctrl Pts',(2.85342062894716,-16.9988223610841,72.5594266767905));
#39305=CARTESIAN_POINT('Ctrl Pts',(2.85112488425854,-16.9989152368701,72.5570842219804));
#39306=CARTESIAN_POINT('Ctrl Pts',(2.84868403352371,-16.9990082804756,72.5545928471897));
#39307=CARTESIAN_POINT('Ctrl Pts',(2.84624625175195,-16.9990947989236,72.552103587594));
#39308=CARTESIAN_POINT('Ctrl Pts',(2.84439897927724,-16.9991603598156,72.5502173068831));
#39309=CARTESIAN_POINT('Ctrl Pts',(2.84255427195848,-16.9992222334679,72.5483330647398));
#39310=CARTESIAN_POINT('Ctrl Pts',(2.84075306394266,-16.9992793054386,72.5464926261216));
#39311=CARTESIAN_POINT('Ctrl Pts',(2.83912769582928,-16.9993308058541,72.5448318572274));
#39312=CARTESIAN_POINT('Ctrl Pts',(2.83753815081149,-16.9993784253393,72.543207168852));
#39313=CARTESIAN_POINT('Ctrl Pts',(2.83598557864455,-16.9994224873957,72.5416197584348));
#39314=CARTESIAN_POINT('Ctrl Pts',(2.83445351746977,-16.9994659673493,72.540053319257));
#39315=CARTESIAN_POINT('Ctrl Pts',(2.83295811821705,-16.9995060035546,72.5385238533706));
#39316=CARTESIAN_POINT('Ctrl Pts',(2.83146270058428,-16.9995437460623,72.5369939676884));
#39317=CARTESIAN_POINT('Ctrl Pts',(2.83000471420189,-16.9995805438512,72.5355023760137));
#39318=CARTESIAN_POINT('Ctrl Pts',(2.82854016663104,-16.9996153196962,72.5340037037557));
#39319=CARTESIAN_POINT('Ctrl Pts',(2.82703981578638,-16.9996485645807,72.5324681805947));
#39320=CARTESIAN_POINT('Ctrl Pts',(2.82542721104074,-16.9996842967954,72.5308177719951));
#39321=CARTESIAN_POINT('Ctrl Pts',(2.82377359513262,-16.9997182120423,72.529125149268));
#39322=CARTESIAN_POINT('Ctrl Pts',(2.82208470500296,-16.9997497930326,72.5273963190708));
#39323=CARTESIAN_POINT('Ctrl Pts',(2.82015515581749,-16.9997858741684,72.5254211385424));
#39324=CARTESIAN_POINT('Ctrl Pts',(2.81818008615893,-16.9998188305302,72.5233992312896));
#39325=CARTESIAN_POINT('Ctrl Pts',(2.81621482751817,-16.9998475191546,72.52138736276));
#39326=CARTESIAN_POINT('Ctrl Pts',(2.81349256857323,-16.9998872583841,72.5186005402078));
#39327=CARTESIAN_POINT('Ctrl Pts',(2.81079201806523,-16.9999185308537,72.5158359360068));
#39328=CARTESIAN_POINT('Ctrl Pts',(2.80832539114039,-16.9999409383933,72.5133109478137));
#39329=CARTESIAN_POINT('Ctrl Pts',(2.80647542094676,-16.9999577440481,72.5114172066689));
#39330=CARTESIAN_POINT('Ctrl Pts',(2.80475967567115,-16.9999696816405,72.5096609508553));
#39331=CARTESIAN_POINT('Ctrl Pts',(2.80325251525599,-16.9999780308564,72.508118309431));
#39332=CARTESIAN_POINT('Ctrl Pts',(2.80198975715482,-16.999985026157,72.5068258239488));
#39333=CARTESIAN_POINT('Ctrl Pts',(2.80087378577512,-16.9999895478102,72.5056836631397));
#39334=CARTESIAN_POINT('Ctrl Pts',(2.79992260032023,-16.9999926045357,72.5047102375997));
#39335=CARTESIAN_POINT('Ctrl Pts',(2.79902830376709,-16.9999954784432,72.5037950311059));
#39336=CARTESIAN_POINT('Ctrl Pts',(2.79828008131994,-16.9999970739683,72.5030293988184));
#39337=CARTESIAN_POINT('Ctrl Pts',(2.79766257486899,-16.9999980838367,72.5023976001144));
#39338=CARTESIAN_POINT('Ctrl Pts',(2.79708702610116,-16.9999990250876,72.5018087302087));
#39339=CARTESIAN_POINT('Ctrl Pts',(2.79662518068281,-16.9999994582021,72.5013362750362));
#39340=CARTESIAN_POINT('Ctrl Pts',(2.79623381941522,-16.9999997079814,72.500935978419));
#39341=CARTESIAN_POINT('Ctrl Pts',(2.79589255313753,-16.9999999257886,72.5005869205336));
#39342=CARTESIAN_POINT('Ctrl Pts',(2.79560461778332,-17.,72.5002924603909));
#39343=CARTESIAN_POINT('Ctrl Pts',(2.79531863640927,-17.,72.5));
#39344=CARTESIAN_POINT('',(3.14765931820464,-17.,72.1476593182046));
#39345=CARTESIAN_POINT('Ctrl Pts',(2.86824535801579,-16.9981470538884,72.5745345887863));
#39346=CARTESIAN_POINT('Ctrl Pts',(3.24643975969903,-16.9790273330526,72.9588414442702));
#39347=CARTESIAN_POINT('Ctrl Pts',(3.89283858086126,-16.6911512202391,73.5507380181503));
#39348=CARTESIAN_POINT('Ctrl Pts',(4.42126461973579,-16.0144112572066,73.9509340499422));
#39349=CARTESIAN_POINT('Ctrl Pts',(4.5,-15.6672482052684,74.));
#39350=CARTESIAN_POINT('Ctrl Pts',(4.5,-15.5,74.));
#39351=CARTESIAN_POINT('Ctrl Pts',(3.10367510160595,-16.9981470538884,72.3391048451961));
#39352=CARTESIAN_POINT('Ctrl Pts',(3.48390698788943,-16.9790273330526,72.7213742160798));
#39353=CARTESIAN_POINT('Ctrl Pts',(4.11213839329095,-16.6911512202391,73.3314382057206));
#39354=CARTESIAN_POINT('Ctrl Pts',(4.59782109647126,-16.0144112572066,73.7743775732067));
#39355=CARTESIAN_POINT('Ctrl Pts',(4.66666666666667,-15.6672482052684,73.8333333333333));
#39356=CARTESIAN_POINT('Ctrl Pts',(4.66666666666667,-15.5,73.8333333333333));
#39357=CARTESIAN_POINT('Ctrl Pts',(3.3391048451961,-16.9981470538884,72.1036751016059));
#39358=CARTESIAN_POINT('Ctrl Pts',(3.72137421607983,-16.9790273330526,72.4839069878894));
#39359=CARTESIAN_POINT('Ctrl Pts',(4.33143820572063,-16.6911512202391,73.112138393291));
#39360=CARTESIAN_POINT('Ctrl Pts',(4.77437757320674,-16.0144112572066,73.5978210964713));
#39361=CARTESIAN_POINT('Ctrl Pts',(4.83333333333334,-15.6672482052684,73.6666666666667));
#39362=CARTESIAN_POINT('Ctrl Pts',(4.83333333333334,-15.5,73.6666666666667));
#39363=CARTESIAN_POINT('Ctrl Pts',(3.57453458878626,-16.9981470538884,71.8682453580158));
#39364=CARTESIAN_POINT('Ctrl Pts',(3.95884144427024,-16.9790273330526,72.246439759699));
#39365=CARTESIAN_POINT('Ctrl Pts',(4.55073801815032,-16.6911512202391,72.8928385808613));
#39366=CARTESIAN_POINT('Ctrl Pts',(4.95093404994221,-16.0144112572066,73.4212646197358));
#39367=CARTESIAN_POINT('Ctrl Pts',(5.,-15.6672482052684,73.5));
#39368=CARTESIAN_POINT('Ctrl Pts',(5.,-15.5,73.5));
#39369=CARTESIAN_POINT('',(5.,-15.5,73.5));
#39370=CARTESIAN_POINT('Ctrl Pts',(3.57453458878626,-16.9981470538884,71.8682453580158));
#39371=CARTESIAN_POINT('Ctrl Pts',(3.95884144427024,-16.9790273330526,72.246439759699));
#39372=CARTESIAN_POINT('Ctrl Pts',(4.55073801815032,-16.6911512202391,72.8928385808613));
#39373=CARTESIAN_POINT('Ctrl Pts',(4.95093404994221,-16.0144112572066,73.4212646197358));
#39374=CARTESIAN_POINT('Ctrl Pts',(5.,-15.6672482052684,73.5));
#39375=CARTESIAN_POINT('Ctrl Pts',(5.,-15.5,73.5));
#39376=CARTESIAN_POINT('',(4.5,-15.5,74.));
#39377=CARTESIAN_POINT('',(5.,-15.5,73.5));
#39378=CARTESIAN_POINT('Ctrl Pts',(4.5,-15.5,74.));
#39379=CARTESIAN_POINT('Ctrl Pts',(4.5,-15.6672482052684,74.));
#39380=CARTESIAN_POINT('Ctrl Pts',(4.42126461973579,-16.0144112572066,73.9509340499422));
#39381=CARTESIAN_POINT('Ctrl Pts',(3.89283858086126,-16.6911512202391,73.5507380181503));
#39382=CARTESIAN_POINT('Ctrl Pts',(3.24643975969903,-16.9790273330526,72.9588414442702));
#39383=CARTESIAN_POINT('Ctrl Pts',(2.86824535801579,-16.9981470538884,72.5745345887863));
#39384=CARTESIAN_POINT('Origin',(4.75,-14.,73.75));
#39385=CARTESIAN_POINT('',(5.,-14.,73.5));
#39386=CARTESIAN_POINT('',(4.5,-14.,74.));
#39387=CARTESIAN_POINT('',(-0.750000000000002,-14.,79.25));
#39388=CARTESIAN_POINT('',(4.5,-14.,74.));
#39389=CARTESIAN_POINT('',(5.,-14.,73.5));
#39390=CARTESIAN_POINT('Origin',(3.33066907387547E-15,-17.,62.));
#39391=CARTESIAN_POINT('',(-2.79531863640926,-17.,72.5));
#39392=CARTESIAN_POINT('',(2.5,-17.,72.5));
#39393=CARTESIAN_POINT('',(-3.5,-17.,71.7953186364093));
#39394=CARTESIAN_POINT('',(-3.14765931820463,-17.,72.1476593182046));
#39395=CARTESIAN_POINT('',(-3.5,-17.,56.3914887194867));
#39396=CARTESIAN_POINT('',(-3.5,-17.,68.));
#39397=CARTESIAN_POINT('',(3.5,-17.,56.3914887194867));
#39398=CARTESIAN_POINT('Origin',(0.,-17.,0.));
#39399=CARTESIAN_POINT('',(3.5,-17.,56.));
#39400=CARTESIAN_POINT('Origin',(2.5,-15.5,72.5));
#39401=CARTESIAN_POINT('',(-4.5,-15.5,74.));
#39402=CARTESIAN_POINT('',(2.5,-15.5,74.));
#39403=CARTESIAN_POINT('',(-2.86824535801578,-16.9981470538884,72.5745345887862));
#39404=CARTESIAN_POINT('Ctrl Pts',(-2.86824535801578,-16.9981470538884,
72.5745345887862));
#39405=CARTESIAN_POINT('Ctrl Pts',(-3.24643975969902,-16.9790273330526,
72.9588414442702));
#39406=CARTESIAN_POINT('Ctrl Pts',(-3.89283858086125,-16.6911512202391,
73.5507380181503));
#39407=CARTESIAN_POINT('Ctrl Pts',(-4.42126461973579,-16.0144112572066,
73.9509340499422));
#39408=CARTESIAN_POINT('Ctrl Pts',(-4.5,-15.6672482052684,74.));
#39409=CARTESIAN_POINT('Ctrl Pts',(-4.5,-15.5,74.));
#39410=CARTESIAN_POINT('Ctrl Pts',(-2.79531863640926,-17.,72.5));
#39411=CARTESIAN_POINT('Ctrl Pts',(-2.79564265664126,-17.,72.5003313610337));
#39412=CARTESIAN_POINT('Ctrl Pts',(-2.79596987101048,-16.9999999087783,
72.5006659910395));
#39413=CARTESIAN_POINT('Ctrl Pts',(-2.79637281953386,-16.9999996125274,
72.5010781547591));
#39414=CARTESIAN_POINT('Ctrl Pts',(-2.7967957210522,-16.9999993016069,72.501510727787));
#39415=CARTESIAN_POINT('Ctrl Pts',(-2.79730183940143,-16.999998768055,72.5020284953742));
#39416=CARTESIAN_POINT('Ctrl Pts',(-2.79793444218738,-16.9999976134245,
72.502675765448));
#39417=CARTESIAN_POINT('Ctrl Pts',(-2.79860841572207,-16.9999963832839,
72.5033653654769));
#39418=CARTESIAN_POINT('Ctrl Pts',(-2.79942567946863,-16.9999944448324,
72.5042016754148));
#39419=CARTESIAN_POINT('Ctrl Pts',(-2.80039721343957,-16.9999910006556,
72.5051959553729));
#39420=CARTESIAN_POINT('Ctrl Pts',(-2.8014697058444,-16.9999871985718,72.5062935574489));
#39421=CARTESIAN_POINT('Ctrl Pts',(-2.80272979087921,-16.9999815341953,
72.5075832522893));
#39422=CARTESIAN_POINT('Ctrl Pts',(-2.80414844370905,-16.9999727872824,
72.509035342403));
#39423=CARTESIAN_POINT('Ctrl Pts',(-2.80592829490881,-16.9999618133477,
72.5108571442398));
#39424=CARTESIAN_POINT('Ctrl Pts',(-2.80795685459662,-16.9999458718544,
72.5129336615423));
#39425=CARTESIAN_POINT('Ctrl Pts',(-2.81011870232467,-16.9999235237508,
72.5151467124795));
#39426=CARTESIAN_POINT('Ctrl Pts',(-2.81241216138654,-16.9998998151149,
72.5174944919555));
#39427=CARTESIAN_POINT('Ctrl Pts',(-2.81485089376864,-16.9998688531822,
72.5199910876103));
#39428=CARTESIAN_POINT('Ctrl Pts',(-2.81728690624045,-16.9998314674613,
72.522484866309));
#39429=CARTESIAN_POINT('Ctrl Pts',(-2.81913249915804,-16.9998031429668,
72.524374224577));
#39430=CARTESIAN_POINT('Ctrl Pts',(-2.82097572933093,-16.9997712320714,
72.5262611440487));
#39431=CARTESIAN_POINT('Ctrl Pts',(-2.82277575793103,-16.9997367040829,
72.5281037084108));
#39432=CARTESIAN_POINT('Ctrl Pts',(-2.82440003690208,-16.9997055473083,
72.5297663700741));
#39433=CARTESIAN_POINT('Ctrl Pts',(-2.82598873685543,-16.9996723091153,
72.531392504458));
#39434=CARTESIAN_POINT('Ctrl Pts',(-2.82754075055383,-16.9996373773349,
72.5329808505079));
#39435=CARTESIAN_POINT('Ctrl Pts',(-2.82907180232415,-16.9996029173527,
72.5345477439148));
#39436=CARTESIAN_POINT('Ctrl Pts',(-2.83056649572128,-16.9995668629652,
72.5360771924232));
#39437=CARTESIAN_POINT('Ctrl Pts',(-2.83206147390568,-16.9995285090951,
72.5376065208571));
#39438=CARTESIAN_POINT('Ctrl Pts',(-2.83351949589972,-16.9994911033411,
72.5390980439549));
#39439=CARTESIAN_POINT('Ctrl Pts',(-2.83498433344674,-16.9994513364011,
72.5405961355826));
#39440=CARTESIAN_POINT('Ctrl Pts',(-2.83648523260947,-16.9994082206029,
72.5421306063153));
#39441=CARTESIAN_POINT('Ctrl Pts',(-2.83809840088706,-16.9993618796896,
72.5437798573578));
#39442=CARTESIAN_POINT('Ctrl Pts',(-2.83975287701613,-16.9993116397098,
72.5454707747875));
#39443=CARTESIAN_POINT('Ctrl Pts',(-2.84144288479758,-16.9992572833264,
72.5471974405305));
#39444=CARTESIAN_POINT('Ctrl Pts',(-2.84337359161561,-16.9991951852455,
72.5491700263133));
#39445=CARTESIAN_POINT('Ctrl Pts',(-2.84535014849355,-16.9991276636876,
72.5511887316101));
#39446=CARTESIAN_POINT('Ctrl Pts',(-2.84731712868052,-16.9990563957717,
72.5531970139765));
#39447=CARTESIAN_POINT('Ctrl Pts',(-2.85004228373109,-16.9989576575525,
72.5559793911808));
#39448=CARTESIAN_POINT('Ctrl Pts',(-2.85274617133165,-16.9988515979041,
72.5587388045197));
#39449=CARTESIAN_POINT('Ctrl Pts',(-2.85521613868755,-16.9987486082515,
72.5612585444167));
#39450=CARTESIAN_POINT('Ctrl Pts',(-2.85706861420448,-16.9986713660121,
72.5631483493395));
#39451=CARTESIAN_POINT('Ctrl Pts',(-2.85878686230645,-16.998596102758,72.5649006457068));
#39452=CARTESIAN_POINT('Ctrl Pts',(-2.86029635854139,-16.9985278711001,
72.5664395931371));
#39453=CARTESIAN_POINT('Ctrl Pts',(-2.86156104371884,-16.9984707052957,
72.5677289530964));
#39454=CARTESIAN_POINT('Ctrl Pts',(-2.86267883139743,-16.9984185388897,
72.5688681843539));
#39455=CARTESIAN_POINT('Ctrl Pts',(-2.86363166532158,-16.998373289921,72.5698389866149));
#39456=CARTESIAN_POINT('Ctrl Pts',(-2.86452750002013,-16.9983307477788,
72.5707517147711));
#39457=CARTESIAN_POINT('Ctrl Pts',(-2.86527711555935,-16.9982943574932,
72.5715151450229));
#39458=CARTESIAN_POINT('Ctrl Pts',(-2.86589586515256,-16.9982640274543,
72.5721450208714));
#39459=CARTESIAN_POINT('Ctrl Pts',(-2.86647256548742,-16.9982357585976,
72.5727320913385));
#39460=CARTESIAN_POINT('Ctrl Pts',(-2.86693543487487,-16.9982127623775,
72.5732029927807));
#39461=CARTESIAN_POINT('Ctrl Pts',(-2.86732772925898,-16.9981931657129,
72.5736018899962));
#39462=CARTESIAN_POINT('Ctrl Pts',(-2.86766987137286,-16.9981760743537,
72.5739497908127));
#39463=CARTESIAN_POINT('Ctrl Pts',(-2.86795859371255,-16.9981615513357,
72.5742431897408));
#39464=CARTESIAN_POINT('Ctrl Pts',(-2.86824535801578,-16.9981470538884,
72.5745345887862));
#39465=CARTESIAN_POINT('Origin',(5.,-14.,74.));
#39466=CARTESIAN_POINT('',(-4.49999999999999,-14.,74.));
#39467=CARTESIAN_POINT('',(2.5,-14.,74.));
#39468=CARTESIAN_POINT('',(-4.49999999999999,-14.,74.));
#39469=CARTESIAN_POINT('Ctrl Pts',(-2.86824535801578,-16.9981470538884,
72.5745345887862));
#39470=CARTESIAN_POINT('Ctrl Pts',(-2.86416335850594,-16.9983534204838,
72.5703866151813));
#39471=CARTESIAN_POINT('Ctrl Pts',(-2.834280745957,-16.9997799301677,72.5399078658621));
#39472=CARTESIAN_POINT('Ctrl Pts',(-2.80161322910155,-16.9999870327594,
72.5064297689792));
#39473=CARTESIAN_POINT('Ctrl Pts',(-2.79633659788021,-17.,72.5010410237755));
#39474=CARTESIAN_POINT('Ctrl Pts',(-2.79531863640926,-17.,72.5));
#39475=CARTESIAN_POINT('Ctrl Pts',(-3.10367510160593,-16.9981470538884,
72.3391048451961));
#39476=CARTESIAN_POINT('Ctrl Pts',(-3.09957111073106,-16.9983534204838,
72.3349788629562));
#39477=CARTESIAN_POINT('Ctrl Pts',(-3.06945705860968,-16.9997799301677,
72.3047315532094));
#39478=CARTESIAN_POINT('Ctrl Pts',(-3.0365616348729,-16.9999870327594,72.2714813632078));
#39479=CARTESIAN_POINT('Ctrl Pts',(-3.03123807317865,-17.,72.2661395484771));
#39480=CARTESIAN_POINT('Ctrl Pts',(-3.03021242427284,-17.,72.2651062121364));
#39481=CARTESIAN_POINT('Ctrl Pts',(-3.33910484519609,-16.9981470538884,
72.1036751016059));
#39482=CARTESIAN_POINT('Ctrl Pts',(-3.33497886295619,-16.9983534204838,
72.0995711107311));
#39483=CARTESIAN_POINT('Ctrl Pts',(-3.30455472555143,-17.0000242835561,
72.0694570586097));
#39484=CARTESIAN_POINT('Ctrl Pts',(-3.27145680316828,-16.9998354184739,
72.0365616348729));
#39485=CARTESIAN_POINT('Ctrl Pts',(-3.26613954847708,-17.,72.0312380731786));
#39486=CARTESIAN_POINT('Ctrl Pts',(-3.26510621213642,-17.,72.0302124242728));
#39487=CARTESIAN_POINT('Ctrl Pts',(-3.57453458878625,-16.9981470538884,
71.8682453580158));
#39488=CARTESIAN_POINT('Ctrl Pts',(-3.57038661518132,-16.9983534204838,
71.8641633585059));
#39489=CARTESIAN_POINT('Ctrl Pts',(-3.53990786586207,-16.9997799301677,
71.834280745957));
#39490=CARTESIAN_POINT('Ctrl Pts',(-3.5064297689792,-16.9999870327594,71.8016132291015));
#39491=CARTESIAN_POINT('Ctrl Pts',(-3.50104102377551,-17.,71.7963365978802));
#39492=CARTESIAN_POINT('Ctrl Pts',(-3.5,-17.,71.7953186364093));
#39493=CARTESIAN_POINT('',(-3.57453458878625,-16.9981470538884,71.8682453580158));
#39494=CARTESIAN_POINT('Ctrl Pts',(-3.57453458878625,-16.9981470538884,
71.8682453580158));
#39495=CARTESIAN_POINT('Ctrl Pts',(-3.33910484519609,-16.9981470538884,
72.1036751016059));
#39496=CARTESIAN_POINT('Ctrl Pts',(-3.10367510160593,-16.9981470538884,
72.3391048451961));
#39497=CARTESIAN_POINT('Ctrl Pts',(-2.86824535801578,-16.9981470538884,
72.5745345887862));
#39498=CARTESIAN_POINT('Ctrl Pts',(-3.57453458878625,-16.9981470538884,
71.8682453580158));
#39499=CARTESIAN_POINT('Ctrl Pts',(-3.57420449252803,-16.9981634765679,
71.8679205119843));
#39500=CARTESIAN_POINT('Ctrl Pts',(-3.57387113100174,-16.9981799708645,
71.8675924675611));
#39501=CARTESIAN_POINT('Ctrl Pts',(-3.57346041281003,-16.9982001093812,
71.867188603525));
#39502=CARTESIAN_POINT('Ctrl Pts',(-3.57302935509,-16.9982212451947,71.8667647393911));
#39503=CARTESIAN_POINT('Ctrl Pts',(-3.57251329683894,-16.9982463879926,
71.8662575638241));
#39504=CARTESIAN_POINT('Ctrl Pts',(-3.57186801151713,-16.9982773404549,
71.8656237691205));
#39505=CARTESIAN_POINT('Ctrl Pts',(-3.57118052112907,-16.9983103173716,
71.8649485208977));
#39506=CARTESIAN_POINT('Ctrl Pts',(-3.57034663061369,-16.9983498713227,
71.8641298278249));
#39507=CARTESIAN_POINT('Ctrl Pts',(-3.56935505358675,-16.9983957676602,
71.8631567176194));
#39508=CARTESIAN_POINT('Ctrl Pts',(-3.56826041042659,-16.9984464345378,
71.8620824607523));
#39509=CARTESIAN_POINT('Ctrl Pts',(-3.56697400911585,-16.9985047829815,
71.8608204240659));
#39510=CARTESIAN_POINT('Ctrl Pts',(-3.56552538795899,-16.9985681244217,
71.8593997067428));
#39511=CARTESIAN_POINT('Ctrl Pts',(-3.56370772709106,-16.9986476022457,
71.8576170582772));
#39512=CARTESIAN_POINT('Ctrl Pts',(-3.56163556088227,-16.9987347812318,
71.8555854664071));
#39513=CARTESIAN_POINT('Ctrl Pts',(-3.55942667679054,-16.9988223610841,
71.8534206289472));
#39514=CARTESIAN_POINT('Ctrl Pts',(-3.55708422198037,-16.9989152368701,
71.8511248842585));
#39515=CARTESIAN_POINT('Ctrl Pts',(-3.55459284718975,-16.9990082804756,
71.8486840335237));
#39516=CARTESIAN_POINT('Ctrl Pts',(-3.55210358759403,-16.9990947989236,
71.8462462517519));
#39517=CARTESIAN_POINT('Ctrl Pts',(-3.55021730688309,-16.9991603598156,
71.8443989792772));
#39518=CARTESIAN_POINT('Ctrl Pts',(-3.54833306473982,-16.9992222334679,
71.8425542719585));
#39519=CARTESIAN_POINT('Ctrl Pts',(-3.54649262612163,-16.9992793054386,
71.8407530639427));
#39520=CARTESIAN_POINT('Ctrl Pts',(-3.54483185722744,-16.9993308058541,
71.8391276958293));
#39521=CARTESIAN_POINT('Ctrl Pts',(-3.543207168852,-16.9993784253393,71.8375381508115));
#39522=CARTESIAN_POINT('Ctrl Pts',(-3.5416197584348,-16.9994224873957,71.8359855786445));
#39523=CARTESIAN_POINT('Ctrl Pts',(-3.54005331925703,-16.9994659673493,
71.8344535174698));
#39524=CARTESIAN_POINT('Ctrl Pts',(-3.53852385337057,-16.9995060035546,
71.8329581182171));
#39525=CARTESIAN_POINT('Ctrl Pts',(-3.53699396768837,-16.9995437460623,
71.8314627005843));
#39526=CARTESIAN_POINT('Ctrl Pts',(-3.53550237601366,-16.9995805438512,
71.8300047142019));
#39527=CARTESIAN_POINT('Ctrl Pts',(-3.53400370375571,-16.9996153196962,
71.828540166631));
#39528=CARTESIAN_POINT('Ctrl Pts',(-3.5324681805947,-16.9996485645807,71.8270398157864));
#39529=CARTESIAN_POINT('Ctrl Pts',(-3.53081777199506,-16.9996842967954,
71.8254272110407));
#39530=CARTESIAN_POINT('Ctrl Pts',(-3.529125149268,-16.9997182120423,71.8237735951326));
#39531=CARTESIAN_POINT('Ctrl Pts',(-3.52739631907081,-16.9997497930326,
71.8220847050029));
#39532=CARTESIAN_POINT('Ctrl Pts',(-3.52542113854234,-16.9997858741684,
71.8201551558175));
#39533=CARTESIAN_POINT('Ctrl Pts',(-3.52339923128959,-16.9998188305302,
71.8181800861589));
#39534=CARTESIAN_POINT('Ctrl Pts',(-3.52138736275996,-16.9998475191546,
71.8162148275182));
#39535=CARTESIAN_POINT('Ctrl Pts',(-3.51860054020783,-16.9998872583841,
71.8134925685732));
#39536=CARTESIAN_POINT('Ctrl Pts',(-3.51583593600677,-16.9999185308537,
71.8107920180652));
#39537=CARTESIAN_POINT('Ctrl Pts',(-3.51331094781369,-16.9999409383933,
71.8083253911404));
#39538=CARTESIAN_POINT('Ctrl Pts',(-3.51141720666888,-16.9999577440481,
71.8064754209467));
#39539=CARTESIAN_POINT('Ctrl Pts',(-3.50966095085531,-16.9999696816405,
71.8047596756711));
#39540=CARTESIAN_POINT('Ctrl Pts',(-3.50811830943095,-16.9999780308564,
71.803252515256));
#39541=CARTESIAN_POINT('Ctrl Pts',(-3.50682582394883,-16.999985026157,71.8019897571548));
#39542=CARTESIAN_POINT('Ctrl Pts',(-3.50568366313966,-16.9999895478102,
71.8008737857751));
#39543=CARTESIAN_POINT('Ctrl Pts',(-3.50471023759971,-16.9999926045357,
71.7999226003202));
#39544=CARTESIAN_POINT('Ctrl Pts',(-3.50379503110591,-16.9999954784432,
71.7990283037671));
#39545=CARTESIAN_POINT('Ctrl Pts',(-3.50302939881839,-16.9999970739683,
71.7982800813199));
#39546=CARTESIAN_POINT('Ctrl Pts',(-3.50239760011444,-16.9999980838367,
71.797662574869));
#39547=CARTESIAN_POINT('Ctrl Pts',(-3.50180873020869,-16.9999990250876,
71.7970870261012));
#39548=CARTESIAN_POINT('Ctrl Pts',(-3.50133627503614,-16.9999994582021,
71.7966251806828));
#39549=CARTESIAN_POINT('Ctrl Pts',(-3.50093597841901,-16.9999997079814,
71.7962338194152));
#39550=CARTESIAN_POINT('Ctrl Pts',(-3.5005869205336,-16.9999999257886,71.7958925531375));
#39551=CARTESIAN_POINT('Ctrl Pts',(-3.50029246039092,-17.,71.7956046177833));
#39552=CARTESIAN_POINT('Ctrl Pts',(-3.5,-17.,71.7953186364093));
#39553=CARTESIAN_POINT('Ctrl Pts',(-3.57453458878625,-16.9981470538884,
71.8682453580158));
#39554=CARTESIAN_POINT('Ctrl Pts',(-3.95884144427023,-16.9790273330526,
72.246439759699));
#39555=CARTESIAN_POINT('Ctrl Pts',(-4.55073801815031,-16.6911512202391,
72.8928385808613));
#39556=CARTESIAN_POINT('Ctrl Pts',(-4.95093404994219,-16.0144112572066,
73.4212646197358));
#39557=CARTESIAN_POINT('Ctrl Pts',(-4.99999999999999,-15.6672482052684,
73.5));
#39558=CARTESIAN_POINT('Ctrl Pts',(-4.99999999999999,-15.5,73.5));
#39559=CARTESIAN_POINT('Ctrl Pts',(-3.33910484519609,-16.9981470538884,
72.1036751016059));
#39560=CARTESIAN_POINT('Ctrl Pts',(-3.72137421607982,-16.9790273330526,
72.4839069878894));
#39561=CARTESIAN_POINT('Ctrl Pts',(-4.33143820572062,-16.6911512202391,
73.1121383932909));
#39562=CARTESIAN_POINT('Ctrl Pts',(-4.77437757320673,-16.0144112572066,
73.5978210964712));
#39563=CARTESIAN_POINT('Ctrl Pts',(-4.83333333333333,-15.6672482052684,
73.6666666666667));
#39564=CARTESIAN_POINT('Ctrl Pts',(-4.83333333333333,-15.5,73.6666666666667));
#39565=CARTESIAN_POINT('Ctrl Pts',(-3.10367510160593,-16.9981470538884,
72.3391048451961));
#39566=CARTESIAN_POINT('Ctrl Pts',(-3.48390698788942,-16.9790273330526,
72.7213742160798));
#39567=CARTESIAN_POINT('Ctrl Pts',(-4.11213839329094,-16.6911512202391,
73.3314382057206));
#39568=CARTESIAN_POINT('Ctrl Pts',(-4.59782109647126,-16.0144112572066,
73.7743775732067));
#39569=CARTESIAN_POINT('Ctrl Pts',(-4.66666666666666,-15.6672482052684,
73.8333333333333));
#39570=CARTESIAN_POINT('Ctrl Pts',(-4.66666666666666,-15.5,73.8333333333333));
#39571=CARTESIAN_POINT('Ctrl Pts',(-2.86824535801578,-16.9981470538884,
72.5745345887862));
#39572=CARTESIAN_POINT('Ctrl Pts',(-3.24643975969902,-16.9790273330526,
72.9588414442702));
#39573=CARTESIAN_POINT('Ctrl Pts',(-3.89283858086125,-16.6911512202391,
73.5507380181503));
#39574=CARTESIAN_POINT('Ctrl Pts',(-4.42126461973579,-16.0144112572066,
73.9509340499422));
#39575=CARTESIAN_POINT('Ctrl Pts',(-4.5,-15.6672482052684,74.));
#39576=CARTESIAN_POINT('Ctrl Pts',(-4.5,-15.5,74.));
#39577=CARTESIAN_POINT('',(-4.99999999999999,-15.5,73.5));
#39578=CARTESIAN_POINT('',(-4.5,-15.5,74.));
#39579=CARTESIAN_POINT('Ctrl Pts',(-4.99999999999999,-15.5,73.5));
#39580=CARTESIAN_POINT('Ctrl Pts',(-4.99999999999999,-15.6672482052684,
73.5));
#39581=CARTESIAN_POINT('Ctrl Pts',(-4.95093404994219,-16.0144112572066,
73.4212646197358));
#39582=CARTESIAN_POINT('Ctrl Pts',(-4.55073801815031,-16.6911512202391,
72.8928385808613));
#39583=CARTESIAN_POINT('Ctrl Pts',(-3.95884144427023,-16.9790273330526,
72.246439759699));
#39584=CARTESIAN_POINT('Ctrl Pts',(-3.57453458878625,-16.9981470538884,
71.8682453580158));
#39585=CARTESIAN_POINT('Origin',(-4.75,-14.,73.75));
#39586=CARTESIAN_POINT('',(-5.,-14.,73.5));
#39587=CARTESIAN_POINT('',(0.749999999999987,-14.,79.2500000000001));
#39588=CARTESIAN_POINT('',(-5.,-14.,73.5));
#39589=CARTESIAN_POINT('Origin',(-3.5,-15.5,68.));
#39590=CARTESIAN_POINT('',(-5.,-15.5,56.2783262011229));
#39591=CARTESIAN_POINT('',(-5.,-15.5,68.));
#39592=CARTESIAN_POINT('Ctrl Pts',(-3.49999999999999,-17.,56.3914887194867));
#39593=CARTESIAN_POINT('Ctrl Pts',(-3.68849285843232,-17.,56.379789702144));
#39594=CARTESIAN_POINT('Ctrl Pts',(-3.88949595769794,-16.9623071985392,
56.366268079425));
#39595=CARTESIAN_POINT('Ctrl Pts',(-4.25923828551908,-16.8090480003591,
56.3395353657988));
#39596=CARTESIAN_POINT('Ctrl Pts',(-4.42798167302478,-16.6934822832211,
56.3263779287031));
#39597=CARTESIAN_POINT('Ctrl Pts',(-4.69412389350913,-16.4270526075957,
56.3048219679644));
#39598=CARTESIAN_POINT('Ctrl Pts',(-4.80941523738749,-16.2585410496607,
56.2949857165266));
#39599=CARTESIAN_POINT('Ctrl Pts',(-4.96235566707568,-15.889189778178,56.2817103328366));
#39600=CARTESIAN_POINT('Ctrl Pts',(-5.,-15.6883461217826,56.2783262011229));
#39601=CARTESIAN_POINT('Ctrl Pts',(-5.,-15.5,56.2783262011229));
#39602=CARTESIAN_POINT('Origin',(-5.,-14.,74.));
#39603=CARTESIAN_POINT('',(-5.,-14.,56.2783262011229));
#39604=CARTESIAN_POINT('',(-4.99999999999999,-14.,82.5));
#39605=CARTESIAN_POINT('',(-5.,-16.45,56.2783262011229));
#39606=CARTESIAN_POINT('Ctrl Pts',(71.8682453580158,-16.9981470538884,-3.57453458878626));
#39607=CARTESIAN_POINT('Ctrl Pts',(71.864163358506,-16.9983534204838,-3.57038661518133));
#39608=CARTESIAN_POINT('Ctrl Pts',(71.834280745957,-16.9997799301677,-3.5399078658621));
#39609=CARTESIAN_POINT('Ctrl Pts',(71.8016132291015,-16.9999870327594,-3.5064297689792));
#39610=CARTESIAN_POINT('Ctrl Pts',(71.7963365978802,-17.,-3.50104102377551));
#39611=CARTESIAN_POINT('Ctrl Pts',(71.7953186364093,-17.,-3.5));
#39612=CARTESIAN_POINT('Ctrl Pts',(72.103675101606,-16.9981470538884,-3.3391048451961));
#39613=CARTESIAN_POINT('Ctrl Pts',(72.0995711107311,-16.9983534204838,-3.33497886295621));
#39614=CARTESIAN_POINT('Ctrl Pts',(72.0694570586096,-16.9997799301677,-3.30473155320941));
#39615=CARTESIAN_POINT('Ctrl Pts',(72.0365616348729,-16.9999870327594,-3.27148136320785));
#39616=CARTESIAN_POINT('Ctrl Pts',(72.0312380731786,-17.,-3.26613954847708));
#39617=CARTESIAN_POINT('Ctrl Pts',(72.0302124242728,-17.,-3.26510621213642));
#39618=CARTESIAN_POINT('Ctrl Pts',(72.3391048451961,-16.9981470538884,-3.10367510160595));
#39619=CARTESIAN_POINT('Ctrl Pts',(72.3349788629562,-16.9983534204838,-3.09957111073108));
#39620=CARTESIAN_POINT('Ctrl Pts',(72.3045547255514,-17.0000242835561,-3.06945705860968));
#39621=CARTESIAN_POINT('Ctrl Pts',(72.2714568031683,-16.9998354184739,-3.03656163487291));
#39622=CARTESIAN_POINT('Ctrl Pts',(72.2661395484771,-17.,-3.03123807317865));
#39623=CARTESIAN_POINT('Ctrl Pts',(72.2651062121364,-17.,-3.03021242427284));
#39624=CARTESIAN_POINT('Ctrl Pts',(72.5745345887863,-16.9981470538884,-2.86824535801579));
#39625=CARTESIAN_POINT('Ctrl Pts',(72.5703866151813,-16.9983534204838,-2.86416335850595));
#39626=CARTESIAN_POINT('Ctrl Pts',(72.5399078658621,-16.9997799301677,-2.83428074595699));
#39627=CARTESIAN_POINT('Ctrl Pts',(72.5064297689792,-16.9999870327594,-2.80161322910156));
#39628=CARTESIAN_POINT('Ctrl Pts',(72.5010410237755,-17.,-2.79633659788022));
#39629=CARTESIAN_POINT('Ctrl Pts',(72.5,-17.,-2.79531863640926));
#39630=CARTESIAN_POINT('',(71.7953186364093,-17.,-3.5));
#39631=CARTESIAN_POINT('',(71.8682453580158,-16.9981470538884,-3.57453458878626));
#39632=CARTESIAN_POINT('Ctrl Pts',(71.7953186364093,-17.,-3.5));
#39633=CARTESIAN_POINT('Ctrl Pts',(71.7956426566413,-17.,-3.50033136103367));
#39634=CARTESIAN_POINT('Ctrl Pts',(71.7959698710105,-16.9999999087783,-3.50066599103948));
#39635=CARTESIAN_POINT('Ctrl Pts',(71.7963728195339,-16.9999996125274,-3.5010781547591));
#39636=CARTESIAN_POINT('Ctrl Pts',(71.7967957210522,-16.9999993016069,-3.50151072778697));
#39637=CARTESIAN_POINT('Ctrl Pts',(71.7973018394014,-16.999998768055,-3.50202849537422));
#39638=CARTESIAN_POINT('Ctrl Pts',(71.7979344421874,-16.9999976134245,-3.50267576544796));
#39639=CARTESIAN_POINT('Ctrl Pts',(71.798608415722,-16.9999963832839,-3.5033653654769));
#39640=CARTESIAN_POINT('Ctrl Pts',(71.7994256794686,-16.9999944448324,-3.50420167541479));
#39641=CARTESIAN_POINT('Ctrl Pts',(71.8003972134396,-16.9999910006556,-3.50519595537292));
#39642=CARTESIAN_POINT('Ctrl Pts',(71.8014697058444,-16.9999871985718,-3.50629355744886));
#39643=CARTESIAN_POINT('Ctrl Pts',(71.8027297908792,-16.9999815341953,-3.50758325228926));
#39644=CARTESIAN_POINT('Ctrl Pts',(71.804148443709,-16.9999727872824,-3.50903534240297));
#39645=CARTESIAN_POINT('Ctrl Pts',(71.8059282949088,-16.9999618133477,-3.51085714423971));
#39646=CARTESIAN_POINT('Ctrl Pts',(71.8079568545965,-16.9999458718544,-3.51293366154225));
#39647=CARTESIAN_POINT('Ctrl Pts',(71.8101187023246,-16.9999235237508,-3.51514671247941));
#39648=CARTESIAN_POINT('Ctrl Pts',(71.8124121613865,-16.9998998151149,-3.51749449195541));
#39649=CARTESIAN_POINT('Ctrl Pts',(71.8148508937686,-16.9998688531822,-3.51999108761023));
#39650=CARTESIAN_POINT('Ctrl Pts',(71.8172869062403,-16.9998314674613,-3.52248486630896));
#39651=CARTESIAN_POINT('Ctrl Pts',(71.8191324991579,-16.9998031429668,-3.52437422457692));
#39652=CARTESIAN_POINT('Ctrl Pts',(71.8209757293308,-16.9997712320714,-3.52626114404862));
#39653=CARTESIAN_POINT('Ctrl Pts',(71.822775757931,-16.9997367040829,-3.52810370841076));
#39654=CARTESIAN_POINT('Ctrl Pts',(71.824400036902,-16.9997055473083,-3.52976637007407));
#39655=CARTESIAN_POINT('Ctrl Pts',(71.8259887368554,-16.9996723091153,-3.53139250445799));
#39656=CARTESIAN_POINT('Ctrl Pts',(71.8275407505538,-16.9996373773349,-3.53298085050784));
#39657=CARTESIAN_POINT('Ctrl Pts',(71.8290718023242,-16.9996029173527,-3.53454774391483));
#39658=CARTESIAN_POINT('Ctrl Pts',(71.8305664957214,-16.9995668629652,-3.53607719242333));
#39659=CARTESIAN_POINT('Ctrl Pts',(71.8320614739058,-16.9995285090951,-3.53760652085725));
#39660=CARTESIAN_POINT('Ctrl Pts',(71.8335194958998,-16.9994911033411,-3.53909804395501));
#39661=CARTESIAN_POINT('Ctrl Pts',(71.8349843334469,-16.9994513364011,-3.54059613558274));
#39662=CARTESIAN_POINT('Ctrl Pts',(71.8364852326096,-16.9994082206029,-3.54213060631543));
#39663=CARTESIAN_POINT('Ctrl Pts',(71.8380984008872,-16.9993618796896,-3.543779857358));
#39664=CARTESIAN_POINT('Ctrl Pts',(71.8397528770163,-16.9993116397098,-3.54547077478768));
#39665=CARTESIAN_POINT('Ctrl Pts',(71.8414428847978,-16.9992572833264,-3.54719744053074));
#39666=CARTESIAN_POINT('Ctrl Pts',(71.8433735916158,-16.9991951852455,-3.54917002631353));
#39667=CARTESIAN_POINT('Ctrl Pts',(71.8453501484938,-16.9991276636876,-3.55118873161033));
#39668=CARTESIAN_POINT('Ctrl Pts',(71.8473171286807,-16.9990563957717,-3.55319701397667));
#39669=CARTESIAN_POINT('Ctrl Pts',(71.8500422837313,-16.9989576575525,-3.55597939118101));
#39670=CARTESIAN_POINT('Ctrl Pts',(71.8527461713318,-16.9988515979041,-3.5587388045199));
#39671=CARTESIAN_POINT('Ctrl Pts',(71.8552161386877,-16.9987486082515,-3.56125854441687));
#39672=CARTESIAN_POINT('Ctrl Pts',(71.8570686142046,-16.9986713660121,-3.56314834933959));
#39673=CARTESIAN_POINT('Ctrl Pts',(71.8587868623066,-16.998596102758,-3.56490064570692));
#39674=CARTESIAN_POINT('Ctrl Pts',(71.8602963585415,-16.9985278711001,-3.56643959313724));
#39675=CARTESIAN_POINT('Ctrl Pts',(71.8615610437189,-16.9984707052957,-3.5677289530965));
#39676=CARTESIAN_POINT('Ctrl Pts',(71.8626788313975,-16.9984185388897,-3.56886818435398));
#39677=CARTESIAN_POINT('Ctrl Pts',(71.8636316653216,-16.998373289921,-3.56983898661491));
#39678=CARTESIAN_POINT('Ctrl Pts',(71.8645275000202,-16.9983307477788,-3.57075171477112));
#39679=CARTESIAN_POINT('Ctrl Pts',(71.8652771155594,-16.9982943574932,-3.57151514502298));
#39680=CARTESIAN_POINT('Ctrl Pts',(71.8658958651526,-16.9982640274543,-3.5721450208714));
#39681=CARTESIAN_POINT('Ctrl Pts',(71.8664725654875,-16.9982357585976,-3.5727320913385));
#39682=CARTESIAN_POINT('Ctrl Pts',(71.8669354348749,-16.9982127623775,-3.57320299278075));
#39683=CARTESIAN_POINT('Ctrl Pts',(71.867327729259,-16.9981931657129,-3.57360188999627));
#39684=CARTESIAN_POINT('Ctrl Pts',(71.8676698713729,-16.9981760743537,-3.57394979081276));
#39685=CARTESIAN_POINT('Ctrl Pts',(71.8679585937126,-16.9981615513357,-3.57424318974083));
#39686=CARTESIAN_POINT('Ctrl Pts',(71.8682453580158,-16.9981470538884,-3.57453458878626));
#39687=CARTESIAN_POINT('',(72.5745345887863,-16.9981470538884,-2.86824535801579));
#39688=CARTESIAN_POINT('Ctrl Pts',(72.5745345887863,-16.9981470538884,-2.86824535801579));
#39689=CARTESIAN_POINT('Ctrl Pts',(72.3391048451961,-16.9981470538884,-3.10367510160595));
#39690=CARTESIAN_POINT('Ctrl Pts',(72.103675101606,-16.9981470538884,-3.3391048451961));
#39691=CARTESIAN_POINT('Ctrl Pts',(71.8682453580158,-16.9981470538884,-3.57453458878626));
#39692=CARTESIAN_POINT('',(72.5,-17.,-2.79531863640926));
#39693=CARTESIAN_POINT('Ctrl Pts',(72.5745345887863,-16.9981470538884,-2.86824535801579));
#39694=CARTESIAN_POINT('Ctrl Pts',(72.5742044925281,-16.9981634765679,-2.86792051198431));
#39695=CARTESIAN_POINT('Ctrl Pts',(72.5738711310018,-16.9981799708645,-2.86759246756107));
#39696=CARTESIAN_POINT('Ctrl Pts',(72.5734604128101,-16.9982001093812,-2.86718860352498));
#39697=CARTESIAN_POINT('Ctrl Pts',(72.57302935509,-16.9982212451946,-2.86676473939109));
#39698=CARTESIAN_POINT('Ctrl Pts',(72.572513296839,-16.9982463879926,-2.86625756382415));
#39699=CARTESIAN_POINT('Ctrl Pts',(72.5718680115172,-16.9982773404549,-2.86562376912052));
#39700=CARTESIAN_POINT('Ctrl Pts',(72.5711805211291,-16.9983103173716,-2.86494852089771));
#39701=CARTESIAN_POINT('Ctrl Pts',(72.5703466306137,-16.9983498713227,-2.86412982782487));
#39702=CARTESIAN_POINT('Ctrl Pts',(72.5693550535868,-16.9983957676602,-2.86315671761943));
#39703=CARTESIAN_POINT('Ctrl Pts',(72.5682604104266,-16.9984464345378,-2.8620824607523));
#39704=CARTESIAN_POINT('Ctrl Pts',(72.5669740091159,-16.9985047829815,-2.86082042406594));
#39705=CARTESIAN_POINT('Ctrl Pts',(72.565525387959,-16.9985681244217,-2.85939970674285));
#39706=CARTESIAN_POINT('Ctrl Pts',(72.5637077270911,-16.9986476022457,-2.8576170582772));
#39707=CARTESIAN_POINT('Ctrl Pts',(72.5616355608823,-16.9987347812318,-2.85558546640713));
#39708=CARTESIAN_POINT('Ctrl Pts',(72.5594266767905,-16.9988223610841,-2.85342062894714));
#39709=CARTESIAN_POINT('Ctrl Pts',(72.5570842219804,-16.9989152368701,-2.85112488425853));
#39710=CARTESIAN_POINT('Ctrl Pts',(72.5545928471898,-16.9990082804756,-2.8486840335237));
#39711=CARTESIAN_POINT('Ctrl Pts',(72.552103587594,-16.9990947989236,-2.84624625175195));
#39712=CARTESIAN_POINT('Ctrl Pts',(72.5502173068831,-16.9991603598156,-2.84439897927724));
#39713=CARTESIAN_POINT('Ctrl Pts',(72.5483330647398,-16.9992222334679,-2.84255427195848));
#39714=CARTESIAN_POINT('Ctrl Pts',(72.5464926261216,-16.9992793054386,-2.84075306394266));
#39715=CARTESIAN_POINT('Ctrl Pts',(72.5448318572274,-16.9993308058541,-2.83912769582928));
#39716=CARTESIAN_POINT('Ctrl Pts',(72.543207168852,-16.9993784253393,-2.83753815081149));
#39717=CARTESIAN_POINT('Ctrl Pts',(72.5416197584348,-16.9994224873957,-2.83598557864455));
#39718=CARTESIAN_POINT('Ctrl Pts',(72.540053319257,-16.9994659673493,-2.83445351746977));
#39719=CARTESIAN_POINT('Ctrl Pts',(72.5385238533706,-16.9995060035546,-2.83295811821705));
#39720=CARTESIAN_POINT('Ctrl Pts',(72.5369939676884,-16.9995437460623,-2.83146270058428));
#39721=CARTESIAN_POINT('Ctrl Pts',(72.5355023760137,-16.9995805438512,-2.83000471420189));
#39722=CARTESIAN_POINT('Ctrl Pts',(72.5340037037557,-16.9996153196962,-2.82854016663104));
#39723=CARTESIAN_POINT('Ctrl Pts',(72.5324681805947,-16.9996485645807,-2.82703981578639));
#39724=CARTESIAN_POINT('Ctrl Pts',(72.5308177719951,-16.9996842967954,-2.82542721104074));
#39725=CARTESIAN_POINT('Ctrl Pts',(72.529125149268,-16.9997182120423,-2.82377359513262));
#39726=CARTESIAN_POINT('Ctrl Pts',(72.5273963190708,-16.9997497930326,-2.82208470500297));
#39727=CARTESIAN_POINT('Ctrl Pts',(72.5254211385424,-16.9997858741684,-2.8201551558175));
#39728=CARTESIAN_POINT('Ctrl Pts',(72.5233992312896,-16.9998188305302,-2.81818008615894));
#39729=CARTESIAN_POINT('Ctrl Pts',(72.52138736276,-16.9998475191546,-2.81621482751819));
#39730=CARTESIAN_POINT('Ctrl Pts',(72.5186005402079,-16.9998872583841,-2.81349256857325));
#39731=CARTESIAN_POINT('Ctrl Pts',(72.5158359360068,-16.9999185308537,-2.81079201806525));
#39732=CARTESIAN_POINT('Ctrl Pts',(72.5133109478137,-16.9999409383933,-2.8083253911404));
#39733=CARTESIAN_POINT('Ctrl Pts',(72.5114172066689,-16.9999577440481,-2.80647542094677));
#39734=CARTESIAN_POINT('Ctrl Pts',(72.5096609508553,-16.9999696816405,-2.80475967567116));
#39735=CARTESIAN_POINT('Ctrl Pts',(72.508118309431,-16.9999780308564,-2.803252515256));
#39736=CARTESIAN_POINT('Ctrl Pts',(72.5068258239489,-16.999985026157,-2.80198975715482));
#39737=CARTESIAN_POINT('Ctrl Pts',(72.5056836631397,-16.9999895478102,-2.80087378577512));
#39738=CARTESIAN_POINT('Ctrl Pts',(72.5047102375997,-16.9999926045357,-2.79992260032024));
#39739=CARTESIAN_POINT('Ctrl Pts',(72.5037950311059,-16.9999954784432,-2.79902830376709));
#39740=CARTESIAN_POINT('Ctrl Pts',(72.5030293988184,-16.9999970739683,-2.79828008131994));
#39741=CARTESIAN_POINT('Ctrl Pts',(72.5023976001144,-16.9999980838367,-2.79766257486899));
#39742=CARTESIAN_POINT('Ctrl Pts',(72.5018087302087,-16.9999990250876,-2.79708702610116));
#39743=CARTESIAN_POINT('Ctrl Pts',(72.5013362750362,-16.9999994582021,-2.79662518068281));
#39744=CARTESIAN_POINT('Ctrl Pts',(72.500935978419,-16.9999997079814,-2.79623381941522));
#39745=CARTESIAN_POINT('Ctrl Pts',(72.5005869205336,-16.9999999257886,-2.79589255313753));
#39746=CARTESIAN_POINT('Ctrl Pts',(72.5002924603909,-17.,-2.79560461778332));
#39747=CARTESIAN_POINT('Ctrl Pts',(72.5,-17.,-2.79531863640926));
#39748=CARTESIAN_POINT('',(72.1476593182046,-17.,-3.14765931820463));
#39749=CARTESIAN_POINT('Ctrl Pts',(72.5745345887863,-16.9981470538884,-2.86824535801579));
#39750=CARTESIAN_POINT('Ctrl Pts',(72.8307391591089,-16.9854005733312,-3.12037495913795));
#39751=CARTESIAN_POINT('Ctrl Pts',(73.3201733549766,-16.8268077199093,-3.63377877163944));
#39752=CARTESIAN_POINT('Ctrl Pts',(73.7358067305414,-16.3991227020429,-4.13541628736354));
#39753=CARTESIAN_POINT('Ctrl Pts',(73.9615602058987,-15.9274342791999,-4.43902863521564));
#39754=CARTESIAN_POINT('Ctrl Pts',(74.,-15.6672482052684,-4.5));
#39755=CARTESIAN_POINT('Ctrl Pts',(74.,-15.5,-4.5));
#39756=CARTESIAN_POINT('Ctrl Pts',(72.3391048451961,-16.9981470538884,-3.10367510160595));
#39757=CARTESIAN_POINT('Ctrl Pts',(72.5939510924519,-16.9854005733312,-3.35716302579494));
#39758=CARTESIAN_POINT('Ctrl Pts',(73.0913751605309,-16.8268077199093,-3.86257696608515));
#39759=CARTESIAN_POINT('Ctrl Pts',(73.5356765828155,-16.3991227020429,-4.3355464350895));
#39760=CARTESIAN_POINT('Ctrl Pts',(73.7873830156711,-15.9274342791999,-4.61320582544333));
#39761=CARTESIAN_POINT('Ctrl Pts',(73.8333333333333,-15.6672482052684,-4.66666666666667));
#39762=CARTESIAN_POINT('Ctrl Pts',(73.8333333333333,-15.5,-4.66666666666667));
#39763=CARTESIAN_POINT('Ctrl Pts',(72.103675101606,-16.9981470538884,-3.3391048451961));
#39764=CARTESIAN_POINT('Ctrl Pts',(72.3571630257949,-16.9854005733312,-3.59395109245193));
#39765=CARTESIAN_POINT('Ctrl Pts',(72.8625769660852,-16.8268077199093,-4.09137516053087));
#39766=CARTESIAN_POINT('Ctrl Pts',(73.3355464350895,-16.3991227020429,-4.53567658281546));
#39767=CARTESIAN_POINT('Ctrl Pts',(73.6132058254434,-15.9274342791999,-4.78738301567102));
#39768=CARTESIAN_POINT('Ctrl Pts',(73.6666666666667,-15.6672482052684,-4.83333333333333));
#39769=CARTESIAN_POINT('Ctrl Pts',(73.6666666666667,-15.5,-4.83333333333333));
#39770=CARTESIAN_POINT('Ctrl Pts',(71.8682453580158,-16.9981470538884,-3.57453458878626));
#39771=CARTESIAN_POINT('Ctrl Pts',(72.120374959138,-16.9854005733312,-3.83073915910891));
#39772=CARTESIAN_POINT('Ctrl Pts',(72.6337787716395,-16.8268077199093,-4.32017335497659));
#39773=CARTESIAN_POINT('Ctrl Pts',(73.1354162873635,-16.3991227020429,-4.73580673054142));
#39774=CARTESIAN_POINT('Ctrl Pts',(73.4390286352157,-15.9274342791999,-4.9615602058987));
#39775=CARTESIAN_POINT('Ctrl Pts',(73.5,-15.6672482052684,-5.));
#39776=CARTESIAN_POINT('Ctrl Pts',(73.5,-15.5,-5.));
#39777=CARTESIAN_POINT('',(73.5,-15.5,-5.));
#39778=CARTESIAN_POINT('Ctrl Pts',(71.8682453580158,-16.9981470538884,-3.57453458878626));
#39779=CARTESIAN_POINT('Ctrl Pts',(72.120374959138,-16.9854005733312,-3.83073915910891));
#39780=CARTESIAN_POINT('Ctrl Pts',(72.6337787716395,-16.8268077199093,-4.32017335497659));
#39781=CARTESIAN_POINT('Ctrl Pts',(73.1354162873635,-16.3991227020429,-4.73580673054142));
#39782=CARTESIAN_POINT('Ctrl Pts',(73.4390286352157,-15.9274342791999,-4.9615602058987));
#39783=CARTESIAN_POINT('Ctrl Pts',(73.5,-15.6672482052684,-5.));
#39784=CARTESIAN_POINT('Ctrl Pts',(73.5,-15.5,-5.));
#39785=CARTESIAN_POINT('',(74.,-15.5,-4.5));
#39786=CARTESIAN_POINT('',(73.5,-15.5,-5.));
#39787=CARTESIAN_POINT('Ctrl Pts',(74.,-15.5,-4.5));
#39788=CARTESIAN_POINT('Ctrl Pts',(74.,-15.6672482052684,-4.5));
#39789=CARTESIAN_POINT('Ctrl Pts',(73.9615602058987,-15.9274342791999,-4.43902863521564));
#39790=CARTESIAN_POINT('Ctrl Pts',(73.7358067305414,-16.3991227020429,-4.13541628736354));
#39791=CARTESIAN_POINT('Ctrl Pts',(73.3201733549766,-16.8268077199093,-3.63377877163944));
#39792=CARTESIAN_POINT('Ctrl Pts',(72.8307391591089,-16.9854005733312,-3.12037495913795));
#39793=CARTESIAN_POINT('Ctrl Pts',(72.5745345887863,-16.9981470538884,-2.86824535801579));
#39794=CARTESIAN_POINT('Origin',(73.75,-14.,-4.75));
#39795=CARTESIAN_POINT('',(73.5,-14.,-5.));
#39796=CARTESIAN_POINT('',(74.,-14.,-4.5));
#39797=CARTESIAN_POINT('',(79.2500000000001,-14.,0.750000000000108));
#39798=CARTESIAN_POINT('',(74.,-14.,-4.5));
#39799=CARTESIAN_POINT('',(73.5,-14.,-5.));
#39800=CARTESIAN_POINT('Origin',(62.,-17.,0.));
#39801=CARTESIAN_POINT('',(72.5,-17.,2.79531863640926));
#39802=CARTESIAN_POINT('',(72.5,-17.,-2.5));
#39803=CARTESIAN_POINT('',(71.7953186364093,-17.,3.5));
#39804=CARTESIAN_POINT('',(72.1476593182046,-17.,3.14765931820463));
#39805=CARTESIAN_POINT('',(56.3914887194867,-17.,3.5));
#39806=CARTESIAN_POINT('',(68.,-17.,3.5));
#39807=CARTESIAN_POINT('',(56.3914887194867,-17.,-3.5));
#39808=CARTESIAN_POINT('Origin',(0.,-17.,0.));
#39809=CARTESIAN_POINT('',(56.,-17.,-3.5));
#39810=CARTESIAN_POINT('Origin',(72.5,-15.5,-2.5));
#39811=CARTESIAN_POINT('',(74.,-15.5,4.5));
#39812=CARTESIAN_POINT('',(74.,-15.5,-2.5));
#39813=CARTESIAN_POINT('',(72.5745345887863,-16.9981470538884,2.86824535801578));
#39814=CARTESIAN_POINT('Ctrl Pts',(72.5745345887863,-16.9981470538884,2.86824535801578));
#39815=CARTESIAN_POINT('Ctrl Pts',(72.8307391591089,-16.9854005733312,3.12037495913794));
#39816=CARTESIAN_POINT('Ctrl Pts',(73.3201733549766,-16.8268077199093,3.63377877163943));
#39817=CARTESIAN_POINT('Ctrl Pts',(73.7358067305414,-16.3991227020429,4.13541628736354));
#39818=CARTESIAN_POINT('Ctrl Pts',(73.9615602058987,-15.9274342791999,4.43902863521564));
#39819=CARTESIAN_POINT('Ctrl Pts',(74.,-15.6672482052684,4.5));
#39820=CARTESIAN_POINT('Ctrl Pts',(74.,-15.5,4.5));
#39821=CARTESIAN_POINT('Ctrl Pts',(72.5,-17.,2.79531863640926));
#39822=CARTESIAN_POINT('Ctrl Pts',(72.5003313610337,-17.,2.79564265664126));
#39823=CARTESIAN_POINT('Ctrl Pts',(72.5006659910395,-16.9999999087783,2.79596987101049));
#39824=CARTESIAN_POINT('Ctrl Pts',(72.5010781547591,-16.9999996125274,2.79637281953386));
#39825=CARTESIAN_POINT('Ctrl Pts',(72.501510727787,-16.9999993016069,2.79679572105221));
#39826=CARTESIAN_POINT('Ctrl Pts',(72.5020284953742,-16.999998768055,2.79730183940144));
#39827=CARTESIAN_POINT('Ctrl Pts',(72.502675765448,-16.9999976134245,2.79793444218739));
#39828=CARTESIAN_POINT('Ctrl Pts',(72.5033653654769,-16.9999963832839,2.79860841572208));
#39829=CARTESIAN_POINT('Ctrl Pts',(72.5042016754148,-16.9999944448324,2.79942567946861));
#39830=CARTESIAN_POINT('Ctrl Pts',(72.5051959553729,-16.9999910006556,2.80039721343955));
#39831=CARTESIAN_POINT('Ctrl Pts',(72.5062935574489,-16.9999871985718,2.80146970584437));
#39832=CARTESIAN_POINT('Ctrl Pts',(72.5075832522893,-16.9999815341953,2.80272979087918));
#39833=CARTESIAN_POINT('Ctrl Pts',(72.509035342403,-16.9999727872824,2.80414844370901));
#39834=CARTESIAN_POINT('Ctrl Pts',(72.5108571442397,-16.9999618133477,2.80592829490876));
#39835=CARTESIAN_POINT('Ctrl Pts',(72.5129336615422,-16.9999458718544,2.80795685459655));
#39836=CARTESIAN_POINT('Ctrl Pts',(72.5151467124794,-16.9999235237508,2.81011870232459));
#39837=CARTESIAN_POINT('Ctrl Pts',(72.5174944919554,-16.9998998151149,2.81241216138644));
#39838=CARTESIAN_POINT('Ctrl Pts',(72.5199910876102,-16.9998688531822,2.81485089376853));
#39839=CARTESIAN_POINT('Ctrl Pts',(72.5224848663089,-16.9998314674613,2.81728690624033));
#39840=CARTESIAN_POINT('Ctrl Pts',(72.5243742245769,-16.9998031429668,2.81913249915794));
#39841=CARTESIAN_POINT('Ctrl Pts',(72.5262611440486,-16.9997712320714,2.82097572933083));
#39842=CARTESIAN_POINT('Ctrl Pts',(72.5281037084107,-16.9997367040829,2.82277575793095));
#39843=CARTESIAN_POINT('Ctrl Pts',(72.529766370074,-16.9997055473083,2.824400036902));
#39844=CARTESIAN_POINT('Ctrl Pts',(72.5313925044579,-16.9996723091153,2.82598873685535));
#39845=CARTESIAN_POINT('Ctrl Pts',(72.5329808505078,-16.9996373773349,2.82754075055375));
#39846=CARTESIAN_POINT('Ctrl Pts',(72.5345477439147,-16.9996029173527,2.82907180232405));
#39847=CARTESIAN_POINT('Ctrl Pts',(72.5360771924231,-16.9995668629652,2.83056649572116));
#39848=CARTESIAN_POINT('Ctrl Pts',(72.5376065208569,-16.9995285090951,2.83206147390553));
#39849=CARTESIAN_POINT('Ctrl Pts',(72.5390980439547,-16.9994911033411,2.83351949589957));
#39850=CARTESIAN_POINT('Ctrl Pts',(72.5405961355824,-16.9994513364011,2.83498433344659));
#39851=CARTESIAN_POINT('Ctrl Pts',(72.5421306063151,-16.9994082206029,2.8364852326093));
#39852=CARTESIAN_POINT('Ctrl Pts',(72.5437798573576,-16.9993618796896,2.83809840088688));
#39853=CARTESIAN_POINT('Ctrl Pts',(72.5454707747873,-16.9993116397099,2.83975287701592));
#39854=CARTESIAN_POINT('Ctrl Pts',(72.5471974405303,-16.9992572833264,2.84144288479735));
#39855=CARTESIAN_POINT('Ctrl Pts',(72.549170026313,-16.9991951852455,2.84337359161536));
#39856=CARTESIAN_POINT('Ctrl Pts',(72.5511887316098,-16.9991276636876,2.84535014849327));
#39857=CARTESIAN_POINT('Ctrl Pts',(72.5531970139762,-16.9990563957717,2.84731712868022));
#39858=CARTESIAN_POINT('Ctrl Pts',(72.5559793911805,-16.9989576575525,2.85004228373082));
#39859=CARTESIAN_POINT('Ctrl Pts',(72.5587388045195,-16.9988515979041,2.85274617133141));
#39860=CARTESIAN_POINT('Ctrl Pts',(72.5612585444165,-16.9987486082516,2.85521613868735));
#39861=CARTESIAN_POINT('Ctrl Pts',(72.5631483493393,-16.9986713660122,2.8570686142043));
#39862=CARTESIAN_POINT('Ctrl Pts',(72.5649006457067,-16.998596102758,2.8587868623063));
#39863=CARTESIAN_POINT('Ctrl Pts',(72.566439593137,-16.9985278711001,2.86029635854127));
#39864=CARTESIAN_POINT('Ctrl Pts',(72.5677289530963,-16.9984707052957,2.86156104371873));
#39865=CARTESIAN_POINT('Ctrl Pts',(72.5688681843538,-16.9984185388897,2.86267883139733));
#39866=CARTESIAN_POINT('Ctrl Pts',(72.5698389866148,-16.998373289921,2.8636316653215));
#39867=CARTESIAN_POINT('Ctrl Pts',(72.570751714771,-16.9983307477788,2.86452750002005));
#39868=CARTESIAN_POINT('Ctrl Pts',(72.5715151450229,-16.9982943574932,2.86527711555929));
#39869=CARTESIAN_POINT('Ctrl Pts',(72.5721450208713,-16.9982640274543,2.86589586515251));
#39870=CARTESIAN_POINT('Ctrl Pts',(72.5727320913384,-16.9982357585976,2.86647256548738));
#39871=CARTESIAN_POINT('Ctrl Pts',(72.5732029927807,-16.9982127623775,2.86693543487483));
#39872=CARTESIAN_POINT('Ctrl Pts',(72.5736018899962,-16.9981931657129,2.86732772925895));
#39873=CARTESIAN_POINT('Ctrl Pts',(72.5739497908127,-16.9981760743537,2.86766987137284));
#39874=CARTESIAN_POINT('Ctrl Pts',(72.5742431897408,-16.9981615513357,2.86795859371254));
#39875=CARTESIAN_POINT('Ctrl Pts',(72.5745345887863,-16.9981470538884,2.86824535801578));
#39876=CARTESIAN_POINT('Origin',(74.,-14.,-5.));
#39877=CARTESIAN_POINT('',(74.,-14.,4.5));
#39878=CARTESIAN_POINT('',(74.,-14.,43.));
#39879=CARTESIAN_POINT('',(74.,-14.,4.5));
#39880=CARTESIAN_POINT('Ctrl Pts',(72.5745345887863,-16.9981470538884,2.86824535801578));
#39881=CARTESIAN_POINT('Ctrl Pts',(72.5703866151813,-16.9983534204838,2.86416335850594));
#39882=CARTESIAN_POINT('Ctrl Pts',(72.5399078658621,-16.9997799301677,2.83428074595701));
#39883=CARTESIAN_POINT('Ctrl Pts',(72.5064297689792,-16.9999870327594,2.80161322910156));
#39884=CARTESIAN_POINT('Ctrl Pts',(72.5010410237755,-17.,2.79633659788022));
#39885=CARTESIAN_POINT('Ctrl Pts',(72.5,-17.,2.79531863640926));
#39886=CARTESIAN_POINT('Ctrl Pts',(72.3391048451961,-16.9981470538884,3.10367510160594));
#39887=CARTESIAN_POINT('Ctrl Pts',(72.3349788629562,-16.9983534204838,3.09957111073107));
#39888=CARTESIAN_POINT('Ctrl Pts',(72.3047315532094,-16.9997799301677,3.06945705860969));
#39889=CARTESIAN_POINT('Ctrl Pts',(72.2714813632079,-16.9999870327594,3.03656163487291));
#39890=CARTESIAN_POINT('Ctrl Pts',(72.2661395484771,-17.,3.03123807317865));
#39891=CARTESIAN_POINT('Ctrl Pts',(72.2651062121364,-17.,3.03021242427284));
#39892=CARTESIAN_POINT('Ctrl Pts',(72.1036751016059,-16.9981470538884,3.3391048451961));
#39893=CARTESIAN_POINT('Ctrl Pts',(72.0995711107311,-16.9983534204838,3.3349788629562));
#39894=CARTESIAN_POINT('Ctrl Pts',(72.0694570586097,-17.0000242835561,3.30455472555144));
#39895=CARTESIAN_POINT('Ctrl Pts',(72.0365616348729,-16.9998354184739,3.27145680316828));
#39896=CARTESIAN_POINT('Ctrl Pts',(72.0312380731786,-17.,3.26613954847708));
#39897=CARTESIAN_POINT('Ctrl Pts',(72.0302124242728,-17.,3.26510621213642));
#39898=CARTESIAN_POINT('Ctrl Pts',(71.8682453580158,-16.9981470538884,3.57453458878625));
#39899=CARTESIAN_POINT('Ctrl Pts',(71.8641633585059,-16.9983534204838,3.57038661518133));
#39900=CARTESIAN_POINT('Ctrl Pts',(71.834280745957,-16.9997799301677,3.53990786586208));
#39901=CARTESIAN_POINT('Ctrl Pts',(71.8016132291015,-16.9999870327594,3.50642976897919));
#39902=CARTESIAN_POINT('Ctrl Pts',(71.7963365978802,-17.,3.50104102377551));
#39903=CARTESIAN_POINT('Ctrl Pts',(71.7953186364093,-17.,3.5));
#39904=CARTESIAN_POINT('',(71.8682453580158,-16.9981470538884,3.57453458878625));
#39905=CARTESIAN_POINT('Ctrl Pts',(71.8682453580158,-16.9981470538884,3.57453458878625));
#39906=CARTESIAN_POINT('Ctrl Pts',(72.1036751016059,-16.9981470538884,3.3391048451961));
#39907=CARTESIAN_POINT('Ctrl Pts',(72.3391048451961,-16.9981470538884,3.10367510160594));
#39908=CARTESIAN_POINT('Ctrl Pts',(72.5745345887863,-16.9981470538884,2.86824535801578));
#39909=CARTESIAN_POINT('Ctrl Pts',(71.8682453580158,-16.9981470538884,3.57453458878625));
#39910=CARTESIAN_POINT('Ctrl Pts',(71.8679205119843,-16.9981634765679,3.57420449252804));
#39911=CARTESIAN_POINT('Ctrl Pts',(71.8675924675611,-16.9981799708645,3.57387113100175));
#39912=CARTESIAN_POINT('Ctrl Pts',(71.867188603525,-16.9982001093812,3.57346041281004));
#39913=CARTESIAN_POINT('Ctrl Pts',(71.8667647393911,-16.9982212451946,3.57302935509001));
#39914=CARTESIAN_POINT('Ctrl Pts',(71.8662575638241,-16.9982463879926,3.57251329683895));
#39915=CARTESIAN_POINT('Ctrl Pts',(71.8656237691205,-16.9982773404549,3.57186801151715));
#39916=CARTESIAN_POINT('Ctrl Pts',(71.8649485208977,-16.9983103173716,3.57118052112908));
#39917=CARTESIAN_POINT('Ctrl Pts',(71.8641298278249,-16.9983498713227,3.57034663061371));
#39918=CARTESIAN_POINT('Ctrl Pts',(71.8631567176194,-16.9983957676602,3.56935505358678));
#39919=CARTESIAN_POINT('Ctrl Pts',(71.8620824607523,-16.9984464345378,3.56826041042662));
#39920=CARTESIAN_POINT('Ctrl Pts',(71.8608204240659,-16.9985047829815,3.56697400911588));
#39921=CARTESIAN_POINT('Ctrl Pts',(71.8593997067429,-16.9985681244217,3.56552538795904));
#39922=CARTESIAN_POINT('Ctrl Pts',(71.8576170582772,-16.9986476022456,3.56370772709111));
#39923=CARTESIAN_POINT('Ctrl Pts',(71.8555854664071,-16.9987347812318,3.5616355608823));
#39924=CARTESIAN_POINT('Ctrl Pts',(71.8534206289472,-16.9988223610841,3.55942667679056));
#39925=CARTESIAN_POINT('Ctrl Pts',(71.8511248842585,-16.9989152368701,3.55708422198038));
#39926=CARTESIAN_POINT('Ctrl Pts',(71.8486840335237,-16.9990082804756,3.55459284718975));
#39927=CARTESIAN_POINT('Ctrl Pts',(71.8462462517519,-16.9990947989236,3.55210358759403));
#39928=CARTESIAN_POINT('Ctrl Pts',(71.8443989792772,-16.9991603598156,3.55021730688309));
#39929=CARTESIAN_POINT('Ctrl Pts',(71.8425542719585,-16.9992222334679,3.54833306473982));
#39930=CARTESIAN_POINT('Ctrl Pts',(71.8407530639426,-16.9992793054386,3.54649262612162));
#39931=CARTESIAN_POINT('Ctrl Pts',(71.8391276958293,-16.9993308058541,3.54483185722743));
#39932=CARTESIAN_POINT('Ctrl Pts',(71.8375381508115,-16.9993784253393,3.543207168852));
#39933=CARTESIAN_POINT('Ctrl Pts',(71.8359855786445,-16.9994224873957,3.54161975843481));
#39934=CARTESIAN_POINT('Ctrl Pts',(71.8344535174697,-16.9994659673493,3.54005331925702));
#39935=CARTESIAN_POINT('Ctrl Pts',(71.832958118217,-16.9995060035546,3.53852385337056));
#39936=CARTESIAN_POINT('Ctrl Pts',(71.8314627005842,-16.9995437460623,3.53699396768834));
#39937=CARTESIAN_POINT('Ctrl Pts',(71.8300047142018,-16.9995805438512,3.53550237601363));
#39938=CARTESIAN_POINT('Ctrl Pts',(71.828540166631,-16.9996153196962,3.53400370375568));
#39939=CARTESIAN_POINT('Ctrl Pts',(71.8270398157863,-16.9996485645807,3.53246818059467));
#39940=CARTESIAN_POINT('Ctrl Pts',(71.8254272110407,-16.9996842967954,3.53081777199503));
#39941=CARTESIAN_POINT('Ctrl Pts',(71.8237735951326,-16.9997182120423,3.52912514926797));
#39942=CARTESIAN_POINT('Ctrl Pts',(71.8220847050029,-16.9997497930326,3.52739631907077));
#39943=CARTESIAN_POINT('Ctrl Pts',(71.8201551558174,-16.9997858741684,3.52542113854231));
#39944=CARTESIAN_POINT('Ctrl Pts',(71.8181800861589,-16.9998188305302,3.52339923128955));
#39945=CARTESIAN_POINT('Ctrl Pts',(71.8162148275181,-16.9998475191546,3.52138736275992));
#39946=CARTESIAN_POINT('Ctrl Pts',(71.8134925685732,-16.9998872583841,3.51860054020779));
#39947=CARTESIAN_POINT('Ctrl Pts',(71.8107920180652,-16.9999185308537,3.51583593600674));
#39948=CARTESIAN_POINT('Ctrl Pts',(71.8083253911404,-16.9999409383933,3.51331094781366));
#39949=CARTESIAN_POINT('Ctrl Pts',(71.8064754209467,-16.9999577440481,3.51141720666885));
#39950=CARTESIAN_POINT('Ctrl Pts',(71.8047596756711,-16.9999696816405,3.50966095085529));
#39951=CARTESIAN_POINT('Ctrl Pts',(71.803252515256,-16.9999780308564,3.50811830943094));
#39952=CARTESIAN_POINT('Ctrl Pts',(71.8019897571548,-16.999985026157,3.50682582394882));
#39953=CARTESIAN_POINT('Ctrl Pts',(71.8008737857751,-16.9999895478102,3.50568366313965));
#39954=CARTESIAN_POINT('Ctrl Pts',(71.7999226003202,-16.9999926045357,3.50471023759971));
#39955=CARTESIAN_POINT('Ctrl Pts',(71.7990283037671,-16.9999954784432,3.50379503110591));
#39956=CARTESIAN_POINT('Ctrl Pts',(71.7982800813199,-16.9999970739683,3.50302939881839));
#39957=CARTESIAN_POINT('Ctrl Pts',(71.797662574869,-16.9999980838367,3.50239760011444));
#39958=CARTESIAN_POINT('Ctrl Pts',(71.7970870261012,-16.9999990250876,3.50180873020869));
#39959=CARTESIAN_POINT('Ctrl Pts',(71.7966251806828,-16.9999994582021,3.50133627503614));
#39960=CARTESIAN_POINT('Ctrl Pts',(71.7962338194152,-16.9999997079814,3.50093597841902));
#39961=CARTESIAN_POINT('Ctrl Pts',(71.7958925531375,-16.9999999257886,3.5005869205336));
#39962=CARTESIAN_POINT('Ctrl Pts',(71.7956046177833,-17.,3.50029246039093));
#39963=CARTESIAN_POINT('Ctrl Pts',(71.7953186364093,-17.,3.5));
#39964=CARTESIAN_POINT('Ctrl Pts',(71.8682453580158,-16.9981470538884,3.57453458878625));
#39965=CARTESIAN_POINT('Ctrl Pts',(72.1203749591379,-16.9854005733312,3.83073915910891));
#39966=CARTESIAN_POINT('Ctrl Pts',(72.6337787716394,-16.8268077199093,4.32017335497658));
#39967=CARTESIAN_POINT('Ctrl Pts',(73.1354162873635,-16.3991227020429,4.73580673054142));
#39968=CARTESIAN_POINT('Ctrl Pts',(73.4390286352156,-15.9274342791999,4.9615602058987));
#39969=CARTESIAN_POINT('Ctrl Pts',(73.5,-15.6672482052684,5.));
#39970=CARTESIAN_POINT('Ctrl Pts',(73.5,-15.5,5.));
#39971=CARTESIAN_POINT('Ctrl Pts',(72.1036751016059,-16.9981470538884,3.3391048451961));
#39972=CARTESIAN_POINT('Ctrl Pts',(72.3571630257949,-16.9854005733312,3.59395109245192));
#39973=CARTESIAN_POINT('Ctrl Pts',(72.8625769660851,-16.8268077199093,4.09137516053087));
#39974=CARTESIAN_POINT('Ctrl Pts',(73.3355464350895,-16.3991227020429,4.53567658281546));
#39975=CARTESIAN_POINT('Ctrl Pts',(73.6132058254433,-15.9274342791999,4.78738301567102));
#39976=CARTESIAN_POINT('Ctrl Pts',(73.6666666666667,-15.6672482052684,4.83333333333333));
#39977=CARTESIAN_POINT('Ctrl Pts',(73.6666666666667,-15.5,4.83333333333333));
#39978=CARTESIAN_POINT('Ctrl Pts',(72.3391048451961,-16.9981470538884,3.10367510160594));
#39979=CARTESIAN_POINT('Ctrl Pts',(72.5939510924519,-16.9854005733312,3.35716302579493));
#39980=CARTESIAN_POINT('Ctrl Pts',(73.0913751605309,-16.8268077199093,3.86257696608515));
#39981=CARTESIAN_POINT('Ctrl Pts',(73.5356765828154,-16.3991227020429,4.3355464350895));
#39982=CARTESIAN_POINT('Ctrl Pts',(73.787383015671,-15.9274342791999,4.61320582544333));
#39983=CARTESIAN_POINT('Ctrl Pts',(73.8333333333333,-15.6672482052684,4.66666666666667));
#39984=CARTESIAN_POINT('Ctrl Pts',(73.8333333333333,-15.5,4.66666666666667));
#39985=CARTESIAN_POINT('Ctrl Pts',(72.5745345887863,-16.9981470538884,2.86824535801578));
#39986=CARTESIAN_POINT('Ctrl Pts',(72.8307391591089,-16.9854005733312,3.12037495913794));
#39987=CARTESIAN_POINT('Ctrl Pts',(73.3201733549766,-16.8268077199093,3.63377877163943));
#39988=CARTESIAN_POINT('Ctrl Pts',(73.7358067305414,-16.3991227020429,4.13541628736354));
#39989=CARTESIAN_POINT('Ctrl Pts',(73.9615602058987,-15.9274342791999,4.43902863521564));
#39990=CARTESIAN_POINT('Ctrl Pts',(74.,-15.6672482052684,4.5));
#39991=CARTESIAN_POINT('Ctrl Pts',(74.,-15.5,4.5));
#39992=CARTESIAN_POINT('',(73.5,-15.5,5.));
#39993=CARTESIAN_POINT('',(74.,-15.5,4.5));
#39994=CARTESIAN_POINT('Ctrl Pts',(73.5,-15.5,5.));
#39995=CARTESIAN_POINT('Ctrl Pts',(73.5,-15.6672482052684,5.));
#39996=CARTESIAN_POINT('Ctrl Pts',(73.4390286352156,-15.9274342791999,4.9615602058987));
#39997=CARTESIAN_POINT('Ctrl Pts',(73.1354162873635,-16.3991227020429,4.73580673054142));
#39998=CARTESIAN_POINT('Ctrl Pts',(72.6337787716394,-16.8268077199093,4.32017335497658));
#39999=CARTESIAN_POINT('Ctrl Pts',(72.1203749591379,-16.9854005733312,3.83073915910891));
#40000=CARTESIAN_POINT('Ctrl Pts',(71.8682453580158,-16.9981470538884,3.57453458878625));
#40001=CARTESIAN_POINT('Origin',(73.75,-14.,4.75));
#40002=CARTESIAN_POINT('',(73.5,-14.,5.));
#40003=CARTESIAN_POINT('',(33.7499999999998,-14.,44.7499999999997));
#40004=CARTESIAN_POINT('',(73.5,-14.,5.));
#40005=CARTESIAN_POINT('Origin',(68.,-15.5,3.5));
#40006=CARTESIAN_POINT('',(56.2783262011229,-15.5,5.));
#40007=CARTESIAN_POINT('',(68.,-15.5,5.));
#40008=CARTESIAN_POINT('Ctrl Pts',(56.3914887194867,-17.,3.5));
#40009=CARTESIAN_POINT('Ctrl Pts',(56.379789702144,-17.,3.68849285843233));
#40010=CARTESIAN_POINT('Ctrl Pts',(56.366268079425,-16.9623071985392,3.88949595769794));
#40011=CARTESIAN_POINT('Ctrl Pts',(56.3395353657988,-16.8090480003591,4.25923828551908));
#40012=CARTESIAN_POINT('Ctrl Pts',(56.3263779287031,-16.6934822832211,4.42798167302478));
#40013=CARTESIAN_POINT('Ctrl Pts',(56.3048219679644,-16.4270526075957,4.69412389350913));
#40014=CARTESIAN_POINT('Ctrl Pts',(56.2949857165266,-16.2585410496607,4.8094152373875));
#40015=CARTESIAN_POINT('Ctrl Pts',(56.2817103328366,-15.889189778178,4.96235566707568));
#40016=CARTESIAN_POINT('Ctrl Pts',(56.2783262011229,-15.6883461217826,5.));
#40017=CARTESIAN_POINT('Ctrl Pts',(56.2783262011229,-15.5,5.));
#40018=CARTESIAN_POINT('Origin',(74.,-14.,5.));
#40019=CARTESIAN_POINT('',(56.2783262011229,-14.,5.));
#40020=CARTESIAN_POINT('',(37.,-14.,5.));
#40021=CARTESIAN_POINT('',(56.2783262011229,-16.45,5.));
#40022=CARTESIAN_POINT('Origin',(0.,-12.3786796564404,0.));
#40023=CARTESIAN_POINT('',(-1.12667505521556E-14,-12.3786796564404,-92.));
#40024=CARTESIAN_POINT('Origin',(0.,-12.3786796564404,0.));
#40025=CARTESIAN_POINT('',(-1.12129469407189E-14,-13.4393398282202,-91.5606601717798));
#40026=CARTESIAN_POINT('Origin',(-1.10830535322835E-14,-12.3786796564404,
-90.5));
#40027=CARTESIAN_POINT('Origin',(-8.40971020553915E-15,-13.4393398282202,
0.));
#40028=CARTESIAN_POINT('Origin',(0.,-13.5,0.));
#40029=CARTESIAN_POINT('',(-1.11980894836777E-14,-13.5606601717798,-91.4393398282202));
#40030=CARTESIAN_POINT('',(-1.12055182121983E-14,-13.5,-91.5));
#40031=CARTESIAN_POINT('Origin',(-8.39856711275827E-15,-13.5606601717798,
0.));
#40032=CARTESIAN_POINT('Origin',(0.,-6.5,0.));
#40033=CARTESIAN_POINT('',(-1.12667505521556E-14,-1.5,-92.));
#40034=CARTESIAN_POINT('Origin',(0.,-1.5,0.));
#40035=CARTESIAN_POINT('',(-1.12667505521556E-14,-6.5,-92.));
#40036=CARTESIAN_POINT('Origin',(0.,-12.5,0.));
#40037=CARTESIAN_POINT('',(-1.10681960752424E-14,-14.,-90.3786796564403));
#40038=CARTESIAN_POINT('Origin',(-1.10681960752424E-14,-12.5,-90.3786796564403));
#40039=CARTESIAN_POINT('Origin',(0.,-14.,0.));
#40040=CARTESIAN_POINT('Origin',(0.,-14.,91.));
#40041=CARTESIAN_POINT('',(25.8800414539374,-14.,-75.7581216659255));
#40042=CARTESIAN_POINT('Origin',(31.3800414539374,-14.,-75.7581216659255));
#40043=CARTESIAN_POINT('',(-81.2581216659255,-14.,-31.3800414539373));
#40044=CARTESIAN_POINT('Origin',(-75.7581216659255,-14.,-31.3800414539373));
#40045=CARTESIAN_POINT('',(-81.2581216659255,-14.,31.3800414539374));
#40046=CARTESIAN_POINT('Origin',(-75.7581216659255,-14.,31.3800414539374));
#40047=CARTESIAN_POINT('',(25.8800414539374,-14.,75.7581216659255));
#40048=CARTESIAN_POINT('Origin',(31.3800414539374,-14.,75.7581216659255));
#40049=CARTESIAN_POINT('',(-36.8800414539374,-14.,75.7581216659255));
#40050=CARTESIAN_POINT('Origin',(-31.3800414539374,-14.,75.7581216659255));
#40051=CARTESIAN_POINT('',(70.2581216659255,-14.,31.3800414539374));
#40052=CARTESIAN_POINT('Origin',(75.7581216659255,-14.,31.3800414539374));
#40053=CARTESIAN_POINT('',(-36.8800414539373,-14.,-75.7581216659255));
#40054=CARTESIAN_POINT('Origin',(-31.3800414539373,-14.,-75.7581216659255));
#40055=CARTESIAN_POINT('',(70.2581216659255,-14.,-31.3800414539373));
#40056=CARTESIAN_POINT('Origin',(75.7581216659255,-14.,-31.3800414539373));
#40057=CARTESIAN_POINT('',(-5.00000000000001,-14.,-56.2783262011229));
#40058=CARTESIAN_POINT('',(-5.,-14.,20.5));
#40059=CARTESIAN_POINT('',(-56.2783262011229,-14.,-4.99999999999999));
#40060=CARTESIAN_POINT('Origin',(0.,-14.,0.));
#40061=CARTESIAN_POINT('',(-72.5,-14.,-4.99999999999998));
#40062=CARTESIAN_POINT('',(-37.,-14.,-4.99999999999998));
#40063=CARTESIAN_POINT('Origin',(-72.5,-14.,-3.49999999999999));
#40064=CARTESIAN_POINT('',(-56.2783262011229,-14.,5.00000000000001));
#40065=CARTESIAN_POINT('',(-25.,-14.,5.));
#40066=CARTESIAN_POINT('Origin',(0.,-14.,0.));
#40067=CARTESIAN_POINT('',(5.,-14.,56.2783262011229));
#40068=CARTESIAN_POINT('',(5.,-14.,70.5));
#40069=CARTESIAN_POINT('Origin',(0.,-14.,0.));
#40070=CARTESIAN_POINT('',(56.2783262011229,-14.,-5.));
#40071=CARTESIAN_POINT('',(25.,-14.,-5.));
#40072=CARTESIAN_POINT('Origin',(0.,-14.,0.));
#40073=CARTESIAN_POINT('Origin',(56.,-15.5,-3.5));
#40074=CARTESIAN_POINT('',(56.2783262011229,-15.5,-5.));
#40075=CARTESIAN_POINT('Ctrl Pts',(56.2783262011229,-15.5,-5.));
#40076=CARTESIAN_POINT('Ctrl Pts',(56.2783262011229,-15.6883461217826,-5.));
#40077=CARTESIAN_POINT('Ctrl Pts',(56.2817103328366,-15.889189778178,-4.96235566707568));
#40078=CARTESIAN_POINT('Ctrl Pts',(56.2949857165266,-16.2585410496607,-4.8094152373875));
#40079=CARTESIAN_POINT('Ctrl Pts',(56.3048219679644,-16.4270526075957,-4.69412389350913));
#40080=CARTESIAN_POINT('Ctrl Pts',(56.3263779287031,-16.6934822832211,-4.42798167302478));
#40081=CARTESIAN_POINT('Ctrl Pts',(56.3395353657988,-16.8090480003591,-4.25923828551909));
#40082=CARTESIAN_POINT('Ctrl Pts',(56.366268079425,-16.9623071985392,-3.88949595769795));
#40083=CARTESIAN_POINT('Ctrl Pts',(56.379789702144,-17.,-3.68849285843233));
#40084=CARTESIAN_POINT('Ctrl Pts',(56.3914887194867,-17.,-3.5));
#40085=CARTESIAN_POINT('',(56.,-15.5,-5.));
#40086=CARTESIAN_POINT('Origin',(50.,-14.,-5.));
#40087=CARTESIAN_POINT('',(56.2783262011229,-16.45,-5.));
#40088=CARTESIAN_POINT('Origin',(3.5,-15.5,56.));
#40089=CARTESIAN_POINT('',(5.,-15.5,56.2783262011229));
#40090=CARTESIAN_POINT('Ctrl Pts',(5.,-15.5,56.2783262011229));
#40091=CARTESIAN_POINT('Ctrl Pts',(5.,-15.6883461217826,56.2783262011229));
#40092=CARTESIAN_POINT('Ctrl Pts',(4.96235566707569,-15.889189778178,56.2817103328366));
#40093=CARTESIAN_POINT('Ctrl Pts',(4.8094152373875,-16.2585410496607,56.2949857165266));
#40094=CARTESIAN_POINT('Ctrl Pts',(4.69412389350913,-16.4270526075957,56.3048219679644));
#40095=CARTESIAN_POINT('Ctrl Pts',(4.42798167302478,-16.6934822832211,56.3263779287031));
#40096=CARTESIAN_POINT('Ctrl Pts',(4.25923828551909,-16.8090480003591,56.3395353657988));
#40097=CARTESIAN_POINT('Ctrl Pts',(3.88949595769795,-16.9623071985392,56.366268079425));
#40098=CARTESIAN_POINT('Ctrl Pts',(3.68849285843233,-17.,56.379789702144));
#40099=CARTESIAN_POINT('Ctrl Pts',(3.5,-17.,56.3914887194867));
#40100=CARTESIAN_POINT('',(5.,-15.5,56.));
#40101=CARTESIAN_POINT('Origin',(5.,-14.,50.));
#40102=CARTESIAN_POINT('',(5.,-16.45,56.2783262011229));
#40103=CARTESIAN_POINT('Origin',(0.,-1.5,0.));
#40104=CARTESIAN_POINT('',(-1.10830535322835E-14,0.,-90.5));
#40105=CARTESIAN_POINT('Origin',(0.,0.,0.));
#40106=CARTESIAN_POINT('Origin',(-1.10830535322835E-14,-1.5,-90.5));
#40107=CARTESIAN_POINT('Origin',(0.,0.,0.));
#40108=CARTESIAN_POINT('',(-70.9934791577936,0.,-28.6326460019314));
#40109=CARTESIAN_POINT('',(-70.9934791577936,0.,28.6326460019316));
#40110=CARTESIAN_POINT('Origin',(0.,0.,0.));
#40111=CARTESIAN_POINT('',(-81.2581216659255,0.,-31.3800414539373));
#40112=CARTESIAN_POINT('Origin',(-75.7581216659255,0.,-31.3800414539373));
#40113=CARTESIAN_POINT('',(-70.4463086837813,0.,-29.9536323812221));
#40114=CARTESIAN_POINT('Origin',(-75.7581216659255,0.,-31.3800414539373));
#40115=CARTESIAN_POINT('',(-29.9536323812221,0.,-70.4463086837813));
#40116=CARTESIAN_POINT('Origin',(0.,0.,0.));
#40117=CARTESIAN_POINT('',(-36.8800414539373,0.,-75.7581216659255));
#40118=CARTESIAN_POINT('Origin',(-31.3800414539373,0.,-75.7581216659255));
#40119=CARTESIAN_POINT('',(-28.6326460019314,0.,-70.9934791577936));
#40120=CARTESIAN_POINT('Origin',(-31.3800414539373,0.,-75.7581216659255));
#40121=CARTESIAN_POINT('',(28.6326460019314,0.,-70.9934791577936));
#40122=CARTESIAN_POINT('Origin',(0.,0.,0.));
#40123=CARTESIAN_POINT('',(25.8800414539374,0.,-75.7581216659255));
#40124=CARTESIAN_POINT('Origin',(31.3800414539374,0.,-75.7581216659255));
#40125=CARTESIAN_POINT('',(29.9536323812222,0.,-70.4463086837813));
#40126=CARTESIAN_POINT('Origin',(31.3800414539374,0.,-75.7581216659255));
#40127=CARTESIAN_POINT('',(70.4463086837813,0.,-29.9536323812221));
#40128=CARTESIAN_POINT('Origin',(0.,0.,0.));
#40129=CARTESIAN_POINT('',(70.2581216659255,0.,-31.3800414539373));
#40130=CARTESIAN_POINT('Origin',(75.7581216659255,0.,-31.3800414539373));
#40131=CARTESIAN_POINT('',(70.9934791577936,0.,-28.6326460019314));
#40132=CARTESIAN_POINT('Origin',(75.7581216659255,0.,-31.3800414539373));
#40133=CARTESIAN_POINT('',(70.9934791577936,0.,28.6326460019314));
#40134=CARTESIAN_POINT('Origin',(0.,0.,0.));
#40135=CARTESIAN_POINT('',(70.2581216659255,0.,31.3800414539374));
#40136=CARTESIAN_POINT('Origin',(75.7581216659255,0.,31.3800414539374));
#40137=CARTESIAN_POINT('',(70.4463086837813,0.,29.9536323812221));
#40138=CARTESIAN_POINT('Origin',(75.7581216659255,0.,31.3800414539374));
#40139=CARTESIAN_POINT('',(29.953632381222,0.,70.4463086837814));
#40140=CARTESIAN_POINT('Origin',(0.,0.,0.));
#40141=CARTESIAN_POINT('',(25.8800414539374,0.,75.7581216659255));
#40142=CARTESIAN_POINT('Origin',(31.3800414539374,0.,75.7581216659255));
#40143=CARTESIAN_POINT('',(28.6326460019316,0.,70.9934791577936));
#40144=CARTESIAN_POINT('Origin',(31.3800414539374,0.,75.7581216659255));
#40145=CARTESIAN_POINT('',(-9.37467124747299E-15,0.,76.55));
#40146=CARTESIAN_POINT('Origin',(0.,0.,0.));
#40147=CARTESIAN_POINT('',(-28.6326460019314,0.,70.9934791577936));
#40148=CARTESIAN_POINT('Origin',(0.,0.,0.));
#40149=CARTESIAN_POINT('',(-36.8800414539374,0.,75.7581216659255));
#40150=CARTESIAN_POINT('Origin',(-31.3800414539374,0.,75.7581216659255));
#40151=CARTESIAN_POINT('',(-29.9536323812221,0.,70.4463086837813));
#40152=CARTESIAN_POINT('Origin',(-31.3800414539374,0.,75.7581216659255));
#40153=CARTESIAN_POINT('',(-70.4463086837814,0.,29.953632381222));
#40154=CARTESIAN_POINT('Origin',(0.,0.,0.));
#40155=CARTESIAN_POINT('',(-81.2581216659255,0.,31.3800414539374));
#40156=CARTESIAN_POINT('Origin',(-75.7581216659255,0.,31.3800414539374));
#40157=CARTESIAN_POINT('Origin',(-75.7581216659255,0.,31.3800414539374));
#40158=CARTESIAN_POINT('Origin',(0.,-18.5,0.));
#40159=CARTESIAN_POINT('',(-6.85059334670459E-15,-19.5606601717798,-55.9393398282202));
#40160=CARTESIAN_POINT('Origin',(-5.13794501002844E-15,-19.5606601717798,
0.));
#40161=CARTESIAN_POINT('',(-6.72069993826926E-15,-20.,-54.8786796564404));
#40162=CARTESIAN_POINT('Origin',(-6.72069993826926E-15,-18.5,-54.8786796564404));
#40163=CARTESIAN_POINT('Origin',(0.,-20.,0.));
#40164=CARTESIAN_POINT('Origin',(0.,-19.5,0.));
#40165=CARTESIAN_POINT('',(-6.86545080374577E-15,-19.4393398282202,-56.0606601717798));
#40166=CARTESIAN_POINT('Origin',(-5.14908810280933E-15,-19.4393398282202,
0.));
#40167=CARTESIAN_POINT('',(-6.85802207522518E-15,-19.5,-56.));
#40168=CARTESIAN_POINT('Origin',(0.,-20.,55.5));
#40169=CARTESIAN_POINT('',(-4.34959053993225,-20.,-4.15347838401794));
#40170=CARTESIAN_POINT('',(-6.39699831604958,-20.,-3.79740738868713));
#40171=CARTESIAN_POINT('Ctrl Pts',(-4.34959053993225,-20.,-4.15347838401794));
#40172=CARTESIAN_POINT('Ctrl Pts',(-5.57128190994263,-20.,-4.15347838401794));
#40173=CARTESIAN_POINT('Ctrl Pts',(-6.39699831604958,-20.,-3.79740738868713));
#40174=CARTESIAN_POINT('',(-7.69235968589783,-20.,-2.72612595558167));
#40175=CARTESIAN_POINT('Ctrl Pts',(-6.39699831604958,-20.,-3.79740738868713));
#40176=CARTESIAN_POINT('Ctrl Pts',(-7.2227144241333,-20.,-3.44133758544922));
#40177=CARTESIAN_POINT('Ctrl Pts',(-7.69235968589783,-20.,-2.72612595558167));
#40178=CARTESIAN_POINT('',(-8.18656161427498,-20.,-1.10845828056335));
#40179=CARTESIAN_POINT('Ctrl Pts',(-7.69235968589783,-20.,-2.72612595558167));
#40180=CARTESIAN_POINT('Ctrl Pts',(-8.16200498491526,-20.,-2.01091432571411));
#40181=CARTESIAN_POINT('Ctrl Pts',(-8.18656161427498,-20.,-1.10845828056335));
#40182=CARTESIAN_POINT('',(-7.06309646368027,-20.,-1.0102322101593));
#40183=CARTESIAN_POINT('',(-1.66843011664469,-20.,-0.538569269720264));
#40184=CARTESIAN_POINT('',(-6.69167771935463,-20.,-2.11834931373596));
#40185=CARTESIAN_POINT('Ctrl Pts',(-7.06309646368027,-20.,-1.0102322101593));
#40186=CARTESIAN_POINT('Ctrl Pts',(-6.98328748345375,-20.,-1.68553912639618));
#40187=CARTESIAN_POINT('Ctrl Pts',(-6.69167771935463,-20.,-2.11834931373596));
#40188=CARTESIAN_POINT('',(-5.78615248203278,-20.,-2.81821274757385));
#40189=CARTESIAN_POINT('Ctrl Pts',(-6.69167771935463,-20.,-2.11834931373596));
#40190=CARTESIAN_POINT('Ctrl Pts',(-6.4000678062439,-20.,-2.55115950107574));
#40191=CARTESIAN_POINT('Ctrl Pts',(-5.78615248203278,-20.,-2.81821274757385));
#40192=CARTESIAN_POINT('',(-4.40484285354614,-20.,-3.08526659011841));
#40193=CARTESIAN_POINT('Ctrl Pts',(-5.78615248203278,-20.,-2.81821274757385));
#40194=CARTESIAN_POINT('Ctrl Pts',(-5.17223715782166,-20.,-3.08526659011841));
#40195=CARTESIAN_POINT('Ctrl Pts',(-4.40484285354614,-20.,-3.08526659011841));
#40196=CARTESIAN_POINT('',(-3.20156872272491,-20.,-2.88267397880554));
#40197=CARTESIAN_POINT('Ctrl Pts',(-4.40484285354614,-20.,-3.08526659011841));
#40198=CARTESIAN_POINT('Ctrl Pts',(-3.7233966588974,-20.,-3.08526659011841));
#40199=CARTESIAN_POINT('Ctrl Pts',(-3.20156872272491,-20.,-2.88267397880554));
#40200=CARTESIAN_POINT('',(-2.4249655008316,-20.,-2.32708060741425));
#40201=CARTESIAN_POINT('Ctrl Pts',(-3.20156872272491,-20.,-2.88267397880554));
#40202=CARTESIAN_POINT('Ctrl Pts',(-2.67974019050598,-20.,-2.68008136749268));
#40203=CARTESIAN_POINT('Ctrl Pts',(-2.4249655008316,-20.,-2.32708060741425));
#40204=CARTESIAN_POINT('',(-2.17019081115723,-20.,-1.5566166639328));
#40205=CARTESIAN_POINT('Ctrl Pts',(-2.4249655008316,-20.,-2.32708060741425));
#40206=CARTESIAN_POINT('Ctrl Pts',(-2.17019081115723,-20.,-1.97407925128937));
#40207=CARTESIAN_POINT('Ctrl Pts',(-2.17019081115723,-20.,-1.5566166639328));
#40208=CARTESIAN_POINT('',(-2.41575658321381,-20.,-0.816848516464234));
#40209=CARTESIAN_POINT('Ctrl Pts',(-2.17019081115723,-20.,-1.5566166639328));
#40210=CARTESIAN_POINT('Ctrl Pts',(-2.17019081115723,-20.,-1.13301539421082));
#40211=CARTESIAN_POINT('Ctrl Pts',(-2.41575658321381,-20.,-0.816848516464234));
#40212=CARTESIAN_POINT('',(-3.22612524032593,-20.,-0.28581166267395));
#40213=CARTESIAN_POINT('Ctrl Pts',(-2.41575658321381,-20.,-0.816848516464234));
#40214=CARTESIAN_POINT('Ctrl Pts',(-2.66132295131683,-20.,-0.500682830810547));
#40215=CARTESIAN_POINT('Ctrl Pts',(-3.22612524032593,-20.,-0.28581166267395));
#40216=CARTESIAN_POINT('',(-4.82844471931458,-20.,0.15313720703125));
#40217=CARTESIAN_POINT('Ctrl Pts',(-3.22612524032593,-20.,-0.28581166267395));
#40218=CARTESIAN_POINT('Ctrl Pts',(-3.5883355140686,-20.,-0.144611835479737));
#40219=CARTESIAN_POINT('Ctrl Pts',(-4.82844471931458,-20.,0.15313720703125));
#40220=CARTESIAN_POINT('',(-6.5658250451088,-20.,0.714870452880859));
#40221=CARTESIAN_POINT('Ctrl Pts',(-4.82844471931458,-20.,0.15313720703125));
#40222=CARTESIAN_POINT('Ctrl Pts',(-6.0685533285141,-20.,0.450886249542236));
#40223=CARTESIAN_POINT('Ctrl Pts',(-6.5658250451088,-20.,0.714870452880859));
#40224=CARTESIAN_POINT('',(-7.52660259604454,-20.,1.55286467075348));
#40225=CARTESIAN_POINT('Ctrl Pts',(-6.5658250451088,-20.,0.714870452880859));
#40226=CARTESIAN_POINT('Ctrl Pts',(-7.21043616533279,-20.,1.05252361297607));
#40227=CARTESIAN_POINT('Ctrl Pts',(-7.52660259604454,-20.,1.55286467075348));
#40228=CARTESIAN_POINT('',(-7.84276902675629,-20.,2.67326033115387));
#40229=CARTESIAN_POINT('Ctrl Pts',(-7.52660259604454,-20.,1.55286467075348));
#40230=CARTESIAN_POINT('Ctrl Pts',(-7.84276902675629,-20.,2.05320572853088));
#40231=CARTESIAN_POINT('Ctrl Pts',(-7.84276902675629,-20.,2.67326033115387));
#40232=CARTESIAN_POINT('',(-7.4560022354126,-20.,3.9471343755722));
#40233=CARTESIAN_POINT('Ctrl Pts',(-7.84276902675629,-20.,2.67326033115387));
#40234=CARTESIAN_POINT('Ctrl Pts',(-7.84276902675629,-20.,3.35470592975616));
#40235=CARTESIAN_POINT('Ctrl Pts',(-7.4560022354126,-20.,3.9471343755722));
#40236=CARTESIAN_POINT('',(-6.32639795541763,-20.,4.84652078151703));
#40237=CARTESIAN_POINT('Ctrl Pts',(-7.4560022354126,-20.,3.9471343755722));
#40238=CARTESIAN_POINT('Ctrl Pts',(-7.06923559308052,-20.,4.53956282138824));
#40239=CARTESIAN_POINT('Ctrl Pts',(-6.32639795541763,-20.,4.84652078151703));
#40240=CARTESIAN_POINT('',(-4.67496573925018,-20.,5.15347814559937));
#40241=CARTESIAN_POINT('Ctrl Pts',(-6.32639795541763,-20.,4.84652078151703));
#40242=CARTESIAN_POINT('Ctrl Pts',(-5.58356046676636,-20.,5.15347814559937));
#40243=CARTESIAN_POINT('Ctrl Pts',(-4.67496573925018,-20.,5.15347814559937));
#40244=CARTESIAN_POINT('',(-2.90995895862579,-20.,4.83117258548737));
#40245=CARTESIAN_POINT('Ctrl Pts',(-4.67496573925018,-20.,5.15347814559937));
#40246=CARTESIAN_POINT('Ctrl Pts',(-3.67428362369537,-20.,5.15347814559937));
#40247=CARTESIAN_POINT('Ctrl Pts',(-2.90995895862579,-20.,4.83117258548737));
#40248=CARTESIAN_POINT('',(-1.73431098461151,-20.,3.88267314434052));
#40249=CARTESIAN_POINT('Ctrl Pts',(-2.90995895862579,-20.,4.83117258548737));
#40250=CARTESIAN_POINT('Ctrl Pts',(-2.14563429355621,-20.,4.50886702537537));
#40251=CARTESIAN_POINT('Ctrl Pts',(-1.73431098461151,-20.,3.88267314434052));
#40252=CARTESIAN_POINT('',(-1.29229187965393,-20.,2.46452903747559));
#40253=CARTESIAN_POINT('Ctrl Pts',(-1.73431098461151,-20.,3.88267314434052));
#40254=CARTESIAN_POINT('Ctrl Pts',(-1.32298767566681,-20.,3.25647985935211));
#40255=CARTESIAN_POINT('Ctrl Pts',(-1.29229187965393,-20.,2.46452903747559));
#40256=CARTESIAN_POINT('',(-2.4341744184494,-20.,2.37858092784882));
#40257=CARTESIAN_POINT('',(1.33492752978397,-20.,2.6622766464846));
#40258=CARTESIAN_POINT('',(-3.05729866027832,-20.,3.66780316829681));
#40259=CARTESIAN_POINT('Ctrl Pts',(-2.4341744184494,-20.,2.37858092784882));
#40260=CARTESIAN_POINT('Ctrl Pts',(-2.52626180648804,-20.,3.2319233417511));
#40261=CARTESIAN_POINT('Ctrl Pts',(-3.05729866027832,-20.,3.66780316829681));
#40262=CARTESIAN_POINT('',(-4.62585210800171,-20.,4.10368299484253));
#40263=CARTESIAN_POINT('Ctrl Pts',(-3.05729866027832,-20.,3.66780316829681));
#40264=CARTESIAN_POINT('Ctrl Pts',(-3.5883355140686,-20.,4.10368299484253));
#40265=CARTESIAN_POINT('Ctrl Pts',(-4.62585210800171,-20.,4.10368299484253));
#40266=CARTESIAN_POINT('',(-6.20054543018341,-20.,3.70770728588104));
#40267=CARTESIAN_POINT('Ctrl Pts',(-4.62585210800171,-20.,4.10368299484253));
#40268=CARTESIAN_POINT('Ctrl Pts',(-5.70634365081787,-20.,4.10368299484253));
#40269=CARTESIAN_POINT('Ctrl Pts',(-6.20054543018341,-20.,3.70770728588104));
#40270=CARTESIAN_POINT('',(-6.69474720954895,-20.,2.75306916236877));
#40271=CARTESIAN_POINT('Ctrl Pts',(-6.20054543018341,-20.,3.70770728588104));
#40272=CARTESIAN_POINT('Ctrl Pts',(-6.69474720954895,-20.,3.311732172966));
#40273=CARTESIAN_POINT('Ctrl Pts',(-6.69474720954895,-20.,2.75306916236877));
#40274=CARTESIAN_POINT('',(-6.34481549263,-20.,1.95497906208038));
#40275=CARTESIAN_POINT('Ctrl Pts',(-6.69474720954895,-20.,2.75306916236877));
#40276=CARTESIAN_POINT('Ctrl Pts',(-6.69474720954895,-20.,2.26807570457458));
#40277=CARTESIAN_POINT('Ctrl Pts',(-6.34481549263,-20.,1.95497906208038));
#40278=CARTESIAN_POINT('',(-4.54911291599274,-20.,1.31343758106232));
#40279=CARTESIAN_POINT('Ctrl Pts',(-6.34481549263,-20.,1.95497906208038));
#40280=CARTESIAN_POINT('Ctrl Pts',(-6.00102305412292,-20.,1.64188241958618));
#40281=CARTESIAN_POINT('Ctrl Pts',(-4.54911291599274,-20.,1.31343758106232));
#40282=CARTESIAN_POINT('',(-2.55695760250092,-20.,0.739426374435425));
#40283=CARTESIAN_POINT('Ctrl Pts',(-4.54911291599274,-20.,1.31343758106232));
#40284=CARTESIAN_POINT('Ctrl Pts',(-3.09720277786255,-20.,0.984992742538452));
#40285=CARTESIAN_POINT('Ctrl Pts',(-2.55695760250092,-20.,0.739426374435425));
#40286=CARTESIAN_POINT('',(-1.39665722846985,-20.,-0.1783766746521));
#40287=CARTESIAN_POINT('Ctrl Pts',(-2.55695760250092,-20.,0.739426374435425));
#40288=CARTESIAN_POINT('Ctrl Pts',(-1.77114546298981,-20.,0.377216696739197));
#40289=CARTESIAN_POINT('Ctrl Pts',(-1.39665722846985,-20.,-0.1783766746521));
#40290=CARTESIAN_POINT('',(-1.02216899394989,-20.,-1.4583899974823));
#40291=CARTESIAN_POINT('Ctrl Pts',(-1.39665722846985,-20.,-0.1783766746521));
#40292=CARTESIAN_POINT('Ctrl Pts',(-1.02216899394989,-20.,-0.733970642089844));
#40293=CARTESIAN_POINT('Ctrl Pts',(-1.02216899394989,-20.,-1.4583899974823));
#40294=CARTESIAN_POINT('',(-1.43349230289459,-20.,-2.81207346916199));
#40295=CARTESIAN_POINT('Ctrl Pts',(-1.02216899394989,-20.,-1.4583899974823));
#40296=CARTESIAN_POINT('Ctrl Pts',(-1.02216899394989,-20.,-2.17667126655579));
#40297=CARTESIAN_POINT('Ctrl Pts',(-1.43349230289459,-20.,-2.81207346916199));
#40298=CARTESIAN_POINT('',(-2.61527955532074,-20.,-3.80047702789307));
#40299=CARTESIAN_POINT('Ctrl Pts',(-1.43349230289459,-20.,-2.81207346916199));
#40300=CARTESIAN_POINT('Ctrl Pts',(-1.84481561183929,-20.,-3.44747567176819));
#40301=CARTESIAN_POINT('Ctrl Pts',(-2.61527955532074,-20.,-3.80047702789307));
#40302=CARTESIAN_POINT('Ctrl Pts',(-2.61527955532074,-20.,-3.80047702789307));
#40303=CARTESIAN_POINT('Ctrl Pts',(-3.38574349880219,-20.,-4.15347838401794));
#40304=CARTESIAN_POINT('Ctrl Pts',(-4.34959053993225,-20.,-4.15347838401794));
#40305=CARTESIAN_POINT('',(25.4253059625626,-20.,4.99999976158142));
#40306=CARTESIAN_POINT('',(21.833900809288,-20.,-0.187585592269898));
#40307=CARTESIAN_POINT('',(33.1234064883977,-20.,16.1194785828128));
#40308=CARTESIAN_POINT('',(21.833900809288,-20.,-4.));
#40309=CARTESIAN_POINT('',(21.833900809288,-20.,27.656207203865));
#40310=CARTESIAN_POINT('',(20.6429049372673,-20.,-4.));
#40311=CARTESIAN_POINT('',(10.916950404644,-20.,-4.));
#40312=CARTESIAN_POINT('',(20.6429049372673,-20.,-0.187585592269898));
#40313=CARTESIAN_POINT('',(20.6429049372673,-20.,25.75));
#40314=CARTESIAN_POINT('',(17.1742831147276,-20.,4.99999976158142));
#40315=CARTESIAN_POINT('',(4.58852554825927,-20.,23.8229487480263));
#40316=CARTESIAN_POINT('',(18.6231234669685,-20.,4.99999976158142));
#40317=CARTESIAN_POINT('',(8.58714155736379,-20.,4.99999976158142));
#40318=CARTESIAN_POINT('',(20.3973388671875,-20.,2.28649353981018));
#40319=CARTESIAN_POINT('',(4.2691955553234,-20.,26.9530685323169));
#40320=CARTESIAN_POINT('',(21.3120725750923,-20.,0.763983488082886));
#40321=CARTESIAN_POINT('Ctrl Pts',(20.3973388671875,-20.,2.28649353981018));
#40322=CARTESIAN_POINT('Ctrl Pts',(20.8884710073471,-20.,1.52523851394653));
#40323=CARTESIAN_POINT('Ctrl Pts',(21.3120725750923,-20.,0.763983488082886));
#40324=CARTESIAN_POINT('',(22.2943377494812,-20.,2.3540244102478));
#40325=CARTESIAN_POINT('Ctrl Pts',(21.3120725750923,-20.,0.763983488082886));
#40326=CARTESIAN_POINT('Ctrl Pts',(21.7172569036484,-20.,1.46998620033264));
#40327=CARTESIAN_POINT('Ctrl Pts',(22.2943377494812,-20.,2.3540244102478));
#40328=CARTESIAN_POINT('',(24.0378570556641,-20.,4.99999976158142));
#40329=CARTESIAN_POINT('',(31.1284359424709,-20.,15.7607047877004));
#40330=CARTESIAN_POINT('',(12.018928527832,-20.,4.99999976158142));
#40331=CARTESIAN_POINT('',(-25.6470237061142,-20.,4.99999976158142));
#40332=CARTESIAN_POINT('',(-18.0214869976044,-20.,4.99999976158142));
#40333=CARTESIAN_POINT('',(-12.2644948586822,-20.,4.99999976158142));
#40334=CARTESIAN_POINT('',(-18.0214869976044,-20.,3.93792605400085));
#40335=CARTESIAN_POINT('',(-18.0214869976044,-20.,30.2499998807907));
#40336=CARTESIAN_POINT('',(-23.3379939198494,-20.,3.93792605400085));
#40337=CARTESIAN_POINT('',(-9.01074349880219,-20.,3.93792605400085));
#40338=CARTESIAN_POINT('',(-23.3379939198494,-20.,1.18144607543945));
#40339=CARTESIAN_POINT('',(-23.3379939198494,-20.,29.7189630270004));
#40340=CARTESIAN_POINT('',(-18.3591401576996,-20.,1.18144607543945));
#40341=CARTESIAN_POINT('',(-11.6689969599247,-20.,1.18144607543945));
#40342=CARTESIAN_POINT('',(-18.3591401576996,-20.,0.125511646270752));
#40343=CARTESIAN_POINT('',(-18.3591401576996,-20.,28.3407230377197));
#40344=CARTESIAN_POINT('',(-23.3379939198494,-20.,0.125511646270752));
#40345=CARTESIAN_POINT('',(-9.17957007884979,-20.,0.125511646270748));
#40346=CARTESIAN_POINT('',(-23.3379939198494,-20.,-2.93792629241943));
#40347=CARTESIAN_POINT('',(-23.3379939198494,-20.,27.8127558231354));
#40348=CARTESIAN_POINT('',(-17.8127557039261,-20.,-2.93792629241943));
#40349=CARTESIAN_POINT('',(-11.6689969599247,-20.,-2.93792629241944));
#40350=CARTESIAN_POINT('',(-17.8127557039261,-20.,-4.));
#40351=CARTESIAN_POINT('',(-17.8127557039261,-20.,26.2810368537903));
#40352=CARTESIAN_POINT('',(-25.6470237061142,-20.,-4.));
#40353=CARTESIAN_POINT('',(-8.90637785196304,-20.,-4.));
#40354=CARTESIAN_POINT('',(-25.6470237061142,-20.,-4.));
#40355=CARTESIAN_POINT('',(-17.3346091195702,-20.,4.99999976158142));
#40356=CARTESIAN_POINT('',(-12.8400406241417,-20.,4.99999976158142));
#40357=CARTESIAN_POINT('',(-8.10828756541014,-20.,4.99999976158142));
#40358=CARTESIAN_POINT('',(-11.1855381727219,-20.,4.72680723667145));
#40359=CARTESIAN_POINT('Ctrl Pts',(-12.8400406241417,-20.,4.99999976158142));
#40360=CARTESIAN_POINT('Ctrl Pts',(-11.8086624145508,-20.,4.99999976158142));
#40361=CARTESIAN_POINT('Ctrl Pts',(-11.1855381727219,-20.,4.72680723667145));
#40362=CARTESIAN_POINT('',(-10.2094125747681,-20.,3.8857433795929));
#40363=CARTESIAN_POINT('Ctrl Pts',(-11.1855381727219,-20.,4.72680723667145));
#40364=CARTESIAN_POINT('Ctrl Pts',(-10.5624139308929,-20.,4.45361471176147));
#40365=CARTESIAN_POINT('Ctrl Pts',(-10.2094125747681,-20.,3.8857433795929));
#40366=CARTESIAN_POINT('',(-9.85641181468963,-20.,2.69781684875488));
#40367=CARTESIAN_POINT('Ctrl Pts',(-10.2094125747681,-20.,3.8857433795929));
#40368=CARTESIAN_POINT('Ctrl Pts',(-9.85641181468963,-20.,3.31787145137787));
#40369=CARTESIAN_POINT('Ctrl Pts',(-9.85641181468963,-20.,2.69781684875488));
#40370=CARTESIAN_POINT('',(-10.1695084571838,-20.,1.6111866235733));
#40371=CARTESIAN_POINT('Ctrl Pts',(-9.85641181468963,-20.,2.69781684875488));
#40372=CARTESIAN_POINT('Ctrl Pts',(-9.85641181468963,-20.,2.12073659896851));
#40373=CARTESIAN_POINT('Ctrl Pts',(-10.1695084571838,-20.,1.6111866235733));
#40374=CARTESIAN_POINT('',(-11.1149382591248,-20.,0.788540005683899));
#40375=CARTESIAN_POINT('Ctrl Pts',(-10.1695084571838,-20.,1.6111866235733));
#40376=CARTESIAN_POINT('Ctrl Pts',(-10.482605099678,-20.,1.1016366481781));
#40377=CARTESIAN_POINT('Ctrl Pts',(-11.1149382591248,-20.,0.788540005683899));
#40378=CARTESIAN_POINT('',(-9.85948085784912,-20.,-0.0279673337936404));
#40379=CARTESIAN_POINT('Ctrl Pts',(-11.1149382591248,-20.,0.788540005683899));
#40380=CARTESIAN_POINT('Ctrl Pts',(-10.2984303236008,-20.,0.549112915992737));
#40381=CARTESIAN_POINT('Ctrl Pts',(-9.85948085784912,-20.,-0.0279673337936404));
#40382=CARTESIAN_POINT('',(-9.42053139209747,-20.,-1.39085972309113));
#40383=CARTESIAN_POINT('Ctrl Pts',(-9.85948085784912,-20.,-0.0279673337936404));
#40384=CARTESIAN_POINT('Ctrl Pts',(-9.42053139209747,-20.,-0.605048179626465));
#40385=CARTESIAN_POINT('Ctrl Pts',(-9.42053139209747,-20.,-1.39085972309113));
#40386=CARTESIAN_POINT('',(-9.68758463859558,-20.,-2.56650769710541));
#40387=CARTESIAN_POINT('Ctrl Pts',(-9.42053139209747,-20.,-1.39085972309113));
#40388=CARTESIAN_POINT('Ctrl Pts',(-9.42053139209747,-20.,-2.02319228649139));
#40389=CARTESIAN_POINT('Ctrl Pts',(-9.68758463859558,-20.,-2.56650769710541));
#40390=CARTESIAN_POINT('',(-10.3475439548492,-20.,-3.40450191497803));
#40391=CARTESIAN_POINT('Ctrl Pts',(-9.68758463859558,-20.,-2.56650769710541));
#40392=CARTESIAN_POINT('Ctrl Pts',(-9.95463788509369,-20.,-3.10982251167297));
#40393=CARTESIAN_POINT('Ctrl Pts',(-10.3475439548492,-20.,-3.40450191497803));
#40394=CARTESIAN_POINT('',(-11.3328778743744,-20.,-3.84959125518799));
#40395=CARTESIAN_POINT('Ctrl Pts',(-10.3475439548492,-20.,-3.40450191497803));
#40396=CARTESIAN_POINT('Ctrl Pts',(-10.7404494285583,-20.,-3.69918131828308));
#40397=CARTESIAN_POINT('Ctrl Pts',(-11.3328778743744,-20.,-3.84959125518799));
#40398=CARTESIAN_POINT('',(-12.7847883105278,-20.,-4.));
#40399=CARTESIAN_POINT('Ctrl Pts',(-11.3328778743744,-20.,-3.84959125518799));
#40400=CARTESIAN_POINT('Ctrl Pts',(-11.9253063201904,-20.,-4.));
#40401=CARTESIAN_POINT('Ctrl Pts',(-12.7847883105278,-20.,-4.));
#40402=CARTESIAN_POINT('',(-17.3346091195702,-20.,-4.));
#40403=CARTESIAN_POINT('',(-6.3923941552639,-20.,-4.));
#40404=CARTESIAN_POINT('',(-17.3346091195702,-20.,-4.));
#40405=CARTESIAN_POINT('',(-0.494909523403555,-20.,4.99999976158142));
#40406=CARTESIAN_POINT('',(4.61357444524765,-20.,4.99999976158142));
#40407=CARTESIAN_POINT('',(0.31156223267317,-20.,4.99999976158142));
#40408=CARTESIAN_POINT('',(6.44304215908051,-20.,4.75750303268433));
#40409=CARTESIAN_POINT('Ctrl Pts',(4.61357444524765,-20.,4.99999976158142));
#40410=CARTESIAN_POINT('Ctrl Pts',(5.81684827804566,-20.,4.99999976158142));
#40411=CARTESIAN_POINT('Ctrl Pts',(6.44304215908051,-20.,4.75750303268433));
#40412=CARTESIAN_POINT('',(7.44372427463532,-20.,3.90109097957611));
#40413=CARTESIAN_POINT('Ctrl Pts',(6.44304215908051,-20.,4.75750303268433));
#40414=CARTESIAN_POINT('Ctrl Pts',(7.06923604011536,-20.,4.51500630378723));
#40415=CARTESIAN_POINT('Ctrl Pts',(7.44372427463532,-20.,3.90109097957611));
#40416=CARTESIAN_POINT('',(7.81821250915528,-20.,2.54433786869049));
#40417=CARTESIAN_POINT('Ctrl Pts',(7.44372427463532,-20.,3.90109097957611));
#40418=CARTESIAN_POINT('Ctrl Pts',(7.81821250915528,-20.,3.28717565536499));
#40419=CARTESIAN_POINT('Ctrl Pts',(7.81821250915528,-20.,2.54433786869049));
#40420=CARTESIAN_POINT('',(7.19815790653229,-20.,0.92974042892456));
#40421=CARTESIAN_POINT('Ctrl Pts',(7.81821250915528,-20.,2.54433786869049));
#40422=CARTESIAN_POINT('Ctrl Pts',(7.81821250915528,-20.,1.58663010597229));
#40423=CARTESIAN_POINT('Ctrl Pts',(7.19815790653229,-20.,0.92974042892456));
#40424=CARTESIAN_POINT('',(5.28274238109589,-20.,0.0948152542114256));
#40425=CARTESIAN_POINT('Ctrl Pts',(7.19815790653229,-20.,0.92974042892456));
#40426=CARTESIAN_POINT('Ctrl Pts',(6.57810330390931,-20.,0.272850751876831));
#40427=CARTESIAN_POINT('Ctrl Pts',(5.28274238109589,-20.,0.0948152542114256));
#40428=CARTESIAN_POINT('',(6.00102305412293,-20.,-0.353342533111572));
#40429=CARTESIAN_POINT('Ctrl Pts',(5.28274238109589,-20.,0.0948152542114256));
#40430=CARTESIAN_POINT('Ctrl Pts',(5.7554566860199,-20.,-0.132333278656006));
#40431=CARTESIAN_POINT('Ctrl Pts',(6.00102305412293,-20.,-0.353342533111572));
#40432=CARTESIAN_POINT('',(6.98942661285401,-20.,-1.55047798156738));
#40433=CARTESIAN_POINT('Ctrl Pts',(6.00102305412293,-20.,-0.353342533111572));
#40434=CARTESIAN_POINT('Ctrl Pts',(6.52285099029541,-20.,-0.832196712493897));
#40435=CARTESIAN_POINT('Ctrl Pts',(6.98942661285401,-20.,-1.55047798156738));
#40436=CARTESIAN_POINT('',(7.89500652006261,-20.,-2.96744382018624));
#40437=CARTESIAN_POINT('',(-6.96767281131813,-20.,20.2882718988485));
#40438=CARTESIAN_POINT('',(10.9548091465744,-20.,4.99999976158142));
#40439=CARTESIAN_POINT('',(7.65239799219948,-20.,-3.5991740309707));
#40440=CARTESIAN_POINT('',(14.6435883014006,-20.,4.99999976158142));
#40441=CARTESIAN_POINT('',(6.07622772455216,-20.,4.99999976158142));
#40442=CARTESIAN_POINT('',(18.3270808427138,-20.,-4.));
#40443=CARTESIAN_POINT('',(14.4702638890185,-20.,5.42348905947456));
#40444=CARTESIAN_POINT('',(15.762277841568,-20.,-4.));
#40445=CARTESIAN_POINT('',(8.55951547622681,-20.,-4.));
#40446=CARTESIAN_POINT('',(14.7124826908112,-20.,-1.27421581745148));
#40447=CARTESIAN_POINT('',(4.76650014291145,-20.,24.5504432976375));
#40448=CARTESIAN_POINT('',(10.9491813182831,-20.,-1.27421581745148));
#40449=CARTESIAN_POINT('',(7.35624134540558,-20.,-1.27421581745148));
#40450=CARTESIAN_POINT('',(9.96077753603459,-20.,-4.));
#40451=CARTESIAN_POINT('',(19.410324588737,-20.,22.0596189038341));
#40452=CARTESIAN_POINT('',(7.05695748329163,-20.,-4.));
#40453=CARTESIAN_POINT('',(4.27745550870896,-20.,-4.));
#40454=CARTESIAN_POINT('',(5.86596190929413,-20.,-2.12755823135376));
#40455=CARTESIAN_POINT('',(-7.43172077059746,-20.,18.7785954266824));
#40456=CARTESIAN_POINT('',(5.00648021697998,-20.,-0.887449026107788));
#40457=CARTESIAN_POINT('Ctrl Pts',(5.86596190929413,-20.,-2.12755823135376));
#40458=CARTESIAN_POINT('Ctrl Pts',(5.34413397312165,-20.,-1.31719017028809));
#40459=CARTESIAN_POINT('Ctrl Pts',(5.00648021697998,-20.,-0.887449026107788));
#40460=CARTESIAN_POINT('',(4.40177381038666,-20.,-0.28581166267395));
#40461=CARTESIAN_POINT('Ctrl Pts',(5.00648021697998,-20.,-0.887449026107788));
#40462=CARTESIAN_POINT('Ctrl Pts',(4.66882705688477,-20.,-0.45770788192749));
#40463=CARTESIAN_POINT('Ctrl Pts',(4.40177381038666,-20.,-0.28581166267395));
#40464=CARTESIAN_POINT('',(3.85845869779587,-20.,-0.0463845729827883));
#40465=CARTESIAN_POINT('Ctrl Pts',(4.40177381038666,-20.,-0.28581166267395));
#40466=CARTESIAN_POINT('Ctrl Pts',(4.13472056388855,-20.,-0.11391544342041));
#40467=CARTESIAN_POINT('Ctrl Pts',(3.85845869779587,-20.,-0.0463845729827883));
#40468=CARTESIAN_POINT('',(3.1954300403595,-20.,-0.00341081619262718));
#40469=CARTESIAN_POINT('Ctrl Pts',(3.85845869779587,-20.,-0.0463845729827883));
#40470=CARTESIAN_POINT('Ctrl Pts',(3.65586668252945,-20.,-0.00341081619262718));
#40471=CARTESIAN_POINT('Ctrl Pts',(3.1954300403595,-20.,-0.00341081619262718));
#40472=CARTESIAN_POINT('',(1.81412041187287,-20.,-0.00341081619262718));
#40473=CARTESIAN_POINT('',(1.59771502017975,-20.,-0.00341081619263051));
#40474=CARTESIAN_POINT('',(1.81412041187287,-20.,-4.));
#40475=CARTESIAN_POINT('',(1.81412041187287,-20.,27.7482945919037));
#40476=CARTESIAN_POINT('',(-0.494909523403555,-20.,-4.));
#40477=CARTESIAN_POINT('',(0.907060205936434,-20.,-4.));
#40478=CARTESIAN_POINT('',(-0.494909523403555,-20.,-4.));
#40479=CARTESIAN_POINT('Origin',(-56.,-15.5,3.50000000000001));
#40480=CARTESIAN_POINT('',(-56.2783262011229,-15.5,5.00000000000001));
#40481=CARTESIAN_POINT('Ctrl Pts',(-56.2783262011229,-15.5,5.00000000000001));
#40482=CARTESIAN_POINT('Ctrl Pts',(-56.2783262011229,-15.6883461217826,
5.00000000000001));
#40483=CARTESIAN_POINT('Ctrl Pts',(-56.2817103328366,-15.889189778178,4.96235566707569));
#40484=CARTESIAN_POINT('Ctrl Pts',(-56.2949857165266,-16.2585410496607,
4.80941523738751));
#40485=CARTESIAN_POINT('Ctrl Pts',(-56.3048219679644,-16.4270526075957,
4.69412389350914));
#40486=CARTESIAN_POINT('Ctrl Pts',(-56.3263779287031,-16.6934822832211,
4.42798167302479));
#40487=CARTESIAN_POINT('Ctrl Pts',(-56.3395353657988,-16.8090480003591,
4.25923828551909));
#40488=CARTESIAN_POINT('Ctrl Pts',(-56.366268079425,-16.9623071985392,3.88949595769795));
#40489=CARTESIAN_POINT('Ctrl Pts',(-56.379789702144,-17.,3.68849285843234));
#40490=CARTESIAN_POINT('Ctrl Pts',(-56.3914887194867,-17.,3.50000000000001));
#40491=CARTESIAN_POINT('',(-56.,-15.5,5.00000000000001));
#40492=CARTESIAN_POINT('Origin',(-72.5,-14.,-3.49999999999999));
#40493=CARTESIAN_POINT('',(-72.5,-15.5,-4.99999999999999));
#40494=CARTESIAN_POINT('Origin',(-72.5,-15.5,-3.49999999999999));
#40495=CARTESIAN_POINT('',(-72.5,-14.,-4.99999999999999));
#40496=CARTESIAN_POINT('Origin',(-72.5,-15.5,-3.49999999999999));
#40497=CARTESIAN_POINT('Origin',(-72.5,-15.5,-3.49999999999999));
#40498=CARTESIAN_POINT('Origin',(-68.,-15.5,-3.49999999999999));
#40499=CARTESIAN_POINT('',(-56.2783262011229,-15.5,-4.99999999999999));
#40500=CARTESIAN_POINT('',(-68.,-15.5,-4.99999999999999));
#40501=CARTESIAN_POINT('Ctrl Pts',(-56.3914887194867,-17.,-3.49999999999999));
#40502=CARTESIAN_POINT('Ctrl Pts',(-56.379789702144,-17.,-3.68849285843232));
#40503=CARTESIAN_POINT('Ctrl Pts',(-56.366268079425,-16.9623071985392,-3.88949595769794));
#40504=CARTESIAN_POINT('Ctrl Pts',(-56.3395353657988,-16.8090480003591,
-4.25923828551908));
#40505=CARTESIAN_POINT('Ctrl Pts',(-56.3263779287031,-16.6934822832211,
-4.42798167302477));
#40506=CARTESIAN_POINT('Ctrl Pts',(-56.3048219679644,-16.4270526075957,
-4.69412389350912));
#40507=CARTESIAN_POINT('Ctrl Pts',(-56.2949857165266,-16.2585410496607,
-4.80941523738749));
#40508=CARTESIAN_POINT('Ctrl Pts',(-56.2817103328366,-15.889189778178,-4.96235566707568));
#40509=CARTESIAN_POINT('Ctrl Pts',(-56.2783262011229,-15.6883461217826,
-4.99999999999999));
#40510=CARTESIAN_POINT('Ctrl Pts',(-56.2783262011229,-15.5,-4.99999999999999));
#40511=CARTESIAN_POINT('Origin',(-74.,-14.,-4.99999999999999));
#40512=CARTESIAN_POINT('',(-56.2783262011229,-16.45,-4.99999999999999));
#40513=CARTESIAN_POINT('Origin',(0.,-18.3786796564404,0.));
#40514=CARTESIAN_POINT('',(-6.91925441518255E-15,-18.3786796564404,-56.5));
#40515=CARTESIAN_POINT('Origin',(0.,-18.3786796564404,0.));
#40516=CARTESIAN_POINT('Origin',(-6.73555739531044E-15,-18.3786796564404,
-55.));
#40517=CARTESIAN_POINT('Origin',(0.,-16.45,0.));
#40518=CARTESIAN_POINT('',(-5.00000000000001,-15.5,-56.2783262011229));
#40519=CARTESIAN_POINT('',(-5.00000000000001,-16.45,-56.2783262011229));
#40520=CARTESIAN_POINT('Ctrl Pts',(-5.00000000000001,-15.5,-56.2783262011229));
#40521=CARTESIAN_POINT('Ctrl Pts',(-5.00000000000001,-15.6883461217826,
-56.2783262011229));
#40522=CARTESIAN_POINT('Ctrl Pts',(-4.96235566707569,-15.889189778178,-56.2817103328366));
#40523=CARTESIAN_POINT('Ctrl Pts',(-4.80941523738751,-16.2585410496607,
-56.2949857165266));
#40524=CARTESIAN_POINT('Ctrl Pts',(-4.69412389350914,-16.4270526075957,
-56.3048219679644));
#40525=CARTESIAN_POINT('Ctrl Pts',(-4.42798167302479,-16.6934822832211,
-56.3263779287031));
#40526=CARTESIAN_POINT('Ctrl Pts',(-4.2592382855191,-16.8090480003591,-56.3395353657988));
#40527=CARTESIAN_POINT('Ctrl Pts',(-3.88949595769795,-16.9623071985392,
-56.366268079425));
#40528=CARTESIAN_POINT('Ctrl Pts',(-3.68849285843234,-17.,-56.379789702144));
#40529=CARTESIAN_POINT('Ctrl Pts',(-3.50000000000001,-17.,-56.3914887194867));
#40530=CARTESIAN_POINT('',(-6.91925441518255E-15,-16.45,-56.5));
#40531=CARTESIAN_POINT('',(-56.2783262011229,-16.45,5.00000000000001));
#40532=CARTESIAN_POINT('Origin',(-3.50000000000001,-15.5,-56.));
#40533=CARTESIAN_POINT('',(-5.00000000000001,-15.5,-56.));
#40534=CARTESIAN_POINT('Origin',(-5.00000000000001,-14.,-50.));
#40535=CARTESIAN_POINT('Origin',(-2.22044604925031E-15,-6.5,-1.11022302462516E-15));
#40536=CARTESIAN_POINT('',(-26.4408249076837,-5.,48.7968521341409));
#40537=CARTESIAN_POINT('',(26.4408249076837,-5.,48.7968521341409));
#40538=CARTESIAN_POINT('Origin',(-2.22044604925031E-15,-5.,-1.11022302462516E-15));
#40539=CARTESIAN_POINT('',(28.5,-6.5,49.363448015713));
#40540=CARTESIAN_POINT('Ctrl Pts',(26.4408249076837,-5.,48.7968521341409));
#40541=CARTESIAN_POINT('Ctrl Pts',(26.4433428933823,-5.,48.7975634354717));
#40542=CARTESIAN_POINT('Ctrl Pts',(26.4458608993077,-5.00000333058454,48.7982746736245));
#40543=CARTESIAN_POINT('Ctrl Pts',(26.6669469009444,-5.00058824010722,48.860716770933));
#40544=CARTESIAN_POINT('Ctrl Pts',(26.8870499673497,-5.02626861297965,48.9223486234079));
#40545=CARTESIAN_POINT('Ctrl Pts',(27.3015455654892,-5.12770348678069,49.037476260629));
#40546=CARTESIAN_POINT('Ctrl Pts',(27.4994252131301,-5.20145984176535,49.0919888636193));
#40547=CARTESIAN_POINT('Ctrl Pts',(27.8654608685803,-5.40254624808677,49.1921485479794));
#40548=CARTESIAN_POINT('Ctrl Pts',(28.0359950887546,-5.53136222218403,49.2384417005703));
#40549=CARTESIAN_POINT('Ctrl Pts',(28.2793834312809,-5.80849396878292,49.3042039204227));
#40550=CARTESIAN_POINT('Ctrl Pts',(28.3653378990205,-5.94334681379896,49.3273143295766));
#40551=CARTESIAN_POINT('Ctrl Pts',(28.4731331307579,-6.22254302463316,49.3562553083628));
#40552=CARTESIAN_POINT('Ctrl Pts',(28.5,-6.35969279486339,49.363448015713));
#40553=CARTESIAN_POINT('Ctrl Pts',(28.5,-6.5,49.363448015713));
#40554=CARTESIAN_POINT('',(-28.5,-6.5,49.363448015713));
#40555=CARTESIAN_POINT('Origin',(-2.22044604925031E-15,-6.5,-1.11022302462516E-15));
#40556=CARTESIAN_POINT('Ctrl Pts',(-28.5,-6.5,49.363448015713));
#40557=CARTESIAN_POINT('Ctrl Pts',(-28.5,-6.35969279486338,49.363448015713));
#40558=CARTESIAN_POINT('Ctrl Pts',(-28.4731331307579,-6.22254302463313,
49.3562553083628));
#40559=CARTESIAN_POINT('Ctrl Pts',(-28.3653378990205,-5.94334681379896,
49.3273143295766));
#40560=CARTESIAN_POINT('Ctrl Pts',(-28.2793834312809,-5.80849396878292,
49.3042039204227));
#40561=CARTESIAN_POINT('Ctrl Pts',(-28.0359950887546,-5.53136222218405,
49.2384417005703));
#40562=CARTESIAN_POINT('Ctrl Pts',(-27.8654608685804,-5.40254624808679,
49.1921485479794));
#40563=CARTESIAN_POINT('Ctrl Pts',(-27.4994252131301,-5.20145984176534,
49.0919888636193));
#40564=CARTESIAN_POINT('Ctrl Pts',(-27.3015455654892,-5.12770348678068,
49.037476260629));
#40565=CARTESIAN_POINT('Ctrl Pts',(-26.8870499673495,-5.0262686129796,48.9223486234078));
#40566=CARTESIAN_POINT('Ctrl Pts',(-26.666946900943,-5.00058824010721,48.8607167709328));
#40567=CARTESIAN_POINT('Ctrl Pts',(-26.4458608993078,-5.00000333058454,
48.7982746736245));
#40568=CARTESIAN_POINT('Ctrl Pts',(-26.4433428933823,-5.,48.7975634354716));
#40569=CARTESIAN_POINT('Ctrl Pts',(-26.4408249076837,-5.,48.7968521341409));
#40570=CARTESIAN_POINT('Origin',(31.4497077307402,-6.5,57.4724916728338));
#40571=CARTESIAN_POINT('',(33.7929481589963,-5.,61.5311031489229));
#40572=CARTESIAN_POINT('',(31.4497077307402,-5.,57.4724916728338));
#40573=CARTESIAN_POINT('',(35.1,-6.5,60.7949833456676));
#40574=CARTESIAN_POINT('Ctrl Pts',(35.1,-6.5,60.7949833456676));
#40575=CARTESIAN_POINT('Ctrl Pts',(35.1,-6.31165607666986,60.7949833456676));
#40576=CARTESIAN_POINT('Ctrl Pts',(35.0674179958086,-6.11075826580663,60.8138311041577));
#40577=CARTESIAN_POINT('Ctrl Pts',(34.9347215325305,-5.74118910309827,60.8901559359346));
#40578=CARTESIAN_POINT('Ctrl Pts',(34.8345853962734,-5.57251778949233,60.9475955008384));
#40579=CARTESIAN_POINT('Ctrl Pts',(34.603070183953,-5.30614953382508,61.0793359017089));
#40580=CARTESIAN_POINT('Ctrl Pts',(34.4562535838124,-5.19070605094542,61.1624128165762));
#40581=CARTESIAN_POINT('Ctrl Pts',(34.1337535001687,-5.03763156427752,61.3429786085339));
#40582=CARTESIAN_POINT('Ctrl Pts',(33.9580490505859,-5.,61.4404295613393));
#40583=CARTESIAN_POINT('Ctrl Pts',(33.7929481589963,-5.,61.5311031489229));
#40584=CARTESIAN_POINT('',(32.7487458364169,-6.5,56.7224916728338));
#40585=CARTESIAN_POINT('Origin',(-28.1497077307402,-6.5,51.7567240078565));
#40586=CARTESIAN_POINT('',(-35.1,-6.5,60.7949833456676));
#40587=CARTESIAN_POINT('',(-29.4487458364169,-6.5,51.0067240078565));
#40588=CARTESIAN_POINT('',(-33.7929481589964,-5.,61.5311031489229));
#40589=CARTESIAN_POINT('Ctrl Pts',(-33.7929481589964,-5.,61.5311031489229));
#40590=CARTESIAN_POINT('Ctrl Pts',(-33.9580490505859,-5.,61.4404295613392));
#40591=CARTESIAN_POINT('Ctrl Pts',(-34.1337535001687,-5.03763156427752,
61.3429786085339));
#40592=CARTESIAN_POINT('Ctrl Pts',(-34.4562535838124,-5.19070605094542,
61.1624128165762));
#40593=CARTESIAN_POINT('Ctrl Pts',(-34.603070183953,-5.30614953382508,61.0793359017089));
#40594=CARTESIAN_POINT('Ctrl Pts',(-34.8345853962734,-5.57251778949232,
60.9475955008384));
#40595=CARTESIAN_POINT('Ctrl Pts',(-34.9347215325305,-5.74118910309827,
60.8901559359346));
#40596=CARTESIAN_POINT('Ctrl Pts',(-35.0674179958086,-6.11075826580663,
60.8138311041577));
#40597=CARTESIAN_POINT('Ctrl Pts',(-35.1,-6.31165607666986,60.7949833456676));
#40598=CARTESIAN_POINT('Ctrl Pts',(-35.1,-6.5,60.7949833456676));
#40599=CARTESIAN_POINT('',(-28.1497077307402,-5.,51.7567240078565));
#40600=CARTESIAN_POINT('Origin',(0.,-5.,70.2));
#40601=CARTESIAN_POINT('Origin',(0.,-5.,0.));
#40602=CARTESIAN_POINT('Origin',(0.,-4.52901994577491,0.));
#40603=CARTESIAN_POINT('',(-8.61200836217972E-15,-4.52901994577491,70.2));
#40604=CARTESIAN_POINT('',(-8.59702053001442E-15,-4.52901994577491,-70.2));
#40605=CARTESIAN_POINT('Origin',(0.,-4.52901994577491,0.));
#40606=CARTESIAN_POINT('Origin',(0.,-4.52901994577491,0.));
#40607=CARTESIAN_POINT('',(0.,-3.05,71.95));
#40608=CARTESIAN_POINT('Origin',(-8.79602563487587E-15,-4.52901994577491,
71.7));
#40609=CARTESIAN_POINT('Origin',(0.,-3.05,0.));
#40610=CARTESIAN_POINT('Origin',(0.,-2.45,0.));
#40611=CARTESIAN_POINT('',(-35.1,-9.,60.7949833456676));
#40612=CARTESIAN_POINT('',(-35.1,-5.,60.7949833456676));
#40613=CARTESIAN_POINT('',(-8.59702053001442E-15,-9.,-70.2));
#40614=CARTESIAN_POINT('Origin',(1.55431223447522E-14,-9.,2.22044604925031E-15));
#40615=CARTESIAN_POINT('',(-8.59702053001442E-15,-2.45,-70.2));
#40616=CARTESIAN_POINT('',(35.1,-9.,60.7949833456676));
#40617=CARTESIAN_POINT('Origin',(1.55431223447522E-14,-9.,2.22044604925031E-15));
#40618=CARTESIAN_POINT('',(35.1,-5.,60.7949833456676));
#40619=CARTESIAN_POINT('Origin',(0.,-1.5,0.));
#40620=CARTESIAN_POINT('Ctrl Pts',(29.9536323812222,-2.71050543121376E-19,
-70.4463086837813));
#40621=CARTESIAN_POINT('Ctrl Pts',(29.4931113267111,3.61002085224869E-16,
-70.5699748242382));
#40622=CARTESIAN_POINT('Ctrl Pts',(29.0477953810644,-8.57026255143317E-17,
-70.754095087701));
#40623=CARTESIAN_POINT('Ctrl Pts',(28.6326460019314,-6.68817215151996E-17,
-70.9934791577936));
#40624=CARTESIAN_POINT('Ctrl Pts',(-28.6326460019314,1.4975542507456E-17,
-70.9934791577936));
#40625=CARTESIAN_POINT('Ctrl Pts',(-29.0457287289759,2.12326426962524E-18,
-70.7552867637899));
#40626=CARTESIAN_POINT('Ctrl Pts',(-29.4908073407614,-9.21355752057452E-17,
-70.570593525701));
#40627=CARTESIAN_POINT('Ctrl Pts',(-29.9536323812221,-8.76170880639848E-17,
-70.4463086837813));
#40628=CARTESIAN_POINT('Ctrl Pts',(-70.4463086837813,-3.38135552543917E-17,
-29.9536323812221));
#40629=CARTESIAN_POINT('Ctrl Pts',(-70.5699748242384,-4.02332320349957E-17,
-29.4931113267108));
#40630=CARTESIAN_POINT('Ctrl Pts',(-70.7540950877011,6.7489870141098E-18,
-29.0477953810642));
#40631=CARTESIAN_POINT('Ctrl Pts',(-70.9934791577937,1.68728963093057E-17,
-28.6326460019314));
#40632=CARTESIAN_POINT('Ctrl Pts',(-70.9934791577936,-2.71050543121376E-19,
28.6326460019316));
#40633=CARTESIAN_POINT('Ctrl Pts',(-70.75528676379,-4.16998824018934E-16,
29.0457287289757));
#40634=CARTESIAN_POINT('Ctrl Pts',(-70.5705935257011,-4.11774089579395E-16,
29.4908073407612));
#40635=CARTESIAN_POINT('Ctrl Pts',(-70.4463086837814,7.45388993583784E-19,
29.953632381222));
#40636=CARTESIAN_POINT('Ctrl Pts',(-29.9536323812221,-6.22060996463558E-17,
70.4463086837813));
#40637=CARTESIAN_POINT('Ctrl Pts',(-29.493111326711,3.15609360022052E-16,
70.5699748242383));
#40638=CARTESIAN_POINT('Ctrl Pts',(-29.0477953810643,-5.68950025513662E-17,
70.754095087701));
#40639=CARTESIAN_POINT('Ctrl Pts',(-28.6326460019314,-6.24771501894772E-17,
70.9934791577936));
#40640=CARTESIAN_POINT('',(-9.19097422760089E-15,-1.5,75.05));
#40641=CARTESIAN_POINT('Origin',(-9.37467124747299E-15,-1.5,76.55));
#40642=CARTESIAN_POINT('',(9.19097422760089E-15,-1.5,-75.05));
#40643=CARTESIAN_POINT('Origin',(0.,-1.5,0.));
#40644=CARTESIAN_POINT('Origin',(0.,-1.5,0.));
#40645=CARTESIAN_POINT('Ctrl Pts',(28.6326460019316,1.74827600313288E-17,
70.9934791577936));
#40646=CARTESIAN_POINT('Ctrl Pts',(29.0457287289756,-7.84991024395544E-16,
70.75528676379));
#40647=CARTESIAN_POINT('Ctrl Pts',(29.4908073407612,-3.46969577256769E-16,
70.5705935257011));
#40648=CARTESIAN_POINT('Ctrl Pts',(29.953632381222,6.44422666271072E-17,
70.4463086837814));
#40649=CARTESIAN_POINT('Ctrl Pts',(70.4463086837813,-1.61817174243462E-16,
29.9536323812221));
#40650=CARTESIAN_POINT('Ctrl Pts',(70.5699748242384,2.02397638118641E-16,
29.4931113267108));
#40651=CARTESIAN_POINT('Ctrl Pts',(70.7540950877011,3.82018796963149E-16,
29.0477953810642));
#40652=CARTESIAN_POINT('Ctrl Pts',(70.9934791577936,1.31459513413867E-17,
28.6326460019314));
#40653=CARTESIAN_POINT('Ctrl Pts',(70.9934791577936,1.03676832743926E-17,
-28.6326460019314));
#40654=CARTESIAN_POINT('Ctrl Pts',(70.7552867637899,-2.39154738916311E-18,
-29.0457287289758));
#40655=CARTESIAN_POINT('Ctrl Pts',(70.5705935257011,-5.99316384971288E-17,
-29.4908073407614));
#40656=CARTESIAN_POINT('Ctrl Pts',(70.4463086837813,-4.58075417875126E-17,
-29.9536323812221));
#40657=CARTESIAN_POINT('Origin',(-75.7581216659255,-14.1,-31.3800414539373));
#40658=CARTESIAN_POINT('',(-81.2581216659255,-14.1,-31.3800414539373));
#40659=CARTESIAN_POINT('Origin',(-31.3800414539373,-14.1,-75.7581216659255));
#40660=CARTESIAN_POINT('',(-36.8800414539373,-14.1,-75.7581216659255));
#40661=CARTESIAN_POINT('Origin',(31.3800414539374,-14.1,-75.7581216659255));
#40662=CARTESIAN_POINT('',(25.8800414539374,-14.1,-75.7581216659255));
#40663=CARTESIAN_POINT('Origin',(75.7581216659255,-14.1,-31.3800414539373));
#40664=CARTESIAN_POINT('',(70.2581216659255,-14.1,-31.3800414539373));
#40665=CARTESIAN_POINT('Origin',(0.,-1.475,0.));
#40666=CARTESIAN_POINT('',(-9.19097422760089E-15,-3.05,-75.05));
#40667=CARTESIAN_POINT('Origin',(0.,-3.05,0.));
#40668=CARTESIAN_POINT('',(-9.19097422760089E-15,-1.475,-75.05));
#40669=CARTESIAN_POINT('Origin',(-0.494909523403555,-18.5,-4.));
#40670=CARTESIAN_POINT('',(0.623124465346341,-19.5,4.99999976158142));
#40671=CARTESIAN_POINT('Origin',(-0.494909523403555,-18.5,4.99999976158142));
#40672=CARTESIAN_POINT('',(0.623124465346341,-19.5,-4.));
#40673=CARTESIAN_POINT('Origin',(-0.494909523403555,-18.5,-4.));
#40674=CARTESIAN_POINT('',(0.623124465346341,-19.5,-4.));
#40675=CARTESIAN_POINT('Origin',(-17.3346091195702,-18.5,-4.));
#40676=CARTESIAN_POINT('',(-16.2165751308203,-19.5,4.99999976158142));
#40677=CARTESIAN_POINT('Origin',(-17.3346091195702,-18.5,4.99999976158142));
#40678=CARTESIAN_POINT('',(-16.2165751308203,-19.5,-4.));
#40679=CARTESIAN_POINT('Origin',(-17.3346091195702,-18.5,-4.));
#40680=CARTESIAN_POINT('',(-16.2165751308203,-19.5,-4.));
#40681=CARTESIAN_POINT('Origin',(-25.6470237061142,-18.5,-4.));
#40682=CARTESIAN_POINT('',(-24.5289897173643,-19.5,4.99999976158142));
#40683=CARTESIAN_POINT('Origin',(-25.6470237061142,-18.5,4.99999976158142));
#40684=CARTESIAN_POINT('',(-24.5289897173643,-19.5,-4.));
#40685=CARTESIAN_POINT('Origin',(-25.6470237061142,-18.5,-4.));
#40686=CARTESIAN_POINT('',(-24.5289897173643,-19.5,-4.));
#40687=CARTESIAN_POINT('Origin',(7.65239799219948,-18.5,-3.5991740309707));
#40688=CARTESIAN_POINT('',(12.1524554491043,-19.5,4.99999976158142));
#40689=CARTESIAN_POINT('Origin',(10.9548091465744,-18.5,4.99999976158142));
#40690=CARTESIAN_POINT('',(8.55491101741791,-19.6302085441738,-4.));
#40691=CARTESIAN_POINT('Origin',(7.89500652006261,-18.5,-2.96744382018624));
#40692=CARTESIAN_POINT('',(8.69611181435176,-19.5,-4.));
#40693=CARTESIAN_POINT('Origin',(7.49846551182189,-18.5,-4.));
#40694=CARTESIAN_POINT('',(8.69611181435176,-19.5,-4.));
#40695=CARTESIAN_POINT('Origin',(14.4702638890185,-18.5,5.42348905947456));
#40696=CARTESIAN_POINT('',(17.1190309524536,-19.5,-4.));
#40697=CARTESIAN_POINT('Origin',(18.3270808427138,-18.5,-4.));
#40698=CARTESIAN_POINT('',(13.4355384111405,-19.5,4.99999976158142));
#40699=CARTESIAN_POINT('Origin',(14.6435883014006,-18.5,4.99999976158142));
#40700=CARTESIAN_POINT('',(13.4355384111405,-19.5,4.99999976158142));
#40701=CARTESIAN_POINT('Origin',(14.7124826908112,-20.,-1.27421581745148));
#40702=CARTESIAN_POINT('',(14.7124826908112,-19.5,-1.27421581745148));
#40703=CARTESIAN_POINT('',(14.7124826908112,-20.,-1.27421581745148));
#40704=CARTESIAN_POINT('',(10.9491813182831,-19.5,-1.27421581745148));
#40705=CARTESIAN_POINT('',(14.7124826908112,-19.5,-1.27421581745148));
#40706=CARTESIAN_POINT('',(10.9491813182831,-20.,-1.27421581745148));
#40707=CARTESIAN_POINT('Origin',(15.762277841568,-20.,-4.));
#40708=CARTESIAN_POINT('',(15.762277841568,-19.5,-4.));
#40709=CARTESIAN_POINT('',(15.762277841568,-20.,-4.));
#40710=CARTESIAN_POINT('',(15.762277841568,-19.5,-4.));
#40711=CARTESIAN_POINT('Origin',(17.1190309524536,-20.,-4.));
#40712=CARTESIAN_POINT('',(17.1190309524536,-19.5,-4.));
#40713=CARTESIAN_POINT('Origin',(12.1524554491043,-20.,4.99999976158142));
#40714=CARTESIAN_POINT('',(12.1524554491043,-19.5,4.99999976158142));
#40715=CARTESIAN_POINT('Origin',(9.96077753603459,-20.,-4.));
#40716=CARTESIAN_POINT('',(9.96077753603459,-19.5,-4.));
#40717=CARTESIAN_POINT('',(9.96077753603459,-20.,-4.));
#40718=CARTESIAN_POINT('',(9.96077753603459,-19.5,-4.));
#40719=CARTESIAN_POINT('',(8.55491101741791,-19.5,-4.));
#40720=CARTESIAN_POINT('',(8.55491101741791,-20.,-4.));
#40721=CARTESIAN_POINT('',(7.05695748329163,-19.5,-4.));
#40722=CARTESIAN_POINT('',(8.55491101741791,-19.5,-4.));
#40723=CARTESIAN_POINT('',(7.05695748329163,-20.,-4.));
#40724=CARTESIAN_POINT('Origin',(10.9491813182831,-20.,-1.27421581745148));
#40725=CARTESIAN_POINT('',(10.9491813182831,-19.5,-1.27421581745148));
#40726=CARTESIAN_POINT('Origin',(12.9075713834027,-19.5,0.49999988079071));
#40727=CARTESIAN_POINT('Origin',(-23.3379939198494,-20.,-2.93792629241943));
#40728=CARTESIAN_POINT('',(-23.3379939198494,-19.5,-2.93792629241943));
#40729=CARTESIAN_POINT('',(-23.3379939198494,-20.,-2.93792629241943));
#40730=CARTESIAN_POINT('',(-17.8127557039261,-19.5,-2.93792629241943));
#40731=CARTESIAN_POINT('',(-23.3379939198494,-19.5,-2.93792629241943));
#40732=CARTESIAN_POINT('',(-17.8127557039261,-20.,-2.93792629241943));
#40733=CARTESIAN_POINT('Origin',(-23.3379939198494,-20.,0.125511646270752));
#40734=CARTESIAN_POINT('',(-23.3379939198494,-19.5,0.125511646270752));
#40735=CARTESIAN_POINT('',(-23.3379939198494,-20.,0.125511646270752));
#40736=CARTESIAN_POINT('',(-23.3379939198494,-19.5,0.125511646270752));
#40737=CARTESIAN_POINT('Origin',(-18.3591401576996,-20.,0.125511646270752));
#40738=CARTESIAN_POINT('',(-18.3591401576996,-19.5,0.125511646270752));
#40739=CARTESIAN_POINT('',(-18.3591401576996,-20.,0.125511646270752));
#40740=CARTESIAN_POINT('',(-18.3591401576996,-19.5,0.125511646270752));
#40741=CARTESIAN_POINT('Origin',(-18.3591401576996,-20.,1.18144607543945));
#40742=CARTESIAN_POINT('',(-18.3591401576996,-19.5,1.18144607543945));
#40743=CARTESIAN_POINT('',(-18.3591401576996,-20.,1.18144607543945));
#40744=CARTESIAN_POINT('',(-18.3591401576996,-19.5,1.18144607543945));
#40745=CARTESIAN_POINT('Origin',(-23.3379939198494,-20.,1.18144607543945));
#40746=CARTESIAN_POINT('',(-23.3379939198494,-19.5,1.18144607543945));
#40747=CARTESIAN_POINT('',(-23.3379939198494,-20.,1.18144607543945));
#40748=CARTESIAN_POINT('',(-23.3379939198494,-19.5,1.18144607543945));
#40749=CARTESIAN_POINT('Origin',(-23.3379939198494,-20.,3.93792605400085));
#40750=CARTESIAN_POINT('',(-23.3379939198494,-19.5,3.93792605400085));
#40751=CARTESIAN_POINT('',(-23.3379939198494,-20.,3.93792605400085));
#40752=CARTESIAN_POINT('',(-23.3379939198494,-19.5,3.93792605400085));
#40753=CARTESIAN_POINT('Origin',(-18.0214869976044,-20.,3.93792605400085));
#40754=CARTESIAN_POINT('',(-18.0214869976044,-19.5,3.93792605400085));
#40755=CARTESIAN_POINT('',(-18.0214869976044,-20.,3.93792605400085));
#40756=CARTESIAN_POINT('',(-18.0214869976044,-19.5,3.93792605400085));
#40757=CARTESIAN_POINT('Origin',(-18.0214869976044,-20.,4.99999976158142));
#40758=CARTESIAN_POINT('',(-18.0214869976044,-19.5,4.99999976158142));
#40759=CARTESIAN_POINT('',(-18.0214869976044,-20.,4.99999976158142));
#40760=CARTESIAN_POINT('',(-18.0214869976044,-19.5,4.99999976158142));
#40761=CARTESIAN_POINT('Origin',(-24.5289897173643,-20.,4.99999976158142));
#40762=CARTESIAN_POINT('',(-24.5289897173643,-19.5,4.99999976158142));
#40763=CARTESIAN_POINT('Origin',(-17.8127557039261,-20.,-4.));
#40764=CARTESIAN_POINT('',(-17.8127557039261,-19.5,-4.));
#40765=CARTESIAN_POINT('',(-17.8127557039261,-20.,-4.));
#40766=CARTESIAN_POINT('',(-17.8127557039261,-19.5,-4.));
#40767=CARTESIAN_POINT('Origin',(-17.8127557039261,-20.,-2.93792629241943));
#40768=CARTESIAN_POINT('',(-17.8127557039261,-19.5,-2.93792629241943));
#40769=CARTESIAN_POINT('Origin',(-21.1708727106452,-19.5,0.49999988079071));
#40770=CARTESIAN_POINT('Ctrl Pts',(-10.3475439548492,-20.,-3.40450191497803));
#40771=CARTESIAN_POINT('Ctrl Pts',(-10.3475439548492,-19.5,-3.40450191497803));
#40772=CARTESIAN_POINT('Ctrl Pts',(-10.7404494285583,-20.,-3.69918131828308));
#40773=CARTESIAN_POINT('Ctrl Pts',(-10.7404494285583,-19.5,-3.69918131828308));
#40774=CARTESIAN_POINT('Ctrl Pts',(-11.3328778743744,-20.,-3.84959125518799));
#40775=CARTESIAN_POINT('Ctrl Pts',(-11.3328778743744,-19.5,-3.84959125518799));
#40776=CARTESIAN_POINT('',(-10.3475439548492,-19.5,-3.40450191497803));
#40777=CARTESIAN_POINT('',(-10.3475439548492,-20.,-3.40450191497803));
#40778=CARTESIAN_POINT('',(-11.3328778743744,-19.5,-3.84959125518799));
#40779=CARTESIAN_POINT('Ctrl Pts',(-10.3475439548492,-19.5,-3.40450191497803));
#40780=CARTESIAN_POINT('Ctrl Pts',(-10.7404494285583,-19.5,-3.69918131828308));
#40781=CARTESIAN_POINT('Ctrl Pts',(-11.3328778743744,-19.5,-3.84959125518799));
#40782=CARTESIAN_POINT('',(-11.3328778743744,-20.,-3.84959125518799));
#40783=CARTESIAN_POINT('Ctrl Pts',(-9.68758463859558,-20.,-2.56650769710541));
#40784=CARTESIAN_POINT('Ctrl Pts',(-9.68758463859558,-19.5,-2.56650769710541));
#40785=CARTESIAN_POINT('Ctrl Pts',(-9.95463788509369,-20.,-3.10982251167297));
#40786=CARTESIAN_POINT('Ctrl Pts',(-9.95463788509369,-19.5,-3.10982251167297));
#40787=CARTESIAN_POINT('Ctrl Pts',(-10.3475439548492,-20.,-3.40450191497803));
#40788=CARTESIAN_POINT('Ctrl Pts',(-10.3475439548492,-19.5,-3.40450191497803));
#40789=CARTESIAN_POINT('',(-9.68758463859558,-19.5,-2.56650769710541));
#40790=CARTESIAN_POINT('',(-9.68758463859558,-20.,-2.56650769710541));
#40791=CARTESIAN_POINT('Ctrl Pts',(-9.68758463859558,-19.5,-2.56650769710541));
#40792=CARTESIAN_POINT('Ctrl Pts',(-9.95463788509369,-19.5,-3.10982251167297));
#40793=CARTESIAN_POINT('Ctrl Pts',(-10.3475439548492,-19.5,-3.40450191497803));
#40794=CARTESIAN_POINT('Ctrl Pts',(-9.42053139209747,-20.,-1.39085972309113));
#40795=CARTESIAN_POINT('Ctrl Pts',(-9.42053139209747,-19.5,-1.39085972309113));
#40796=CARTESIAN_POINT('Ctrl Pts',(-9.42053139209747,-20.,-2.02319228649139));
#40797=CARTESIAN_POINT('Ctrl Pts',(-9.42053139209747,-19.5,-2.02319228649139));
#40798=CARTESIAN_POINT('Ctrl Pts',(-9.68758463859558,-20.,-2.56650769710541));
#40799=CARTESIAN_POINT('Ctrl Pts',(-9.68758463859558,-19.5,-2.56650769710541));
#40800=CARTESIAN_POINT('',(-9.42053139209747,-19.5,-1.39085972309113));
#40801=CARTESIAN_POINT('',(-9.42053139209747,-20.,-1.39085972309113));
#40802=CARTESIAN_POINT('Ctrl Pts',(-9.42053139209747,-19.5,-1.39085972309113));
#40803=CARTESIAN_POINT('Ctrl Pts',(-9.42053139209747,-19.5,-2.02319228649139));
#40804=CARTESIAN_POINT('Ctrl Pts',(-9.68758463859558,-19.5,-2.56650769710541));
#40805=CARTESIAN_POINT('Ctrl Pts',(-9.85948085784912,-20.,-0.0279673337936404));
#40806=CARTESIAN_POINT('Ctrl Pts',(-9.85948085784912,-19.5,-0.0279673337936404));
#40807=CARTESIAN_POINT('Ctrl Pts',(-9.42053139209747,-20.,-0.605048179626465));
#40808=CARTESIAN_POINT('Ctrl Pts',(-9.42053139209747,-19.5,-0.605048179626465));
#40809=CARTESIAN_POINT('Ctrl Pts',(-9.42053139209747,-20.,-1.39085972309113));
#40810=CARTESIAN_POINT('Ctrl Pts',(-9.42053139209747,-19.5,-1.39085972309113));
#40811=CARTESIAN_POINT('',(-9.85948085784912,-19.5,-0.0279673337936404));
#40812=CARTESIAN_POINT('',(-9.85948085784912,-20.,-0.0279673337936404));
#40813=CARTESIAN_POINT('Ctrl Pts',(-9.85948085784912,-19.5,-0.0279673337936404));
#40814=CARTESIAN_POINT('Ctrl Pts',(-9.42053139209747,-19.5,-0.605048179626465));
#40815=CARTESIAN_POINT('Ctrl Pts',(-9.42053139209747,-19.5,-1.39085972309113));
#40816=CARTESIAN_POINT('Ctrl Pts',(-11.1149382591248,-20.,0.788540005683899));
#40817=CARTESIAN_POINT('Ctrl Pts',(-11.1149382591248,-19.5,0.788540005683899));
#40818=CARTESIAN_POINT('Ctrl Pts',(-10.2984303236008,-20.,0.549112915992737));
#40819=CARTESIAN_POINT('Ctrl Pts',(-10.2984303236008,-19.5,0.549112915992737));
#40820=CARTESIAN_POINT('Ctrl Pts',(-9.85948085784912,-20.,-0.0279673337936404));
#40821=CARTESIAN_POINT('Ctrl Pts',(-9.85948085784912,-19.5,-0.0279673337936404));
#40822=CARTESIAN_POINT('',(-11.1149382591248,-19.5,0.788540005683899));
#40823=CARTESIAN_POINT('',(-11.1149382591248,-20.,0.788540005683899));
#40824=CARTESIAN_POINT('Ctrl Pts',(-11.1149382591248,-19.5,0.788540005683899));
#40825=CARTESIAN_POINT('Ctrl Pts',(-10.2984303236008,-19.5,0.549112915992737));
#40826=CARTESIAN_POINT('Ctrl Pts',(-9.85948085784912,-19.5,-0.0279673337936404));
#40827=CARTESIAN_POINT('Ctrl Pts',(-10.1695084571838,-20.,1.6111866235733));
#40828=CARTESIAN_POINT('Ctrl Pts',(-10.1695084571838,-19.5,1.6111866235733));
#40829=CARTESIAN_POINT('Ctrl Pts',(-10.482605099678,-20.,1.1016366481781));
#40830=CARTESIAN_POINT('Ctrl Pts',(-10.482605099678,-19.5,1.1016366481781));
#40831=CARTESIAN_POINT('Ctrl Pts',(-11.1149382591248,-20.,0.788540005683899));
#40832=CARTESIAN_POINT('Ctrl Pts',(-11.1149382591248,-19.5,0.788540005683899));
#40833=CARTESIAN_POINT('',(-10.1695084571838,-19.5,1.6111866235733));
#40834=CARTESIAN_POINT('',(-10.1695084571838,-20.,1.6111866235733));
#40835=CARTESIAN_POINT('Ctrl Pts',(-10.1695084571838,-19.5,1.6111866235733));
#40836=CARTESIAN_POINT('Ctrl Pts',(-10.482605099678,-19.5,1.1016366481781));
#40837=CARTESIAN_POINT('Ctrl Pts',(-11.1149382591248,-19.5,0.788540005683899));
#40838=CARTESIAN_POINT('Ctrl Pts',(-9.85641181468963,-20.,2.69781684875488));
#40839=CARTESIAN_POINT('Ctrl Pts',(-9.85641181468963,-19.5,2.69781684875488));
#40840=CARTESIAN_POINT('Ctrl Pts',(-9.85641181468963,-20.,2.12073659896851));
#40841=CARTESIAN_POINT('Ctrl Pts',(-9.85641181468963,-19.5,2.12073659896851));
#40842=CARTESIAN_POINT('Ctrl Pts',(-10.1695084571838,-20.,1.6111866235733));
#40843=CARTESIAN_POINT('Ctrl Pts',(-10.1695084571838,-19.5,1.6111866235733));
#40844=CARTESIAN_POINT('',(-9.85641181468963,-19.5,2.69781684875488));
#40845=CARTESIAN_POINT('',(-9.85641181468963,-20.,2.69781684875488));
#40846=CARTESIAN_POINT('Ctrl Pts',(-9.85641181468963,-19.5,2.69781684875488));
#40847=CARTESIAN_POINT('Ctrl Pts',(-9.85641181468963,-19.5,2.12073659896851));
#40848=CARTESIAN_POINT('Ctrl Pts',(-10.1695084571838,-19.5,1.6111866235733));
#40849=CARTESIAN_POINT('Ctrl Pts',(-10.2094125747681,-20.,3.8857433795929));
#40850=CARTESIAN_POINT('Ctrl Pts',(-10.2094125747681,-19.5,3.8857433795929));
#40851=CARTESIAN_POINT('Ctrl Pts',(-9.85641181468963,-20.,3.31787145137787));
#40852=CARTESIAN_POINT('Ctrl Pts',(-9.85641181468963,-19.5,3.31787145137787));
#40853=CARTESIAN_POINT('Ctrl Pts',(-9.85641181468963,-20.,2.69781684875488));
#40854=CARTESIAN_POINT('Ctrl Pts',(-9.85641181468963,-19.5,2.69781684875488));
#40855=CARTESIAN_POINT('',(-10.2094125747681,-19.5,3.8857433795929));
#40856=CARTESIAN_POINT('',(-10.2094125747681,-20.,3.8857433795929));
#40857=CARTESIAN_POINT('Ctrl Pts',(-10.2094125747681,-19.5,3.8857433795929));
#40858=CARTESIAN_POINT('Ctrl Pts',(-9.85641181468963,-19.5,3.31787145137787));
#40859=CARTESIAN_POINT('Ctrl Pts',(-9.85641181468963,-19.5,2.69781684875488));
#40860=CARTESIAN_POINT('Ctrl Pts',(-11.1855381727219,-20.,4.72680723667145));
#40861=CARTESIAN_POINT('Ctrl Pts',(-11.1855381727219,-19.5,4.72680723667145));
#40862=CARTESIAN_POINT('Ctrl Pts',(-10.5624139308929,-20.,4.45361471176147));
#40863=CARTESIAN_POINT('Ctrl Pts',(-10.5624139308929,-19.5,4.45361471176147));
#40864=CARTESIAN_POINT('Ctrl Pts',(-10.2094125747681,-20.,3.8857433795929));
#40865=CARTESIAN_POINT('Ctrl Pts',(-10.2094125747681,-19.5,3.8857433795929));
#40866=CARTESIAN_POINT('',(-11.1855381727219,-19.5,4.72680723667145));
#40867=CARTESIAN_POINT('',(-11.1855381727219,-20.,4.72680723667145));
#40868=CARTESIAN_POINT('Ctrl Pts',(-11.1855381727219,-19.5,4.72680723667145));
#40869=CARTESIAN_POINT('Ctrl Pts',(-10.5624139308929,-19.5,4.45361471176147));
#40870=CARTESIAN_POINT('Ctrl Pts',(-10.2094125747681,-19.5,3.8857433795929));
#40871=CARTESIAN_POINT('Ctrl Pts',(-12.8400406241417,-20.,4.99999976158142));
#40872=CARTESIAN_POINT('Ctrl Pts',(-12.8400406241417,-19.5,4.99999976158142));
#40873=CARTESIAN_POINT('Ctrl Pts',(-11.8086624145508,-20.,4.99999976158142));
#40874=CARTESIAN_POINT('Ctrl Pts',(-11.8086624145508,-19.5,4.99999976158142));
#40875=CARTESIAN_POINT('Ctrl Pts',(-11.1855381727219,-20.,4.72680723667145));
#40876=CARTESIAN_POINT('Ctrl Pts',(-11.1855381727219,-19.5,4.72680723667145));
#40877=CARTESIAN_POINT('',(-12.8400406241417,-19.5,4.99999976158142));
#40878=CARTESIAN_POINT('',(-12.8400406241417,-20.,4.99999976158142));
#40879=CARTESIAN_POINT('Ctrl Pts',(-12.8400406241417,-19.5,4.99999976158142));
#40880=CARTESIAN_POINT('Ctrl Pts',(-11.8086624145508,-19.5,4.99999976158142));
#40881=CARTESIAN_POINT('Ctrl Pts',(-11.1855381727219,-19.5,4.72680723667145));
#40882=CARTESIAN_POINT('Origin',(-16.2165751308203,-20.,4.99999976158142));
#40883=CARTESIAN_POINT('',(-16.2165751308203,-19.5,4.99999976158142));
#40884=CARTESIAN_POINT('Origin',(-12.7847883105278,-20.,-4.));
#40885=CARTESIAN_POINT('',(-12.7847883105278,-19.5,-4.));
#40886=CARTESIAN_POINT('',(-12.7847883105278,-20.,-4.));
#40887=CARTESIAN_POINT('',(-12.7847883105278,-19.5,-4.));
#40888=CARTESIAN_POINT('Ctrl Pts',(-11.3328778743744,-20.,-3.84959125518799));
#40889=CARTESIAN_POINT('Ctrl Pts',(-11.3328778743744,-19.5,-3.84959125518799));
#40890=CARTESIAN_POINT('Ctrl Pts',(-11.9253063201904,-20.,-4.));
#40891=CARTESIAN_POINT('Ctrl Pts',(-11.9253063201904,-19.5,-4.));
#40892=CARTESIAN_POINT('Ctrl Pts',(-12.7847883105278,-20.,-4.));
#40893=CARTESIAN_POINT('Ctrl Pts',(-12.7847883105278,-19.5,-4.));
#40894=CARTESIAN_POINT('Ctrl Pts',(-11.3328778743744,-19.5,-3.84959125518799));
#40895=CARTESIAN_POINT('Ctrl Pts',(-11.9253063201904,-19.5,-4.));
#40896=CARTESIAN_POINT('Ctrl Pts',(-12.7847883105278,-19.5,-4.));
#40897=CARTESIAN_POINT('Origin',(-12.8185532614589,-19.5,0.49999988079071));
#40898=CARTESIAN_POINT('Ctrl Pts',(-4.34959053993225,-20.,-4.15347838401794));
#40899=CARTESIAN_POINT('Ctrl Pts',(-4.34959053993225,-19.5,-4.15347838401794));
#40900=CARTESIAN_POINT('Ctrl Pts',(-5.57128190994263,-20.,-4.15347838401794));
#40901=CARTESIAN_POINT('Ctrl Pts',(-5.57128190994263,-19.5,-4.15347838401794));
#40902=CARTESIAN_POINT('Ctrl Pts',(-6.39699831604958,-20.,-3.79740738868713));
#40903=CARTESIAN_POINT('Ctrl Pts',(-6.39699831604958,-19.5,-3.79740738868713));
#40904=CARTESIAN_POINT('',(-4.34959053993225,-19.5,-4.15347838401794));
#40905=CARTESIAN_POINT('',(-4.34959053993225,-20.,-4.15347838401794));
#40906=CARTESIAN_POINT('',(-6.39699831604958,-19.5,-3.79740738868713));
#40907=CARTESIAN_POINT('Ctrl Pts',(-4.34959053993225,-19.5,-4.15347838401794));
#40908=CARTESIAN_POINT('Ctrl Pts',(-5.57128190994263,-19.5,-4.15347838401794));
#40909=CARTESIAN_POINT('Ctrl Pts',(-6.39699831604958,-19.5,-3.79740738868713));
#40910=CARTESIAN_POINT('',(-6.39699831604958,-20.,-3.79740738868713));
#40911=CARTESIAN_POINT('Ctrl Pts',(-2.61527955532074,-20.,-3.80047702789307));
#40912=CARTESIAN_POINT('Ctrl Pts',(-2.61527955532074,-19.5,-3.80047702789307));
#40913=CARTESIAN_POINT('Ctrl Pts',(-3.38574349880219,-20.,-4.15347838401794));
#40914=CARTESIAN_POINT('Ctrl Pts',(-3.38574349880219,-19.5,-4.15347838401794));
#40915=CARTESIAN_POINT('Ctrl Pts',(-4.34959053993225,-20.,-4.15347838401794));
#40916=CARTESIAN_POINT('Ctrl Pts',(-4.34959053993225,-19.5,-4.15347838401794));
#40917=CARTESIAN_POINT('',(-2.61527955532074,-19.5,-3.80047702789307));
#40918=CARTESIAN_POINT('',(-2.61527955532074,-20.,-3.80047702789307));
#40919=CARTESIAN_POINT('Ctrl Pts',(-2.61527955532074,-19.5,-3.80047702789307));
#40920=CARTESIAN_POINT('Ctrl Pts',(-3.38574349880219,-19.5,-4.15347838401794));
#40921=CARTESIAN_POINT('Ctrl Pts',(-4.34959053993225,-19.5,-4.15347838401794));
#40922=CARTESIAN_POINT('Ctrl Pts',(-1.43349230289459,-20.,-2.81207346916199));
#40923=CARTESIAN_POINT('Ctrl Pts',(-1.43349230289459,-19.5,-2.81207346916199));
#40924=CARTESIAN_POINT('Ctrl Pts',(-1.84481561183929,-20.,-3.44747567176819));
#40925=CARTESIAN_POINT('Ctrl Pts',(-1.84481561183929,-19.5,-3.44747567176819));
#40926=CARTESIAN_POINT('Ctrl Pts',(-2.61527955532074,-20.,-3.80047702789307));
#40927=CARTESIAN_POINT('Ctrl Pts',(-2.61527955532074,-19.5,-3.80047702789307));
#40928=CARTESIAN_POINT('',(-1.43349230289459,-19.5,-2.81207346916199));
#40929=CARTESIAN_POINT('',(-1.43349230289459,-20.,-2.81207346916199));
#40930=CARTESIAN_POINT('Ctrl Pts',(-1.43349230289459,-19.5,-2.81207346916199));
#40931=CARTESIAN_POINT('Ctrl Pts',(-1.84481561183929,-19.5,-3.44747567176819));
#40932=CARTESIAN_POINT('Ctrl Pts',(-2.61527955532074,-19.5,-3.80047702789307));
#40933=CARTESIAN_POINT('Ctrl Pts',(-1.02216899394989,-20.,-1.4583899974823));
#40934=CARTESIAN_POINT('Ctrl Pts',(-1.02216899394989,-19.5,-1.4583899974823));
#40935=CARTESIAN_POINT('Ctrl Pts',(-1.02216899394989,-20.,-2.17667126655579));
#40936=CARTESIAN_POINT('Ctrl Pts',(-1.02216899394989,-19.5,-2.17667126655579));
#40937=CARTESIAN_POINT('Ctrl Pts',(-1.43349230289459,-20.,-2.81207346916199));
#40938=CARTESIAN_POINT('Ctrl Pts',(-1.43349230289459,-19.5,-2.81207346916199));
#40939=CARTESIAN_POINT('',(-1.02216899394989,-19.5,-1.4583899974823));
#40940=CARTESIAN_POINT('',(-1.02216899394989,-20.,-1.4583899974823));
#40941=CARTESIAN_POINT('Ctrl Pts',(-1.02216899394989,-19.5,-1.4583899974823));
#40942=CARTESIAN_POINT('Ctrl Pts',(-1.02216899394989,-19.5,-2.17667126655579));
#40943=CARTESIAN_POINT('Ctrl Pts',(-1.43349230289459,-19.5,-2.81207346916199));
#40944=CARTESIAN_POINT('Ctrl Pts',(-1.39665722846985,-20.,-0.1783766746521));
#40945=CARTESIAN_POINT('Ctrl Pts',(-1.39665722846985,-19.5,-0.1783766746521));
#40946=CARTESIAN_POINT('Ctrl Pts',(-1.02216899394989,-20.,-0.733970642089844));
#40947=CARTESIAN_POINT('Ctrl Pts',(-1.02216899394989,-19.5,-0.733970642089844));
#40948=CARTESIAN_POINT('Ctrl Pts',(-1.02216899394989,-20.,-1.4583899974823));
#40949=CARTESIAN_POINT('Ctrl Pts',(-1.02216899394989,-19.5,-1.4583899974823));
#40950=CARTESIAN_POINT('',(-1.39665722846985,-19.5,-0.1783766746521));
#40951=CARTESIAN_POINT('',(-1.39665722846985,-20.,-0.1783766746521));
#40952=CARTESIAN_POINT('Ctrl Pts',(-1.39665722846985,-19.5,-0.1783766746521));
#40953=CARTESIAN_POINT('Ctrl Pts',(-1.02216899394989,-19.5,-0.733970642089844));
#40954=CARTESIAN_POINT('Ctrl Pts',(-1.02216899394989,-19.5,-1.4583899974823));
#40955=CARTESIAN_POINT('Ctrl Pts',(-2.55695760250092,-20.,0.739426374435425));
#40956=CARTESIAN_POINT('Ctrl Pts',(-2.55695760250092,-19.5,0.739426374435425));
#40957=CARTESIAN_POINT('Ctrl Pts',(-1.77114546298981,-20.,0.377216696739197));
#40958=CARTESIAN_POINT('Ctrl Pts',(-1.77114546298981,-19.5,0.377216696739197));
#40959=CARTESIAN_POINT('Ctrl Pts',(-1.39665722846985,-20.,-0.1783766746521));
#40960=CARTESIAN_POINT('Ctrl Pts',(-1.39665722846985,-19.5,-0.1783766746521));
#40961=CARTESIAN_POINT('',(-2.55695760250092,-19.5,0.739426374435425));
#40962=CARTESIAN_POINT('',(-2.55695760250092,-20.,0.739426374435425));
#40963=CARTESIAN_POINT('Ctrl Pts',(-2.55695760250092,-19.5,0.739426374435425));
#40964=CARTESIAN_POINT('Ctrl Pts',(-1.77114546298981,-19.5,0.377216696739197));
#40965=CARTESIAN_POINT('Ctrl Pts',(-1.39665722846985,-19.5,-0.1783766746521));
#40966=CARTESIAN_POINT('Ctrl Pts',(-4.54911291599274,-20.,1.31343758106232));
#40967=CARTESIAN_POINT('Ctrl Pts',(-4.54911291599274,-19.5,1.31343758106232));
#40968=CARTESIAN_POINT('Ctrl Pts',(-3.09720277786255,-20.,0.984992742538452));
#40969=CARTESIAN_POINT('Ctrl Pts',(-3.09720277786255,-19.5,0.984992742538452));
#40970=CARTESIAN_POINT('Ctrl Pts',(-2.55695760250092,-20.,0.739426374435425));
#40971=CARTESIAN_POINT('Ctrl Pts',(-2.55695760250092,-19.5,0.739426374435425));
#40972=CARTESIAN_POINT('',(-4.54911291599274,-19.5,1.31343758106232));
#40973=CARTESIAN_POINT('',(-4.54911291599274,-20.,1.31343758106232));
#40974=CARTESIAN_POINT('Ctrl Pts',(-4.54911291599274,-19.5,1.31343758106232));
#40975=CARTESIAN_POINT('Ctrl Pts',(-3.09720277786255,-19.5,0.984992742538452));
#40976=CARTESIAN_POINT('Ctrl Pts',(-2.55695760250092,-19.5,0.739426374435425));
#40977=CARTESIAN_POINT('Ctrl Pts',(-6.34481549263,-20.,1.95497906208038));
#40978=CARTESIAN_POINT('Ctrl Pts',(-6.34481549263,-19.5,1.95497906208038));
#40979=CARTESIAN_POINT('Ctrl Pts',(-6.00102305412292,-20.,1.64188241958618));
#40980=CARTESIAN_POINT('Ctrl Pts',(-6.00102305412292,-19.5,1.64188241958618));
#40981=CARTESIAN_POINT('Ctrl Pts',(-4.54911291599274,-20.,1.31343758106232));
#40982=CARTESIAN_POINT('Ctrl Pts',(-4.54911291599274,-19.5,1.31343758106232));
#40983=CARTESIAN_POINT('',(-6.34481549263,-19.5,1.95497906208038));
#40984=CARTESIAN_POINT('',(-6.34481549263,-20.,1.95497906208038));
#40985=CARTESIAN_POINT('Ctrl Pts',(-6.34481549263,-19.5,1.95497906208038));
#40986=CARTESIAN_POINT('Ctrl Pts',(-6.00102305412292,-19.5,1.64188241958618));
#40987=CARTESIAN_POINT('Ctrl Pts',(-4.54911291599274,-19.5,1.31343758106232));
#40988=CARTESIAN_POINT('Ctrl Pts',(-6.69474720954895,-20.,2.75306916236877));
#40989=CARTESIAN_POINT('Ctrl Pts',(-6.69474720954895,-19.5,2.75306916236877));
#40990=CARTESIAN_POINT('Ctrl Pts',(-6.69474720954895,-20.,2.26807570457458));
#40991=CARTESIAN_POINT('Ctrl Pts',(-6.69474720954895,-19.5,2.26807570457458));
#40992=CARTESIAN_POINT('Ctrl Pts',(-6.34481549263,-20.,1.95497906208038));
#40993=CARTESIAN_POINT('Ctrl Pts',(-6.34481549263,-19.5,1.95497906208038));
#40994=CARTESIAN_POINT('',(-6.69474720954895,-19.5,2.75306916236877));
#40995=CARTESIAN_POINT('',(-6.69474720954895,-20.,2.75306916236877));
#40996=CARTESIAN_POINT('Ctrl Pts',(-6.69474720954895,-19.5,2.75306916236877));
#40997=CARTESIAN_POINT('Ctrl Pts',(-6.69474720954895,-19.5,2.26807570457458));
#40998=CARTESIAN_POINT('Ctrl Pts',(-6.34481549263,-19.5,1.95497906208038));
#40999=CARTESIAN_POINT('Ctrl Pts',(-6.20054543018341,-20.,3.70770728588104));
#41000=CARTESIAN_POINT('Ctrl Pts',(-6.20054543018341,-19.5,3.70770728588104));
#41001=CARTESIAN_POINT('Ctrl Pts',(-6.69474720954895,-20.,3.311732172966));
#41002=CARTESIAN_POINT('Ctrl Pts',(-6.69474720954895,-19.5,3.311732172966));
#41003=CARTESIAN_POINT('Ctrl Pts',(-6.69474720954895,-20.,2.75306916236877));
#41004=CARTESIAN_POINT('Ctrl Pts',(-6.69474720954895,-19.5,2.75306916236877));
#41005=CARTESIAN_POINT('',(-6.20054543018341,-19.5,3.70770728588104));
#41006=CARTESIAN_POINT('',(-6.20054543018341,-20.,3.70770728588104));
#41007=CARTESIAN_POINT('Ctrl Pts',(-6.20054543018341,-19.5,3.70770728588104));
#41008=CARTESIAN_POINT('Ctrl Pts',(-6.69474720954895,-19.5,3.311732172966));
#41009=CARTESIAN_POINT('Ctrl Pts',(-6.69474720954895,-19.5,2.75306916236877));
#41010=CARTESIAN_POINT('Ctrl Pts',(-4.62585210800171,-20.,4.10368299484253));
#41011=CARTESIAN_POINT('Ctrl Pts',(-4.62585210800171,-19.5,4.10368299484253));
#41012=CARTESIAN_POINT('Ctrl Pts',(-5.70634365081787,-20.,4.10368299484253));
#41013=CARTESIAN_POINT('Ctrl Pts',(-5.70634365081787,-19.5,4.10368299484253));
#41014=CARTESIAN_POINT('Ctrl Pts',(-6.20054543018341,-20.,3.70770728588104));
#41015=CARTESIAN_POINT('Ctrl Pts',(-6.20054543018341,-19.5,3.70770728588104));
#41016=CARTESIAN_POINT('',(-4.62585210800171,-19.5,4.10368299484253));
#41017=CARTESIAN_POINT('',(-4.62585210800171,-20.,4.10368299484253));
#41018=CARTESIAN_POINT('Ctrl Pts',(-4.62585210800171,-19.5,4.10368299484253));
#41019=CARTESIAN_POINT('Ctrl Pts',(-5.70634365081787,-19.5,4.10368299484253));
#41020=CARTESIAN_POINT('Ctrl Pts',(-6.20054543018341,-19.5,3.70770728588104));
#41021=CARTESIAN_POINT('Ctrl Pts',(-3.05729866027832,-20.,3.66780316829681));
#41022=CARTESIAN_POINT('Ctrl Pts',(-3.05729866027832,-19.5,3.66780316829681));
#41023=CARTESIAN_POINT('Ctrl Pts',(-3.5883355140686,-20.,4.10368299484253));
#41024=CARTESIAN_POINT('Ctrl Pts',(-3.5883355140686,-19.5,4.10368299484253));
#41025=CARTESIAN_POINT('Ctrl Pts',(-4.62585210800171,-20.,4.10368299484253));
#41026=CARTESIAN_POINT('Ctrl Pts',(-4.62585210800171,-19.5,4.10368299484253));
#41027=CARTESIAN_POINT('',(-3.05729866027832,-19.5,3.66780316829681));
#41028=CARTESIAN_POINT('',(-3.05729866027832,-20.,3.66780316829681));
#41029=CARTESIAN_POINT('Ctrl Pts',(-3.05729866027832,-19.5,3.66780316829681));
#41030=CARTESIAN_POINT('Ctrl Pts',(-3.5883355140686,-19.5,4.10368299484253));
#41031=CARTESIAN_POINT('Ctrl Pts',(-4.62585210800171,-19.5,4.10368299484253));
#41032=CARTESIAN_POINT('Ctrl Pts',(-2.4341744184494,-20.,2.37858092784882));
#41033=CARTESIAN_POINT('Ctrl Pts',(-2.4341744184494,-19.5,2.37858092784882));
#41034=CARTESIAN_POINT('Ctrl Pts',(-2.52626180648804,-20.,3.2319233417511));
#41035=CARTESIAN_POINT('Ctrl Pts',(-2.52626180648804,-19.5,3.2319233417511));
#41036=CARTESIAN_POINT('Ctrl Pts',(-3.05729866027832,-20.,3.66780316829681));
#41037=CARTESIAN_POINT('Ctrl Pts',(-3.05729866027832,-19.5,3.66780316829681));
#41038=CARTESIAN_POINT('',(-2.4341744184494,-19.5,2.37858092784882));
#41039=CARTESIAN_POINT('',(-2.4341744184494,-20.,2.37858092784882));
#41040=CARTESIAN_POINT('Ctrl Pts',(-2.4341744184494,-19.5,2.37858092784882));
#41041=CARTESIAN_POINT('Ctrl Pts',(-2.52626180648804,-19.5,3.2319233417511));
#41042=CARTESIAN_POINT('Ctrl Pts',(-3.05729866027832,-19.5,3.66780316829681));
#41043=CARTESIAN_POINT('Origin',(-1.29229187965393,-20.,2.46452903747559));
#41044=CARTESIAN_POINT('',(-1.29229187965393,-19.5,2.46452903747559));
#41045=CARTESIAN_POINT('',(-1.29229187965393,-20.,2.46452903747559));
#41046=CARTESIAN_POINT('',(-1.29229187965393,-19.5,2.46452903747559));
#41047=CARTESIAN_POINT('Ctrl Pts',(-1.73431098461151,-20.,3.88267314434052));
#41048=CARTESIAN_POINT('Ctrl Pts',(-1.73431098461151,-19.5,3.88267314434052));
#41049=CARTESIAN_POINT('Ctrl Pts',(-1.32298767566681,-20.,3.25647985935211));
#41050=CARTESIAN_POINT('Ctrl Pts',(-1.32298767566681,-19.5,3.25647985935211));
#41051=CARTESIAN_POINT('Ctrl Pts',(-1.29229187965393,-20.,2.46452903747559));
#41052=CARTESIAN_POINT('Ctrl Pts',(-1.29229187965393,-19.5,2.46452903747559));
#41053=CARTESIAN_POINT('',(-1.73431098461151,-19.5,3.88267314434052));
#41054=CARTESIAN_POINT('',(-1.73431098461151,-20.,3.88267314434052));
#41055=CARTESIAN_POINT('Ctrl Pts',(-1.73431098461151,-19.5,3.88267314434052));
#41056=CARTESIAN_POINT('Ctrl Pts',(-1.32298767566681,-19.5,3.25647985935211));
#41057=CARTESIAN_POINT('Ctrl Pts',(-1.29229187965393,-19.5,2.46452903747559));
#41058=CARTESIAN_POINT('Ctrl Pts',(-2.90995895862579,-20.,4.83117258548737));
#41059=CARTESIAN_POINT('Ctrl Pts',(-2.90995895862579,-19.5,4.83117258548737));
#41060=CARTESIAN_POINT('Ctrl Pts',(-2.14563429355621,-20.,4.50886702537537));
#41061=CARTESIAN_POINT('Ctrl Pts',(-2.14563429355621,-19.5,4.50886702537537));
#41062=CARTESIAN_POINT('Ctrl Pts',(-1.73431098461151,-20.,3.88267314434052));
#41063=CARTESIAN_POINT('Ctrl Pts',(-1.73431098461151,-19.5,3.88267314434052));
#41064=CARTESIAN_POINT('',(-2.90995895862579,-19.5,4.83117258548737));
#41065=CARTESIAN_POINT('',(-2.90995895862579,-20.,4.83117258548737));
#41066=CARTESIAN_POINT('Ctrl Pts',(-2.90995895862579,-19.5,4.83117258548737));
#41067=CARTESIAN_POINT('Ctrl Pts',(-2.14563429355621,-19.5,4.50886702537537));
#41068=CARTESIAN_POINT('Ctrl Pts',(-1.73431098461151,-19.5,3.88267314434052));
#41069=CARTESIAN_POINT('Ctrl Pts',(-4.67496573925018,-20.,5.15347814559937));
#41070=CARTESIAN_POINT('Ctrl Pts',(-4.67496573925018,-19.5,5.15347814559937));
#41071=CARTESIAN_POINT('Ctrl Pts',(-3.67428362369537,-20.,5.15347814559937));
#41072=CARTESIAN_POINT('Ctrl Pts',(-3.67428362369537,-19.5,5.15347814559937));
#41073=CARTESIAN_POINT('Ctrl Pts',(-2.90995895862579,-20.,4.83117258548737));
#41074=CARTESIAN_POINT('Ctrl Pts',(-2.90995895862579,-19.5,4.83117258548737));
#41075=CARTESIAN_POINT('',(-4.67496573925018,-19.5,5.15347814559937));
#41076=CARTESIAN_POINT('',(-4.67496573925018,-20.,5.15347814559937));
#41077=CARTESIAN_POINT('Ctrl Pts',(-4.67496573925018,-19.5,5.15347814559937));
#41078=CARTESIAN_POINT('Ctrl Pts',(-3.67428362369537,-19.5,5.15347814559937));
#41079=CARTESIAN_POINT('Ctrl Pts',(-2.90995895862579,-19.5,4.83117258548737));
#41080=CARTESIAN_POINT('Ctrl Pts',(-6.32639795541763,-20.,4.84652078151703));
#41081=CARTESIAN_POINT('Ctrl Pts',(-6.32639795541763,-19.5,4.84652078151703));
#41082=CARTESIAN_POINT('Ctrl Pts',(-5.58356046676636,-20.,5.15347814559937));
#41083=CARTESIAN_POINT('Ctrl Pts',(-5.58356046676636,-19.5,5.15347814559937));
#41084=CARTESIAN_POINT('Ctrl Pts',(-4.67496573925018,-20.,5.15347814559937));
#41085=CARTESIAN_POINT('Ctrl Pts',(-4.67496573925018,-19.5,5.15347814559937));
#41086=CARTESIAN_POINT('',(-6.32639795541763,-19.5,4.84652078151703));
#41087=CARTESIAN_POINT('',(-6.32639795541763,-20.,4.84652078151703));
#41088=CARTESIAN_POINT('Ctrl Pts',(-6.32639795541763,-19.5,4.84652078151703));
#41089=CARTESIAN_POINT('Ctrl Pts',(-5.58356046676636,-19.5,5.15347814559937));
#41090=CARTESIAN_POINT('Ctrl Pts',(-4.67496573925018,-19.5,5.15347814559937));
#41091=CARTESIAN_POINT('Ctrl Pts',(-7.4560022354126,-20.,3.9471343755722));
#41092=CARTESIAN_POINT('Ctrl Pts',(-7.4560022354126,-19.5,3.9471343755722));
#41093=CARTESIAN_POINT('Ctrl Pts',(-7.06923559308052,-20.,4.53956282138824));
#41094=CARTESIAN_POINT('Ctrl Pts',(-7.06923559308052,-19.5,4.53956282138824));
#41095=CARTESIAN_POINT('Ctrl Pts',(-6.32639795541763,-20.,4.84652078151703));
#41096=CARTESIAN_POINT('Ctrl Pts',(-6.32639795541763,-19.5,4.84652078151703));
#41097=CARTESIAN_POINT('',(-7.4560022354126,-19.5,3.9471343755722));
#41098=CARTESIAN_POINT('',(-7.4560022354126,-20.,3.9471343755722));
#41099=CARTESIAN_POINT('Ctrl Pts',(-7.4560022354126,-19.5,3.9471343755722));
#41100=CARTESIAN_POINT('Ctrl Pts',(-7.06923559308052,-19.5,4.53956282138824));
#41101=CARTESIAN_POINT('Ctrl Pts',(-6.32639795541763,-19.5,4.84652078151703));
#41102=CARTESIAN_POINT('Ctrl Pts',(-7.84276902675629,-20.,2.67326033115387));
#41103=CARTESIAN_POINT('Ctrl Pts',(-7.84276902675629,-19.5,2.67326033115387));
#41104=CARTESIAN_POINT('Ctrl Pts',(-7.84276902675629,-20.,3.35470592975616));
#41105=CARTESIAN_POINT('Ctrl Pts',(-7.84276902675629,-19.5,3.35470592975616));
#41106=CARTESIAN_POINT('Ctrl Pts',(-7.4560022354126,-20.,3.9471343755722));
#41107=CARTESIAN_POINT('Ctrl Pts',(-7.4560022354126,-19.5,3.9471343755722));
#41108=CARTESIAN_POINT('',(-7.84276902675629,-19.5,2.67326033115387));
#41109=CARTESIAN_POINT('',(-7.84276902675629,-20.,2.67326033115387));
#41110=CARTESIAN_POINT('Ctrl Pts',(-7.84276902675629,-19.5,2.67326033115387));
#41111=CARTESIAN_POINT('Ctrl Pts',(-7.84276902675629,-19.5,3.35470592975616));
#41112=CARTESIAN_POINT('Ctrl Pts',(-7.4560022354126,-19.5,3.9471343755722));
#41113=CARTESIAN_POINT('Ctrl Pts',(-7.52660259604454,-20.,1.55286467075348));
#41114=CARTESIAN_POINT('Ctrl Pts',(-7.52660259604454,-19.5,1.55286467075348));
#41115=CARTESIAN_POINT('Ctrl Pts',(-7.84276902675629,-20.,2.05320572853088));
#41116=CARTESIAN_POINT('Ctrl Pts',(-7.84276902675629,-19.5,2.05320572853088));
#41117=CARTESIAN_POINT('Ctrl Pts',(-7.84276902675629,-20.,2.67326033115387));
#41118=CARTESIAN_POINT('Ctrl Pts',(-7.84276902675629,-19.5,2.67326033115387));
#41119=CARTESIAN_POINT('',(-7.52660259604454,-19.5,1.55286467075348));
#41120=CARTESIAN_POINT('',(-7.52660259604454,-20.,1.55286467075348));
#41121=CARTESIAN_POINT('Ctrl Pts',(-7.52660259604454,-19.5,1.55286467075348));
#41122=CARTESIAN_POINT('Ctrl Pts',(-7.84276902675629,-19.5,2.05320572853088));
#41123=CARTESIAN_POINT('Ctrl Pts',(-7.84276902675629,-19.5,2.67326033115387));
#41124=CARTESIAN_POINT('Ctrl Pts',(-6.5658250451088,-20.,0.714870452880859));
#41125=CARTESIAN_POINT('Ctrl Pts',(-6.5658250451088,-19.5,0.714870452880859));
#41126=CARTESIAN_POINT('Ctrl Pts',(-7.21043616533279,-20.,1.05252361297607));
#41127=CARTESIAN_POINT('Ctrl Pts',(-7.21043616533279,-19.5,1.05252361297607));
#41128=CARTESIAN_POINT('Ctrl Pts',(-7.52660259604454,-20.,1.55286467075348));
#41129=CARTESIAN_POINT('Ctrl Pts',(-7.52660259604454,-19.5,1.55286467075348));
#41130=CARTESIAN_POINT('',(-6.5658250451088,-19.5,0.714870452880859));
#41131=CARTESIAN_POINT('',(-6.5658250451088,-20.,0.714870452880859));
#41132=CARTESIAN_POINT('Ctrl Pts',(-6.5658250451088,-19.5,0.714870452880859));
#41133=CARTESIAN_POINT('Ctrl Pts',(-7.21043616533279,-19.5,1.05252361297607));
#41134=CARTESIAN_POINT('Ctrl Pts',(-7.52660259604454,-19.5,1.55286467075348));
#41135=CARTESIAN_POINT('Ctrl Pts',(-4.82844471931458,-20.,0.15313720703125));
#41136=CARTESIAN_POINT('Ctrl Pts',(-4.82844471931458,-19.5,0.15313720703125));
#41137=CARTESIAN_POINT('Ctrl Pts',(-6.0685533285141,-20.,0.450886249542236));
#41138=CARTESIAN_POINT('Ctrl Pts',(-6.0685533285141,-19.5,0.450886249542236));
#41139=CARTESIAN_POINT('Ctrl Pts',(-6.5658250451088,-20.,0.714870452880859));
#41140=CARTESIAN_POINT('Ctrl Pts',(-6.5658250451088,-19.5,0.714870452880859));
#41141=CARTESIAN_POINT('',(-4.82844471931458,-19.5,0.15313720703125));
#41142=CARTESIAN_POINT('',(-4.82844471931458,-20.,0.15313720703125));
#41143=CARTESIAN_POINT('Ctrl Pts',(-4.82844471931458,-19.5,0.15313720703125));
#41144=CARTESIAN_POINT('Ctrl Pts',(-6.0685533285141,-19.5,0.450886249542236));
#41145=CARTESIAN_POINT('Ctrl Pts',(-6.5658250451088,-19.5,0.714870452880859));
#41146=CARTESIAN_POINT('Ctrl Pts',(-3.22612524032593,-20.,-0.28581166267395));
#41147=CARTESIAN_POINT('Ctrl Pts',(-3.22612524032593,-19.5,-0.28581166267395));
#41148=CARTESIAN_POINT('Ctrl Pts',(-3.5883355140686,-20.,-0.144611835479737));
#41149=CARTESIAN_POINT('Ctrl Pts',(-3.5883355140686,-19.5,-0.144611835479737));
#41150=CARTESIAN_POINT('Ctrl Pts',(-4.82844471931458,-20.,0.15313720703125));
#41151=CARTESIAN_POINT('Ctrl Pts',(-4.82844471931458,-19.5,0.15313720703125));
#41152=CARTESIAN_POINT('',(-3.22612524032593,-19.5,-0.28581166267395));
#41153=CARTESIAN_POINT('',(-3.22612524032593,-20.,-0.28581166267395));
#41154=CARTESIAN_POINT('Ctrl Pts',(-3.22612524032593,-19.5,-0.28581166267395));
#41155=CARTESIAN_POINT('Ctrl Pts',(-3.5883355140686,-19.5,-0.144611835479737));
#41156=CARTESIAN_POINT('Ctrl Pts',(-4.82844471931458,-19.5,0.15313720703125));
#41157=CARTESIAN_POINT('Ctrl Pts',(-2.41575658321381,-20.,-0.816848516464234));
#41158=CARTESIAN_POINT('Ctrl Pts',(-2.41575658321381,-19.5,-0.816848516464234));
#41159=CARTESIAN_POINT('Ctrl Pts',(-2.66132295131683,-20.,-0.500682830810547));
#41160=CARTESIAN_POINT('Ctrl Pts',(-2.66132295131683,-19.5,-0.500682830810547));
#41161=CARTESIAN_POINT('Ctrl Pts',(-3.22612524032593,-20.,-0.28581166267395));
#41162=CARTESIAN_POINT('Ctrl Pts',(-3.22612524032593,-19.5,-0.28581166267395));
#41163=CARTESIAN_POINT('',(-2.41575658321381,-19.5,-0.816848516464234));
#41164=CARTESIAN_POINT('',(-2.41575658321381,-20.,-0.816848516464234));
#41165=CARTESIAN_POINT('Ctrl Pts',(-2.41575658321381,-19.5,-0.816848516464234));
#41166=CARTESIAN_POINT('Ctrl Pts',(-2.66132295131683,-19.5,-0.500682830810547));
#41167=CARTESIAN_POINT('Ctrl Pts',(-3.22612524032593,-19.5,-0.28581166267395));
#41168=CARTESIAN_POINT('Ctrl Pts',(-2.17019081115723,-20.,-1.5566166639328));
#41169=CARTESIAN_POINT('Ctrl Pts',(-2.17019081115723,-19.5,-1.5566166639328));
#41170=CARTESIAN_POINT('Ctrl Pts',(-2.17019081115723,-20.,-1.13301539421082));
#41171=CARTESIAN_POINT('Ctrl Pts',(-2.17019081115723,-19.5,-1.13301539421082));
#41172=CARTESIAN_POINT('Ctrl Pts',(-2.41575658321381,-20.,-0.816848516464234));
#41173=CARTESIAN_POINT('Ctrl Pts',(-2.41575658321381,-19.5,-0.816848516464234));
#41174=CARTESIAN_POINT('',(-2.17019081115723,-19.5,-1.5566166639328));
#41175=CARTESIAN_POINT('',(-2.17019081115723,-20.,-1.5566166639328));
#41176=CARTESIAN_POINT('Ctrl Pts',(-2.17019081115723,-19.5,-1.5566166639328));
#41177=CARTESIAN_POINT('Ctrl Pts',(-2.17019081115723,-19.5,-1.13301539421082));
#41178=CARTESIAN_POINT('Ctrl Pts',(-2.41575658321381,-19.5,-0.816848516464234));
#41179=CARTESIAN_POINT('Ctrl Pts',(-2.4249655008316,-20.,-2.32708060741425));
#41180=CARTESIAN_POINT('Ctrl Pts',(-2.4249655008316,-19.5,-2.32708060741425));
#41181=CARTESIAN_POINT('Ctrl Pts',(-2.17019081115723,-20.,-1.97407925128937));
#41182=CARTESIAN_POINT('Ctrl Pts',(-2.17019081115723,-19.5,-1.97407925128937));
#41183=CARTESIAN_POINT('Ctrl Pts',(-2.17019081115723,-20.,-1.5566166639328));
#41184=CARTESIAN_POINT('Ctrl Pts',(-2.17019081115723,-19.5,-1.5566166639328));
#41185=CARTESIAN_POINT('',(-2.4249655008316,-19.5,-2.32708060741425));
#41186=CARTESIAN_POINT('',(-2.4249655008316,-20.,-2.32708060741425));
#41187=CARTESIAN_POINT('Ctrl Pts',(-2.4249655008316,-19.5,-2.32708060741425));
#41188=CARTESIAN_POINT('Ctrl Pts',(-2.17019081115723,-19.5,-1.97407925128937));
#41189=CARTESIAN_POINT('Ctrl Pts',(-2.17019081115723,-19.5,-1.5566166639328));
#41190=CARTESIAN_POINT('Ctrl Pts',(-3.20156872272491,-20.,-2.88267397880554));
#41191=CARTESIAN_POINT('Ctrl Pts',(-3.20156872272491,-19.5,-2.88267397880554));
#41192=CARTESIAN_POINT('Ctrl Pts',(-2.67974019050598,-20.,-2.68008136749268));
#41193=CARTESIAN_POINT('Ctrl Pts',(-2.67974019050598,-19.5,-2.68008136749268));
#41194=CARTESIAN_POINT('Ctrl Pts',(-2.4249655008316,-20.,-2.32708060741425));
#41195=CARTESIAN_POINT('Ctrl Pts',(-2.4249655008316,-19.5,-2.32708060741425));
#41196=CARTESIAN_POINT('',(-3.20156872272491,-19.5,-2.88267397880554));
#41197=CARTESIAN_POINT('',(-3.20156872272491,-20.,-2.88267397880554));
#41198=CARTESIAN_POINT('Ctrl Pts',(-3.20156872272491,-19.5,-2.88267397880554));
#41199=CARTESIAN_POINT('Ctrl Pts',(-2.67974019050598,-19.5,-2.68008136749268));
#41200=CARTESIAN_POINT('Ctrl Pts',(-2.4249655008316,-19.5,-2.32708060741425));
#41201=CARTESIAN_POINT('Ctrl Pts',(-4.40484285354614,-20.,-3.08526659011841));
#41202=CARTESIAN_POINT('Ctrl Pts',(-4.40484285354614,-19.5,-3.08526659011841));
#41203=CARTESIAN_POINT('Ctrl Pts',(-3.7233966588974,-20.,-3.08526659011841));
#41204=CARTESIAN_POINT('Ctrl Pts',(-3.7233966588974,-19.5,-3.08526659011841));
#41205=CARTESIAN_POINT('Ctrl Pts',(-3.20156872272491,-20.,-2.88267397880554));
#41206=CARTESIAN_POINT('Ctrl Pts',(-3.20156872272491,-19.5,-2.88267397880554));
#41207=CARTESIAN_POINT('',(-4.40484285354614,-19.5,-3.08526659011841));
#41208=CARTESIAN_POINT('',(-4.40484285354614,-20.,-3.08526659011841));
#41209=CARTESIAN_POINT('Ctrl Pts',(-4.40484285354614,-19.5,-3.08526659011841));
#41210=CARTESIAN_POINT('Ctrl Pts',(-3.7233966588974,-19.5,-3.08526659011841));
#41211=CARTESIAN_POINT('Ctrl Pts',(-3.20156872272491,-19.5,-2.88267397880554));
#41212=CARTESIAN_POINT('Ctrl Pts',(-5.78615248203278,-20.,-2.81821274757385));
#41213=CARTESIAN_POINT('Ctrl Pts',(-5.78615248203278,-19.5,-2.81821274757385));
#41214=CARTESIAN_POINT('Ctrl Pts',(-5.17223715782166,-20.,-3.08526659011841));
#41215=CARTESIAN_POINT('Ctrl Pts',(-5.17223715782166,-19.5,-3.08526659011841));
#41216=CARTESIAN_POINT('Ctrl Pts',(-4.40484285354614,-20.,-3.08526659011841));
#41217=CARTESIAN_POINT('Ctrl Pts',(-4.40484285354614,-19.5,-3.08526659011841));
#41218=CARTESIAN_POINT('',(-5.78615248203278,-19.5,-2.81821274757385));
#41219=CARTESIAN_POINT('',(-5.78615248203278,-20.,-2.81821274757385));
#41220=CARTESIAN_POINT('Ctrl Pts',(-5.78615248203278,-19.5,-2.81821274757385));
#41221=CARTESIAN_POINT('Ctrl Pts',(-5.17223715782166,-19.5,-3.08526659011841));
#41222=CARTESIAN_POINT('Ctrl Pts',(-4.40484285354614,-19.5,-3.08526659011841));
#41223=CARTESIAN_POINT('Ctrl Pts',(-6.69167771935463,-20.,-2.11834931373596));
#41224=CARTESIAN_POINT('Ctrl Pts',(-6.69167771935463,-19.5,-2.11834931373596));
#41225=CARTESIAN_POINT('Ctrl Pts',(-6.4000678062439,-20.,-2.55115950107574));
#41226=CARTESIAN_POINT('Ctrl Pts',(-6.4000678062439,-19.5,-2.55115950107574));
#41227=CARTESIAN_POINT('Ctrl Pts',(-5.78615248203278,-20.,-2.81821274757385));
#41228=CARTESIAN_POINT('Ctrl Pts',(-5.78615248203278,-19.5,-2.81821274757385));
#41229=CARTESIAN_POINT('',(-6.69167771935463,-19.5,-2.11834931373596));
#41230=CARTESIAN_POINT('',(-6.69167771935463,-20.,-2.11834931373596));
#41231=CARTESIAN_POINT('Ctrl Pts',(-6.69167771935463,-19.5,-2.11834931373596));
#41232=CARTESIAN_POINT('Ctrl Pts',(-6.4000678062439,-19.5,-2.55115950107574));
#41233=CARTESIAN_POINT('Ctrl Pts',(-5.78615248203278,-19.5,-2.81821274757385));
#41234=CARTESIAN_POINT('Ctrl Pts',(-7.06309646368027,-20.,-1.0102322101593));
#41235=CARTESIAN_POINT('Ctrl Pts',(-7.06309646368027,-19.5,-1.0102322101593));
#41236=CARTESIAN_POINT('Ctrl Pts',(-6.98328748345375,-20.,-1.68553912639618));
#41237=CARTESIAN_POINT('Ctrl Pts',(-6.98328748345375,-19.5,-1.68553912639618));
#41238=CARTESIAN_POINT('Ctrl Pts',(-6.69167771935463,-20.,-2.11834931373596));
#41239=CARTESIAN_POINT('Ctrl Pts',(-6.69167771935463,-19.5,-2.11834931373596));
#41240=CARTESIAN_POINT('',(-7.06309646368027,-19.5,-1.0102322101593));
#41241=CARTESIAN_POINT('',(-7.06309646368027,-20.,-1.0102322101593));
#41242=CARTESIAN_POINT('Ctrl Pts',(-7.06309646368027,-19.5,-1.0102322101593));
#41243=CARTESIAN_POINT('Ctrl Pts',(-6.98328748345375,-19.5,-1.68553912639618));
#41244=CARTESIAN_POINT('Ctrl Pts',(-6.69167771935463,-19.5,-2.11834931373596));
#41245=CARTESIAN_POINT('Origin',(-8.18656161427498,-20.,-1.10845828056335));
#41246=CARTESIAN_POINT('',(-8.18656161427498,-19.5,-1.10845828056335));
#41247=CARTESIAN_POINT('',(-8.18656161427498,-20.,-1.10845828056335));
#41248=CARTESIAN_POINT('',(-8.18656161427498,-19.5,-1.10845828056335));
#41249=CARTESIAN_POINT('Ctrl Pts',(-7.69235968589783,-20.,-2.72612595558167));
#41250=CARTESIAN_POINT('Ctrl Pts',(-7.69235968589783,-19.5,-2.72612595558167));
#41251=CARTESIAN_POINT('Ctrl Pts',(-8.16200498491526,-20.,-2.01091432571411));
#41252=CARTESIAN_POINT('Ctrl Pts',(-8.16200498491526,-19.5,-2.01091432571411));
#41253=CARTESIAN_POINT('Ctrl Pts',(-8.18656161427498,-20.,-1.10845828056335));
#41254=CARTESIAN_POINT('Ctrl Pts',(-8.18656161427498,-19.5,-1.10845828056335));
#41255=CARTESIAN_POINT('',(-7.69235968589783,-19.5,-2.72612595558167));
#41256=CARTESIAN_POINT('',(-7.69235968589783,-20.,-2.72612595558167));
#41257=CARTESIAN_POINT('Ctrl Pts',(-7.69235968589783,-19.5,-2.72612595558167));
#41258=CARTESIAN_POINT('Ctrl Pts',(-8.16200498491526,-19.5,-2.01091432571411));
#41259=CARTESIAN_POINT('Ctrl Pts',(-8.18656161427498,-19.5,-1.10845828056335));
#41260=CARTESIAN_POINT('Ctrl Pts',(-6.39699831604958,-20.,-3.79740738868713));
#41261=CARTESIAN_POINT('Ctrl Pts',(-6.39699831604958,-19.5,-3.79740738868713));
#41262=CARTESIAN_POINT('Ctrl Pts',(-7.2227144241333,-20.,-3.44133758544922));
#41263=CARTESIAN_POINT('Ctrl Pts',(-7.2227144241333,-19.5,-3.44133758544922));
#41264=CARTESIAN_POINT('Ctrl Pts',(-7.69235968589783,-20.,-2.72612595558167));
#41265=CARTESIAN_POINT('Ctrl Pts',(-7.69235968589783,-19.5,-2.72612595558167));
#41266=CARTESIAN_POINT('Ctrl Pts',(-6.39699831604958,-19.5,-3.79740738868713));
#41267=CARTESIAN_POINT('Ctrl Pts',(-7.2227144241333,-19.5,-3.44133758544922));
#41268=CARTESIAN_POINT('Ctrl Pts',(-7.69235968589783,-19.5,-2.72612595558167));
#41269=CARTESIAN_POINT('Origin',(-4.60436530411243,-19.5,0.49999988079071));
#41270=CARTESIAN_POINT('Origin',(3.1954300403595,-20.,-0.00341081619262718));
#41271=CARTESIAN_POINT('',(3.1954300403595,-19.5,-0.00341081619262718));
#41272=CARTESIAN_POINT('',(3.1954300403595,-20.,-0.00341081619262718));
#41273=CARTESIAN_POINT('',(1.81412041187287,-19.5,-0.00341081619262718));
#41274=CARTESIAN_POINT('',(3.1954300403595,-19.5,-0.00341081619262718));
#41275=CARTESIAN_POINT('',(1.81412041187287,-20.,-0.00341081619262718));
#41276=CARTESIAN_POINT('Ctrl Pts',(3.85845869779587,-20.,-0.0463845729827883));
#41277=CARTESIAN_POINT('Ctrl Pts',(3.85845869779587,-19.5,-0.0463845729827883));
#41278=CARTESIAN_POINT('Ctrl Pts',(3.65586668252945,-20.,-0.00341081619262718));
#41279=CARTESIAN_POINT('Ctrl Pts',(3.65586668252945,-19.5,-0.00341081619262718));
#41280=CARTESIAN_POINT('Ctrl Pts',(3.1954300403595,-20.,-0.00341081619262718));
#41281=CARTESIAN_POINT('Ctrl Pts',(3.1954300403595,-19.5,-0.00341081619262718));
#41282=CARTESIAN_POINT('',(3.85845869779587,-19.5,-0.0463845729827883));
#41283=CARTESIAN_POINT('',(3.85845869779587,-20.,-0.0463845729827883));
#41284=CARTESIAN_POINT('Ctrl Pts',(3.85845869779587,-19.5,-0.0463845729827883));
#41285=CARTESIAN_POINT('Ctrl Pts',(3.65586668252945,-19.5,-0.00341081619262718));
#41286=CARTESIAN_POINT('Ctrl Pts',(3.1954300403595,-19.5,-0.00341081619262718));
#41287=CARTESIAN_POINT('Ctrl Pts',(4.40177381038666,-20.,-0.28581166267395));
#41288=CARTESIAN_POINT('Ctrl Pts',(4.40177381038666,-19.5,-0.28581166267395));
#41289=CARTESIAN_POINT('Ctrl Pts',(4.13472056388855,-20.,-0.11391544342041));
#41290=CARTESIAN_POINT('Ctrl Pts',(4.13472056388855,-19.5,-0.11391544342041));
#41291=CARTESIAN_POINT('Ctrl Pts',(3.85845869779587,-20.,-0.0463845729827883));
#41292=CARTESIAN_POINT('Ctrl Pts',(3.85845869779587,-19.5,-0.0463845729827883));
#41293=CARTESIAN_POINT('',(4.40177381038666,-19.5,-0.28581166267395));
#41294=CARTESIAN_POINT('',(4.40177381038666,-20.,-0.28581166267395));
#41295=CARTESIAN_POINT('Ctrl Pts',(4.40177381038666,-19.5,-0.28581166267395));
#41296=CARTESIAN_POINT('Ctrl Pts',(4.13472056388855,-19.5,-0.11391544342041));
#41297=CARTESIAN_POINT('Ctrl Pts',(3.85845869779587,-19.5,-0.0463845729827883));
#41298=CARTESIAN_POINT('Ctrl Pts',(5.00648021697998,-20.,-0.887449026107788));
#41299=CARTESIAN_POINT('Ctrl Pts',(5.00648021697998,-19.5,-0.887449026107788));
#41300=CARTESIAN_POINT('Ctrl Pts',(4.66882705688477,-20.,-0.45770788192749));
#41301=CARTESIAN_POINT('Ctrl Pts',(4.66882705688477,-19.5,-0.45770788192749));
#41302=CARTESIAN_POINT('Ctrl Pts',(4.40177381038666,-20.,-0.28581166267395));
#41303=CARTESIAN_POINT('Ctrl Pts',(4.40177381038666,-19.5,-0.28581166267395));
#41304=CARTESIAN_POINT('',(5.00648021697998,-19.5,-0.887449026107788));
#41305=CARTESIAN_POINT('',(5.00648021697998,-20.,-0.887449026107788));
#41306=CARTESIAN_POINT('Ctrl Pts',(5.00648021697998,-19.5,-0.887449026107788));
#41307=CARTESIAN_POINT('Ctrl Pts',(4.66882705688477,-19.5,-0.45770788192749));
#41308=CARTESIAN_POINT('Ctrl Pts',(4.40177381038666,-19.5,-0.28581166267395));
#41309=CARTESIAN_POINT('Ctrl Pts',(5.86596190929413,-20.,-2.12755823135376));
#41310=CARTESIAN_POINT('Ctrl Pts',(5.86596190929413,-19.5,-2.12755823135376));
#41311=CARTESIAN_POINT('Ctrl Pts',(5.34413397312165,-20.,-1.31719017028809));
#41312=CARTESIAN_POINT('Ctrl Pts',(5.34413397312165,-19.5,-1.31719017028809));
#41313=CARTESIAN_POINT('Ctrl Pts',(5.00648021697998,-20.,-0.887449026107788));
#41314=CARTESIAN_POINT('Ctrl Pts',(5.00648021697998,-19.5,-0.887449026107788));
#41315=CARTESIAN_POINT('',(5.86596190929413,-19.5,-2.12755823135376));
#41316=CARTESIAN_POINT('',(5.86596190929413,-20.,-2.12755823135376));
#41317=CARTESIAN_POINT('Ctrl Pts',(5.86596190929413,-19.5,-2.12755823135376));
#41318=CARTESIAN_POINT('Ctrl Pts',(5.34413397312165,-19.5,-1.31719017028809));
#41319=CARTESIAN_POINT('Ctrl Pts',(5.00648021697998,-19.5,-0.887449026107788));
#41320=CARTESIAN_POINT('Origin',(7.05695748329163,-20.,-4.));
#41321=CARTESIAN_POINT('',(7.05695748329163,-19.5,-4.));
#41322=CARTESIAN_POINT('Origin',(6.98942661285401,-20.,-1.55047798156738));
#41323=CARTESIAN_POINT('',(6.98942661285401,-19.5,-1.55047798156738));
#41324=CARTESIAN_POINT('',(6.98942661285401,-20.,-1.55047798156738));
#41325=CARTESIAN_POINT('',(6.98942661285401,-19.5,-1.55047798156738));
#41326=CARTESIAN_POINT('Ctrl Pts',(6.00102305412293,-20.,-0.353342533111572));
#41327=CARTESIAN_POINT('Ctrl Pts',(6.00102305412293,-19.5,-0.353342533111572));
#41328=CARTESIAN_POINT('Ctrl Pts',(6.52285099029541,-20.,-0.832196712493897));
#41329=CARTESIAN_POINT('Ctrl Pts',(6.52285099029541,-19.5,-0.832196712493897));
#41330=CARTESIAN_POINT('Ctrl Pts',(6.98942661285401,-20.,-1.55047798156738));
#41331=CARTESIAN_POINT('Ctrl Pts',(6.98942661285401,-19.5,-1.55047798156738));
#41332=CARTESIAN_POINT('',(6.00102305412293,-19.5,-0.353342533111572));
#41333=CARTESIAN_POINT('',(6.00102305412293,-20.,-0.353342533111572));
#41334=CARTESIAN_POINT('Ctrl Pts',(6.00102305412293,-19.5,-0.353342533111572));
#41335=CARTESIAN_POINT('Ctrl Pts',(6.52285099029541,-19.5,-0.832196712493897));
#41336=CARTESIAN_POINT('Ctrl Pts',(6.98942661285401,-19.5,-1.55047798156738));
#41337=CARTESIAN_POINT('Ctrl Pts',(5.28274238109589,-20.,0.0948152542114256));
#41338=CARTESIAN_POINT('Ctrl Pts',(5.28274238109589,-19.5,0.0948152542114256));
#41339=CARTESIAN_POINT('Ctrl Pts',(5.7554566860199,-20.,-0.132333278656006));
#41340=CARTESIAN_POINT('Ctrl Pts',(5.7554566860199,-19.5,-0.132333278656006));
#41341=CARTESIAN_POINT('Ctrl Pts',(6.00102305412293,-20.,-0.353342533111572));
#41342=CARTESIAN_POINT('Ctrl Pts',(6.00102305412293,-19.5,-0.353342533111572));
#41343=CARTESIAN_POINT('',(5.28274238109589,-19.5,0.0948152542114256));
#41344=CARTESIAN_POINT('',(5.28274238109589,-20.,0.0948152542114256));
#41345=CARTESIAN_POINT('Ctrl Pts',(5.28274238109589,-19.5,0.0948152542114256));
#41346=CARTESIAN_POINT('Ctrl Pts',(5.7554566860199,-19.5,-0.132333278656006));
#41347=CARTESIAN_POINT('Ctrl Pts',(6.00102305412293,-19.5,-0.353342533111572));
#41348=CARTESIAN_POINT('Ctrl Pts',(7.19815790653229,-20.,0.92974042892456));
#41349=CARTESIAN_POINT('Ctrl Pts',(7.19815790653229,-19.5,0.92974042892456));
#41350=CARTESIAN_POINT('Ctrl Pts',(6.57810330390931,-20.,0.272850751876831));
#41351=CARTESIAN_POINT('Ctrl Pts',(6.57810330390931,-19.5,0.272850751876831));
#41352=CARTESIAN_POINT('Ctrl Pts',(5.28274238109589,-20.,0.0948152542114256));
#41353=CARTESIAN_POINT('Ctrl Pts',(5.28274238109589,-19.5,0.0948152542114256));
#41354=CARTESIAN_POINT('',(7.19815790653229,-19.5,0.92974042892456));
#41355=CARTESIAN_POINT('',(7.19815790653229,-20.,0.92974042892456));
#41356=CARTESIAN_POINT('Ctrl Pts',(7.19815790653229,-19.5,0.92974042892456));
#41357=CARTESIAN_POINT('Ctrl Pts',(6.57810330390931,-19.5,0.272850751876831));
#41358=CARTESIAN_POINT('Ctrl Pts',(5.28274238109589,-19.5,0.0948152542114256));
#41359=CARTESIAN_POINT('Ctrl Pts',(7.81821250915528,-20.,2.54433786869049));
#41360=CARTESIAN_POINT('Ctrl Pts',(7.81821250915528,-19.5,2.54433786869049));
#41361=CARTESIAN_POINT('Ctrl Pts',(7.81821250915528,-20.,1.58663010597229));
#41362=CARTESIAN_POINT('Ctrl Pts',(7.81821250915528,-19.5,1.58663010597229));
#41363=CARTESIAN_POINT('Ctrl Pts',(7.19815790653229,-20.,0.92974042892456));
#41364=CARTESIAN_POINT('Ctrl Pts',(7.19815790653229,-19.5,0.92974042892456));
#41365=CARTESIAN_POINT('',(7.81821250915528,-19.5,2.54433786869049));
#41366=CARTESIAN_POINT('',(7.81821250915528,-20.,2.54433786869049));
#41367=CARTESIAN_POINT('Ctrl Pts',(7.81821250915528,-19.5,2.54433786869049));
#41368=CARTESIAN_POINT('Ctrl Pts',(7.81821250915528,-19.5,1.58663010597229));
#41369=CARTESIAN_POINT('Ctrl Pts',(7.19815790653229,-19.5,0.92974042892456));
#41370=CARTESIAN_POINT('Ctrl Pts',(7.44372427463532,-20.,3.90109097957611));
#41371=CARTESIAN_POINT('Ctrl Pts',(7.44372427463532,-19.5,3.90109097957611));
#41372=CARTESIAN_POINT('Ctrl Pts',(7.81821250915528,-20.,3.28717565536499));
#41373=CARTESIAN_POINT('Ctrl Pts',(7.81821250915528,-19.5,3.28717565536499));
#41374=CARTESIAN_POINT('Ctrl Pts',(7.81821250915528,-20.,2.54433786869049));
#41375=CARTESIAN_POINT('Ctrl Pts',(7.81821250915528,-19.5,2.54433786869049));
#41376=CARTESIAN_POINT('',(7.44372427463532,-19.5,3.90109097957611));
#41377=CARTESIAN_POINT('',(7.44372427463532,-20.,3.90109097957611));
#41378=CARTESIAN_POINT('Ctrl Pts',(7.44372427463532,-19.5,3.90109097957611));
#41379=CARTESIAN_POINT('Ctrl Pts',(7.81821250915528,-19.5,3.28717565536499));
#41380=CARTESIAN_POINT('Ctrl Pts',(7.81821250915528,-19.5,2.54433786869049));
#41381=CARTESIAN_POINT('Ctrl Pts',(6.44304215908051,-20.,4.75750303268433));
#41382=CARTESIAN_POINT('Ctrl Pts',(6.44304215908051,-19.5,4.75750303268433));
#41383=CARTESIAN_POINT('Ctrl Pts',(7.06923604011536,-20.,4.51500630378723));
#41384=CARTESIAN_POINT('Ctrl Pts',(7.06923604011536,-19.5,4.51500630378723));
#41385=CARTESIAN_POINT('Ctrl Pts',(7.44372427463532,-20.,3.90109097957611));
#41386=CARTESIAN_POINT('Ctrl Pts',(7.44372427463532,-19.5,3.90109097957611));
#41387=CARTESIAN_POINT('',(6.44304215908051,-19.5,4.75750303268433));
#41388=CARTESIAN_POINT('',(6.44304215908051,-20.,4.75750303268433));
#41389=CARTESIAN_POINT('Ctrl Pts',(6.44304215908051,-19.5,4.75750303268433));
#41390=CARTESIAN_POINT('Ctrl Pts',(7.06923604011536,-19.5,4.51500630378723));
#41391=CARTESIAN_POINT('Ctrl Pts',(7.44372427463532,-19.5,3.90109097957611));
#41392=CARTESIAN_POINT('Ctrl Pts',(4.61357444524765,-20.,4.99999976158142));
#41393=CARTESIAN_POINT('Ctrl Pts',(4.61357444524765,-19.5,4.99999976158142));
#41394=CARTESIAN_POINT('Ctrl Pts',(5.81684827804566,-20.,4.99999976158142));
#41395=CARTESIAN_POINT('Ctrl Pts',(5.81684827804566,-19.5,4.99999976158142));
#41396=CARTESIAN_POINT('Ctrl Pts',(6.44304215908051,-20.,4.75750303268433));
#41397=CARTESIAN_POINT('Ctrl Pts',(6.44304215908051,-19.5,4.75750303268433));
#41398=CARTESIAN_POINT('',(4.61357444524765,-19.5,4.99999976158142));
#41399=CARTESIAN_POINT('',(4.61357444524765,-20.,4.99999976158142));
#41400=CARTESIAN_POINT('Ctrl Pts',(4.61357444524765,-19.5,4.99999976158142));
#41401=CARTESIAN_POINT('Ctrl Pts',(5.81684827804566,-19.5,4.99999976158142));
#41402=CARTESIAN_POINT('Ctrl Pts',(6.44304215908051,-19.5,4.75750303268433));
#41403=CARTESIAN_POINT('Origin',(0.623124465346341,-20.,4.99999976158142));
#41404=CARTESIAN_POINT('',(0.623124465346341,-19.5,4.99999976158142));
#41405=CARTESIAN_POINT('Origin',(1.81412041187287,-20.,-4.));
#41406=CARTESIAN_POINT('',(1.81412041187287,-19.5,-4.));
#41407=CARTESIAN_POINT('',(1.81412041187287,-20.,-4.));
#41408=CARTESIAN_POINT('',(1.81412041187287,-19.5,-4.));
#41409=CARTESIAN_POINT('Origin',(1.81412041187287,-20.,-0.00341081619262718));
#41410=CARTESIAN_POINT('',(1.81412041187287,-19.5,-0.00341081619262718));
#41411=CARTESIAN_POINT('Origin',(4.58901774138213,-19.5,0.49999988079071));
#41412=CARTESIAN_POINT('Origin',(25.4253059625626,-20.,4.99999976158142));
#41413=CARTESIAN_POINT('',(25.4253059625626,-19.5,4.99999976158142));
#41414=CARTESIAN_POINT('',(25.4253059625626,-20.,4.99999976158142));
#41415=CARTESIAN_POINT('',(21.833900809288,-19.5,-0.187585592269898));
#41416=CARTESIAN_POINT('',(25.4253059625626,-19.5,4.99999976158142));
#41417=CARTESIAN_POINT('',(21.833900809288,-20.,-0.187585592269898));
#41418=CARTESIAN_POINT('Origin',(24.0378570556641,-20.,4.99999976158142));
#41419=CARTESIAN_POINT('',(24.0378570556641,-19.5,4.99999976158142));
#41420=CARTESIAN_POINT('',(24.0378570556641,-20.,4.99999976158142));
#41421=CARTESIAN_POINT('',(24.0378570556641,-19.5,4.99999976158142));
#41422=CARTESIAN_POINT('Origin',(22.2943377494812,-20.,2.3540244102478));
#41423=CARTESIAN_POINT('',(22.2943377494812,-19.5,2.3540244102478));
#41424=CARTESIAN_POINT('',(22.2943377494812,-20.,2.3540244102478));
#41425=CARTESIAN_POINT('',(22.2943377494812,-19.5,2.3540244102478));
#41426=CARTESIAN_POINT('Ctrl Pts',(21.3120725750923,-20.,0.763983488082886));
#41427=CARTESIAN_POINT('Ctrl Pts',(21.3120725750923,-19.5,0.763983488082886));
#41428=CARTESIAN_POINT('Ctrl Pts',(21.7172569036484,-20.,1.46998620033264));
#41429=CARTESIAN_POINT('Ctrl Pts',(21.7172569036484,-19.5,1.46998620033264));
#41430=CARTESIAN_POINT('Ctrl Pts',(22.2943377494812,-20.,2.3540244102478));
#41431=CARTESIAN_POINT('Ctrl Pts',(22.2943377494812,-19.5,2.3540244102478));
#41432=CARTESIAN_POINT('',(21.3120725750923,-19.5,0.763983488082886));
#41433=CARTESIAN_POINT('',(21.3120725750923,-20.,0.763983488082886));
#41434=CARTESIAN_POINT('Ctrl Pts',(21.3120725750923,-19.5,0.763983488082886));
#41435=CARTESIAN_POINT('Ctrl Pts',(21.7172569036484,-19.5,1.46998620033264));
#41436=CARTESIAN_POINT('Ctrl Pts',(22.2943377494812,-19.5,2.3540244102478));
#41437=CARTESIAN_POINT('Ctrl Pts',(20.3973388671875,-20.,2.28649353981018));
#41438=CARTESIAN_POINT('Ctrl Pts',(20.3973388671875,-19.5,2.28649353981018));
#41439=CARTESIAN_POINT('Ctrl Pts',(20.8884710073471,-20.,1.52523851394653));
#41440=CARTESIAN_POINT('Ctrl Pts',(20.8884710073471,-19.5,1.52523851394653));
#41441=CARTESIAN_POINT('Ctrl Pts',(21.3120725750923,-20.,0.763983488082886));
#41442=CARTESIAN_POINT('Ctrl Pts',(21.3120725750923,-19.5,0.763983488082886));
#41443=CARTESIAN_POINT('',(20.3973388671875,-19.5,2.28649353981018));
#41444=CARTESIAN_POINT('',(20.3973388671875,-20.,2.28649353981018));
#41445=CARTESIAN_POINT('Ctrl Pts',(20.3973388671875,-19.5,2.28649353981018));
#41446=CARTESIAN_POINT('Ctrl Pts',(20.8884710073471,-19.5,1.52523851394653));
#41447=CARTESIAN_POINT('Ctrl Pts',(21.3120725750923,-19.5,0.763983488082886));
#41448=CARTESIAN_POINT('Origin',(18.6231234669685,-20.,4.99999976158142));
#41449=CARTESIAN_POINT('',(18.6231234669685,-19.5,4.99999976158142));
#41450=CARTESIAN_POINT('',(18.6231234669685,-20.,4.99999976158142));
#41451=CARTESIAN_POINT('',(18.6231234669685,-19.5,4.99999976158142));
#41452=CARTESIAN_POINT('Origin',(17.1742831147276,-20.,4.99999976158142));
#41453=CARTESIAN_POINT('',(17.1742831147276,-19.5,4.99999976158142));
#41454=CARTESIAN_POINT('',(17.1742831147276,-20.,4.99999976158142));
#41455=CARTESIAN_POINT('',(17.1742831147276,-19.5,4.99999976158142));
#41456=CARTESIAN_POINT('Origin',(20.6429049372673,-20.,-0.187585592269898));
#41457=CARTESIAN_POINT('',(20.6429049372673,-19.5,-0.187585592269898));
#41458=CARTESIAN_POINT('',(20.6429049372673,-20.,-0.187585592269898));
#41459=CARTESIAN_POINT('',(20.6429049372673,-19.5,-0.187585592269898));
#41460=CARTESIAN_POINT('Origin',(20.6429049372673,-20.,-4.));
#41461=CARTESIAN_POINT('',(20.6429049372673,-19.5,-4.));
#41462=CARTESIAN_POINT('',(20.6429049372673,-20.,-4.));
#41463=CARTESIAN_POINT('',(20.6429049372673,-19.5,-4.));
#41464=CARTESIAN_POINT('Origin',(21.833900809288,-20.,-4.));
#41465=CARTESIAN_POINT('',(21.833900809288,-19.5,-4.));
#41466=CARTESIAN_POINT('',(21.833900809288,-20.,-4.));
#41467=CARTESIAN_POINT('',(21.833900809288,-19.5,-4.));
#41468=CARTESIAN_POINT('Origin',(21.833900809288,-20.,-0.187585592269898));
#41469=CARTESIAN_POINT('',(21.833900809288,-19.5,-0.187585592269898));
#41470=CARTESIAN_POINT('Origin',(21.2997945386451,-19.5,0.49999988079071));
#41471=CARTESIAN_POINT('Origin',(-75.7581216659255,-14.1,31.3800414539374));
#41472=CARTESIAN_POINT('',(-81.2581216659255,-14.1,31.3800414539374));
#41473=CARTESIAN_POINT('Origin',(31.3800414539374,-14.1,75.7581216659255));
#41474=CARTESIAN_POINT('',(25.8800414539374,-14.1,75.7581216659255));
#41475=CARTESIAN_POINT('Origin',(-31.3800414539374,-14.1,75.7581216659255));
#41476=CARTESIAN_POINT('',(-36.8800414539374,-14.1,75.7581216659255));
#41477=CARTESIAN_POINT('Origin',(75.7581216659255,-14.1,31.3800414539374));
#41478=CARTESIAN_POINT('',(70.2581216659255,-14.1,31.3800414539374));
#41479=CARTESIAN_POINT('Origin',(0.,-3.05,75.05));
#41480=CARTESIAN_POINT('Origin',(-2.22044604925031E-15,-5.,-1.11022302462516E-15));
#41481=CARTESIAN_POINT('',(28.5,-9.,49.363448015713));
#41482=CARTESIAN_POINT('',(28.5,-5.,49.363448015713));
#41483=CARTESIAN_POINT('',(-28.5,-9.,49.363448015713));
#41484=CARTESIAN_POINT('Origin',(-2.22044604925031E-15,-9.,-1.11022302462516E-15));
#41485=CARTESIAN_POINT('',(-28.5,-5.,49.363448015713));
#41486=CARTESIAN_POINT('Origin',(35.1,-5.,60.7949833456676));
#41487=CARTESIAN_POINT('',(35.1,-9.,60.7949833456676));
#41488=CARTESIAN_POINT('Origin',(-28.5,-5.,49.363448015713));
#41489=CARTESIAN_POINT('',(-35.1,-9.,60.7949833456676));
#41490=CARTESIAN_POINT('Origin',(1.77635683940025E-14,-9.,-4.70250832716619));
#41491=CARTESIAN_POINT('Origin',(-50.,-14.,5.00000000000001));
#55696=UNCERTAINTY_MEASURE_WITH_UNIT(LENGTH_MEASURE(0.01),#55738,
'DISTANCE_ACCURACY_VALUE',
'Maximum model space distance between geometric entities at asserted c
onnectivities');
#55715=UNCERTAINTY_MEASURE_WITH_UNIT(LENGTH_MEASURE(0.01),#55738,
'DISTANCE_ACCURACY_VALUE',
'Maximum model space distance between geometric entities at asserted c
onnectivities');
#55718=(
GEOMETRIC_REPRESENTATION_CONTEXT(3)
GLOBAL_UNCERTAINTY_ASSIGNED_CONTEXT((#55696))
GLOBAL_UNIT_ASSIGNED_CONTEXT((#55738,#55740,#55741))
REPRESENTATION_CONTEXT('','3D')
);
#55737=(
GEOMETRIC_REPRESENTATION_CONTEXT(3)
GLOBAL_UNCERTAINTY_ASSIGNED_CONTEXT((#55715))
GLOBAL_UNIT_ASSIGNED_CONTEXT((#55738,#55740,#55741))
REPRESENTATION_CONTEXT('','3D')
);
#55738=(
LENGTH_UNIT()
NAMED_UNIT(*)
SI_UNIT(.MILLI.,.METRE.)
);
#55740=(
NAMED_UNIT(*)
PLANE_ANGLE_UNIT()
SI_UNIT($,.RADIAN.)
);
#55741=(
NAMED_UNIT(*)
SI_UNIT($,.STERADIAN.)
SOLID_ANGLE_UNIT()
);
#55744=SHAPE_DEFINITION_REPRESENTATION(#55765,#55822);
#55765=PRODUCT_DEFINITION_SHAPE('',$,#55844);
#55822=SHAPE_REPRESENTATION('',(#27785),#55718);
#55841=PRODUCT_DEFINITION_CONTEXT('part definition',#55906,'design');
#55844=PRODUCT_DEFINITION('2026-10-26-00-33-58-284','02_Casing_Cover',#55865,
#55841);
#55865=PRODUCT_DEFINITION_FORMATION('',$,#55910);
#55906=APPLICATION_CONTEXT(
'Core Data for Automotive Mechanical Design Process');
#55907=PRODUCT_CONTEXT('part definition',#55906,'mechanical');
#55910=PRODUCT('2026-10-26-00-33-58-284','02_Casing_Cover',$,(#55907));
#55971=COLOUR_RGB('Light Blue',0.38,0.62,0.78);
#55972=FILL_AREA_STYLE_COLOUR('',#55971);
#55973=FILL_AREA_STYLE('',(#55972));
#55974=SURFACE_STYLE_FILL_AREA(#55973);
#55975=SURFACE_SIDE_STYLE('',(#55974));
#55976=SURFACE_STYLE_USAGE(.BOTH.,#55975);
#55977=PRESENTATION_STYLE_ASSIGNMENT((#55976));
ENDSEC;
END-ISO-10303-21;
